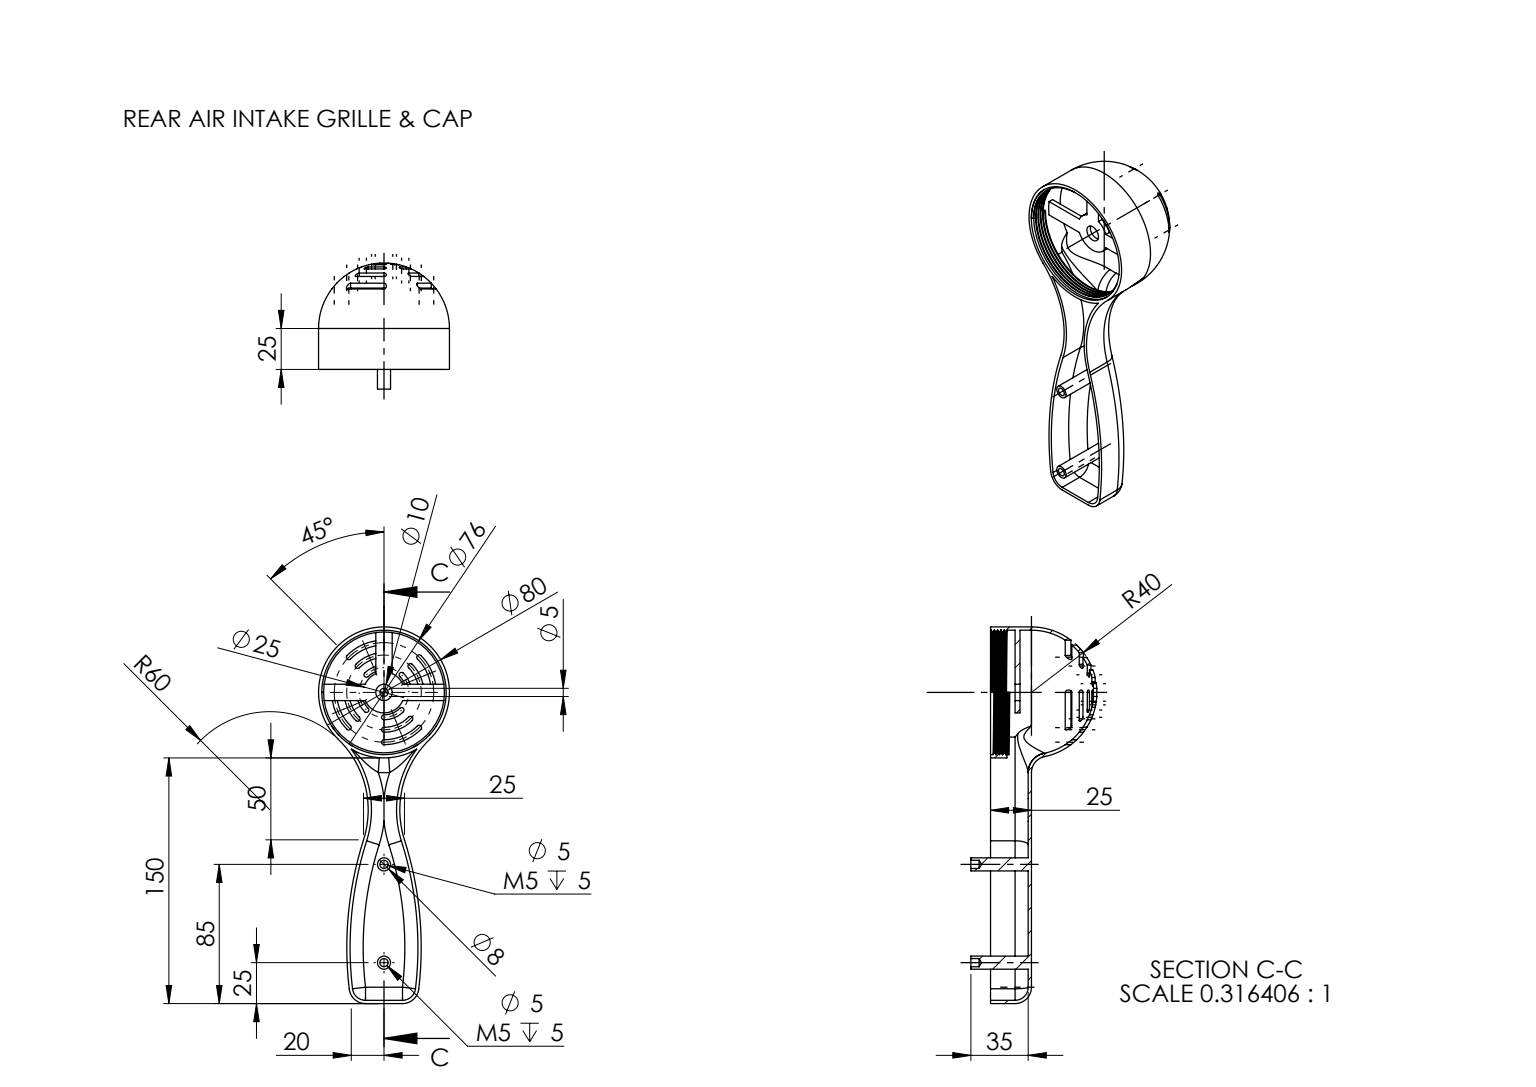
ISO-10303-21;
HEADER;
FILE_DESCRIPTION (('STEP AP214'),
    '1' );
FILE_NAME ('Rear Air Intake Grille & Cap.step',
    '2026-10-04T13:31:42',
    ( '' ),
    ( '' ),
    'SwSTEP 2.0',
    'SolidWorks 2026',
    '' );
FILE_SCHEMA (( 'AUTOMOTIVE_DESIGN' ));
ENDSEC;

DATA;
#20=CARTESIAN_POINT ( 'NONE',  ( 0.000000000000000000, 0.000000000000000000, -45.64921306006598201 ) ) ;
#25=CARTESIAN_POINT ( 'NONE',  ( -3.573655867282028392E-15, 2.428612866367529932E-14, -24.99999999999997868 ) ) ;
#63=ORIENTED_EDGE ( 'NONE', *, *, #98272, .F. ) ;
#65=CIRCLE ( 'NONE', #138924, 4.000000000000000888 ) ;
#97=CARTESIAN_POINT ( 'NONE',  ( 7.656827144875921753, -71.74905178543389184, -15.00000000000000178 ) ) ;
#127=FACE_OUTER_BOUND ( 'NONE', #92552, .T. ) ;
#189=ORIENTED_EDGE ( 'NONE', *, *, #119223, .F. ) ;
#212=SPHERICAL_SURFACE ( 'NONE', #37950, 10.00000000000000000 ) ;
#223=CARTESIAN_POINT ( 'NONE',  ( 15.64208950468054127, -40.81369178264755959, -21.33727593494802122 ) ) ;
#225=CYLINDRICAL_SURFACE ( 'NONE', #105054, 10.00000000000000178 ) ;
#232=CARTESIAN_POINT ( 'NONE',  ( 17.25602135761909395, -17.10936820804715808, -56.77278709839602300 ) ) ;
#243=VERTEX_POINT ( 'NONE', #159375 ) ;
#246=CARTESIAN_POINT ( 'NONE',  ( -30.74264578624800492, -22.33583958711396278, -7.800000000000000711 ) ) ;
#272=CARTESIAN_POINT ( 'NONE',  ( 14.16830335033699662, -40.16376294013230819, -20.11902964094307933 ) ) ;
#277=EDGE_LOOP ( 'NONE', ( #133276, #198078, #94972, #136074, #147190 ) ) ;
#299=CARTESIAN_POINT ( 'NONE',  ( 33.78191506369888941, -21.41920200728860380, -24.99999999999997868 ) ) ;
#420=ORIENTED_EDGE ( 'NONE', *, *, #46651, .T. ) ;
#424=ORIENTED_EDGE ( 'NONE', *, *, #57992, .F. ) ;
#435=CARTESIAN_POINT ( 'NONE',  ( -8.139631411200216604, -37.86970803905148131, -24.01681473740524808 ) ) ;
#457=CARTESIAN_POINT ( 'NONE',  ( 22.90195793322444473, -20.95683088396668481, -46.91699765554876222 ) ) ;
#468=EDGE_CURVE ( 'NONE', #150285, #194492, #147057, .T. ) ;
#495=CARTESIAN_POINT ( 'NONE',  ( 5.136056113497502906, -40.38396894446272967, -25.53196577693411840 ) ) ;
#515=VERTEX_POINT ( 'NONE', #119633 ) ;
#540=DIRECTION ( 'NONE',  ( 1.000000000000000000, 0.000000000000000000, 0.000000000000000000 ) ) ;
#584=AXIS2_PLACEMENT_3D ( 'NONE', #105275, #147807, #196325 ) ;
#611=ORIENTED_EDGE ( 'NONE', *, *, #28066, .F. ) ;
#630=EDGE_CURVE ( 'NONE', #182346, #12418, #12467, .T. ) ;
#707=CARTESIAN_POINT ( 'NONE',  ( -1.429200727443362906, -15.66521691804238436, -59.59145728475412795 ) ) ;
#713=CARTESIAN_POINT ( 'NONE',  ( 0.9827870232946694928, 21.65019873939048267, -58.62068706038626686 ) ) ;
#720=EDGE_LOOP ( 'NONE', ( #54967, #73852, #188508, #135992 ) ) ;
#722=ADVANCED_FACE ( 'NONE', ( #57962 ), #165143, .F. ) ;
#729=CARTESIAN_POINT ( 'NONE',  ( 37.99999999999999289, 2.893978650043524126E-14, -10.74999999453762811 ) ) ;
#742=CARTESIAN_POINT ( 'NONE',  ( 3.915344532211609163, 5.773958127068983259, -62.35465819465156301 ) ) ;
#749=EDGE_CURVE ( 'NONE', #58211, #154964, #98211, .T. ) ;
#778=CARTESIAN_POINT ( 'NONE',  ( -11.40812507854754720, -35.11059874428192273, -8.724999997268813701 ) ) ;
#782=ORIENTED_EDGE ( 'NONE', *, *, #187478, .F. ) ;
#789=CARTESIAN_POINT ( 'NONE',  ( -11.74323870453920549, 9.621741624713935792, -62.00714677346291381 ) ) ;
#803=CARTESIAN_POINT ( 'NONE',  ( -33.52048507002410105, -21.84028095222511823, -24.62089730557312350 ) ) ;
#834=ORIENTED_EDGE ( 'NONE', *, *, #188269, .F. ) ;
#928=CARTESIAN_POINT ( 'NONE',  ( -22.90350128981420141, 22.02608267474392179, -45.83983912514964487 ) ) ;
#930=CARTESIAN_POINT ( 'NONE',  ( 6.685465210013314952, -6.128229644718811819, -61.90241664256964782 ) ) ;
#962=EDGE_LOOP ( 'NONE', ( #189631, #4030 ) ) ;
#966=CARTESIAN_POINT ( 'NONE',  ( -8.724588103088155577, 0.9974278668898441946, -61.97156292062780381 ) ) ;
#981=EDGE_CURVE ( 'NONE', #31363, #49313, #26634, .T. ) ;
#1026=CARTESIAN_POINT ( 'NONE',  ( -10.65638358537376007, -44.90791467878717924, -23.56120423312990297 ) ) ;
#1031=DIRECTION ( 'NONE',  ( 0.000000000000000000, 0.000000000000000000, 1.000000000000000000 ) ) ;
#1065=CARTESIAN_POINT ( 'NONE',  ( -0.4881926659581863892, -9.021779378622676759, -61.91041879129567604 ) ) ;
#1092=CARTESIAN_POINT ( 'NONE',  ( 0.000000000000000000, 0.000000000000000000, -64.92279855667830191 ) ) ;
#1129=DIRECTION ( 'NONE',  ( -0.000000000000000000, 0.000000000000000000, 1.000000000000000000 ) ) ;
#1179=ORIENTED_EDGE ( 'NONE', *, *, #88509, .T. ) ;
#1181=DIRECTION ( 'NONE',  ( -0.000000000000000000, -0.000000000000000000, 1.000000000000000000 ) ) ;
#1190=EDGE_CURVE ( 'NONE', #113441, #194207, #182299, .T. ) ;
#1215=CARTESIAN_POINT ( 'NONE',  ( 26.46959431505284499, -27.26463967846488146, -15.00000000000000178 ) ) ;
#1217=CARTESIAN_POINT ( 'NONE',  ( -1.227931366032057224E-14, -24.30000000000003268, -54.21489346206828230 ) ) ;
#1222=CARTESIAN_POINT ( 'NONE',  ( 17.61359324038537721, -16.30702395557608142, -56.99769869564799052 ) ) ;
#1227=CARTESIAN_POINT ( 'NONE',  ( -17.26089242801066348, 17.10449713765558499, -56.77278709839601589 ) ) ;
#1233=VERTEX_POINT ( 'NONE', #44770 ) ;
#1262=CARTESIAN_POINT ( 'NONE',  ( 17.93416671128860784, -36.08982269496112139, -18.53391066944393728 ) ) ;
#1266=ORIENTED_EDGE ( 'NONE', *, *, #147318, .T. ) ;
#1280=VECTOR ( 'NONE', #85682, 1000.000000000000000 ) ;
#1289=ORIENTED_EDGE ( 'NONE', *, *, #38432, .T. ) ;
#1351=LINE ( 'NONE', #17535, #30677 ) ;
#1378=CARTESIAN_POINT ( 'NONE',  ( -20.01995586163601715, -21.79717389941245287, -51.90954606063881016 ) ) ;
#1419=ORIENTED_EDGE ( 'NONE', *, *, #80402, .F. ) ;
#1430=EDGE_CURVE ( 'NONE', #122419, #49313, #11102, .T. ) ;
#1432=CARTESIAN_POINT ( 'NONE',  ( -17.48462780208382128, -33.70920939566911301, -26.63509803227388062 ) ) ;
#1450=CARTESIAN_POINT ( 'NONE',  ( 17.62203461105333702, -16.12203461105326951, -57.08650645001478097 ) ) ;
#1454=CARTESIAN_POINT ( 'NONE',  ( 22.14710224105762748, -20.13854895287483515, -48.40914604263300447 ) ) ;
#1462=CARTESIAN_POINT ( 'NONE',  ( 6.685389299484707948, -6.128353407782586082, -63.95879637121625194 ) ) ;
#1481=CARTESIAN_POINT ( 'NONE',  ( 11.40812507854754365, 35.11059874428196537, -1.224999997268813479 ) ) ;
#1491=CARTESIAN_POINT ( 'NONE',  ( 21.53686564358446631, -33.52628202222955167, -20.57266355564622629 ) ) ;
#1611=VERTEX_POINT ( 'NONE', #4204 ) ;
#1629=EDGE_CURVE ( 'NONE', #185763, #46465, #128478, .T. ) ;
#1684=AXIS2_PLACEMENT_3D ( 'NONE', #76193, #63008, #124687 ) ;
#1712=CARTESIAN_POINT ( 'NONE',  ( -0.2055526423334300690, -16.68934465457932959, -59.13845350790287370 ) ) ;
#1733=CARTESIAN_POINT ( 'NONE',  ( 3.556970738554033499E-15, -38.81732327939057825, -10.62499999726881050 ) ) ;
#1746=CARTESIAN_POINT ( 'NONE',  ( -193.3062444957834884, -155.7167183371838064, -15.00000000000000178 ) ) ;
#1762=AXIS2_PLACEMENT_3D ( 'NONE', #110360, #81011, #66842 ) ;
#1784=CARTESIAN_POINT ( 'NONE',  ( 22.81625015709509441, 31.40387420917330275, -3.824999997268813345 ) ) ;
#1786=ORIENTED_EDGE ( 'NONE', *, *, #121976, .F. ) ;
#1793=CARTESIAN_POINT ( 'NONE',  ( 17.10305700086941272, -33.88765926517208982, -26.94085628989243730 ) ) ;
#1807=ORIENTED_EDGE ( 'NONE', *, *, #14345, .F. ) ;
#1891=DIRECTION ( 'NONE',  ( 1.000000000000000000, 0.000000000000000000, 0.000000000000000000 ) ) ;
#1893=EDGE_CURVE ( 'NONE', #82035, #127301, #31585, .T. ) ;
#1906=VECTOR ( 'NONE', #11374, 1000.000000000000000 ) ;
#1912=CARTESIAN_POINT ( 'NONE',  ( 1.425040633100159937, 7.121692137566853376, -62.29960613186693763 ) ) ;
#1935=CARTESIAN_POINT ( 'NONE',  ( 1.366360357771132517, 29.77508901761298787, -48.57104573785031221 ) ) ;
#1937=CARTESIAN_POINT ( 'NONE',  ( -24.11542121825890561, 0.7284999611697620114, -54.35861002160294930 ) ) ;
#1974=ADVANCED_FACE ( 'NONE', ( #188258, #93235, #49732, #35552, #138750, #32579, #47755, #94232, #173085, #34564, #96220, #155913, #15422, #140738, #16418, #19399, #154920, #127556 ), #125579, .F. ) ;
#2027=CARTESIAN_POINT ( 'NONE',  ( 1.221313414957698099E-14, -31.90000000000003411, -45.64921306006598201 ) ) ;
#2054=AXIS2_PLACEMENT_3D ( 'NONE', #17433, #106450, #168129 ) ;
#2072=CYLINDRICAL_SURFACE ( 'NONE', #98302, 1.500000000000001332 ) ;
#2145=CIRCLE ( 'NONE', #140835, 61.99999999999998579 ) ;
#2188=CARTESIAN_POINT ( 'NONE',  ( 0.000000000000000000, -165.0000000000000000, 12.00000000000000355 ) ) ;
#2196=VECTOR ( 'NONE', #7013, 1000.000000000000000 ) ;
#2220=CARTESIAN_POINT ( 'NONE',  ( 13.50000934768028671, -42.70547949999480153, -22.37447973961942793 ) ) ;
#2232=DIRECTION ( 'NONE',  ( 0.000000000000000000, 0.000000000000000000, 1.000000000000000000 ) ) ;
#2238=ORIENTED_EDGE ( 'NONE', *, *, #185422, .T. ) ;
#2265=CARTESIAN_POINT ( 'NONE',  ( 9.164641033550608995, -36.31047332450842902, -31.46032839770289513 ) ) ;
#2292=ORIENTED_EDGE ( 'NONE', *, *, #135320, .T. ) ;
#2294=AXIS2_PLACEMENT_3D ( 'NONE', #133017, #26862, #120823 ) ;
#2307=DIRECTION ( 'NONE',  ( 1.000000000000000000, 0.000000000000000000, 0.000000000000000000 ) ) ;
#2350=CARTESIAN_POINT ( 'NONE',  ( -38.00000000000000711, 2.428612866367529932E-14, -3.749999994537626780 ) ) ;
#2366=EDGE_CURVE ( 'NONE', #144904, #188934, #66351, .T. ) ;
#2371=DIRECTION ( 'NONE',  ( 0.000000000000000000, 0.000000000000000000, -1.000000000000000000 ) ) ;
#2380=CARTESIAN_POINT ( 'NONE',  ( 3.766062262543149401E-15, -39.95556452105413570, -7.500000000000000888 ) ) ;
#2382=CARTESIAN_POINT ( 'NONE',  ( -21.29652154493212990, -22.98910344481098988, -49.85957558946837054 ) ) ;
#2401=B_SPLINE_CURVE_WITH_KNOTS ( 'NONE', 3,
 ( #185497, #49966, #125805, #48974, #110629, #172310, #78294, #18640, #139968, #80286, #46988, #31817, #63135, #143950, #37777, #52933, #51944, #193471, #159112, #5430, #7426, #19624, #113604, #189481, #116620, #175298 ),
 .UNSPECIFIED., .F., .F.,
 ( 4, 2, 2, 2, 2, 2, 2, 2, 2, 2, 2, 2, 4 ),
 ( 2.788292423116888737E-07, 0.0002961032055655192312, 0.0005919275818887267775, 0.0008877519582119342695, 0.001183576334535141545, 0.001775225087181556095, 0.002366873839827970862, 0.002662698216151183558, 0.002958522592474396255, 0.003254346968797609384, 0.003550171345120822081, 0.004141820097767247473, 0.004733468850413673733 ),
 .UNSPECIFIED. ) ;
#2417=ORIENTED_EDGE ( 'NONE', *, *, #165213, .F. ) ;
#2423=DIRECTION ( 'NONE',  ( -9.445700745138859830E-17, 1.000000000000000000, 0.000000000000000000 ) ) ;
#2456=CARTESIAN_POINT ( 'NONE',  ( 21.60633875066715959, -19.99157099255409165, -49.03222299240194815 ) ) ;
#2462=DIRECTION ( 'NONE',  ( 0.000000000000000000, 0.000000000000000000, 1.000000000000000000 ) ) ;
#2474=AXIS2_PLACEMENT_3D ( 'NONE', #196952, #104924, #28113 ) ;
#2483=CARTESIAN_POINT ( 'NONE',  ( 22.81625015709510151, -31.40387420917324590, -3.924999997268811658 ) ) ;
#2493=CARTESIAN_POINT ( 'NONE',  ( 24.80109738229595351, -30.87060611836716717, -19.02242571536587334 ) ) ;
#2512=ORIENTED_EDGE ( 'NONE', *, *, #55964, .F. ) ;
#2540=CARTESIAN_POINT ( 'NONE',  ( -16.15948758285046338, -17.62941224709156529, -54.53140136687973438 ) ) ;
#2544=CARTESIAN_POINT ( 'NONE',  ( 11.40812507854755253, -35.11059874428192273, -8.524999997268814411 ) ) ;
#2545=CARTESIAN_POINT ( 'NONE',  ( 23.48529157249599564, 32.32473071737754111, -2.449999994537626513 ) ) ;
#2552=FACE_OUTER_BOUND ( 'NONE', #116365, .T. ) ;
#2590=ADVANCED_FACE ( 'NONE', ( #83038 ), #179085, .F. ) ;
#2607=CIRCLE ( 'NONE', #18786, 216.0437394197456911 ) ;
#2693=B_SPLINE_CURVE_WITH_KNOTS ( 'NONE', 3,
 ( #139494, #65640, #46503, #108163, #142482, #141494, #49487, #63665, #200187, #111149, #153678, #172839, #140497, #186027, #169845, #45512, #110160, #34318, #80804, #77825, #32336, #15175, #48506, #3960 ),
 .UNSPECIFIED., .F., .F.,
 ( 4, 2, 2, 2, 2, 2, 2, 2, 2, 2, 2, 4 ),
 ( 1.968491852713559257E-07, 0.0003260565056757782384, 0.0006519161621662850634, 0.0009777758186567920510, 0.001303635475147298930, 0.001955354788128312472, 0.002607074101109326230, 0.003258793414090339988, 0.003910512727071354180, 0.004562232040052368806, 0.004888091696542873517, 0.005213951353033378228 ),
 .UNSPECIFIED. ) ;
#2723=EDGE_LOOP ( 'NONE', ( #5934, #77789, #146194, #159845 ) ) ;
#2730=CARTESIAN_POINT ( 'NONE',  ( -22.81625015709509441, -31.40387420917324590, -10.82499999726881157 ) ) ;
#2742=CARTESIAN_POINT ( 'NONE',  ( 4.381595247748339084, 6.502951376627817304, -62.18229462841636490 ) ) ;
#2746=EDGE_CURVE ( 'NONE', #167830, #92192, #92435, .T. ) ;
#2777=DIRECTION ( 'NONE',  ( 0.000000000000000000, 0.000000000000000000, 1.000000000000000000 ) ) ;
#2780=CARTESIAN_POINT ( 'NONE',  ( 22.81625015709510151, -31.40387420917324590, -2.424999997268812546 ) ) ;
#2803=ORIENTED_EDGE ( 'NONE', *, *, #179291, .F. ) ;
#2889=CARTESIAN_POINT ( 'NONE',  ( -1.040834085586084257E-14, 30.40000000000003766, -65.00100000000003320 ) ) ;
#2927=DIRECTION ( 'NONE',  ( 0.000000000000000000, 0.000000000000000000, 1.000000000000000000 ) ) ;
#2931=CARTESIAN_POINT ( 'NONE',  ( -1.304248841091933035E-15, -21.30000000000002913, -64.92279855667830191 ) ) ;
#2947=CARTESIAN_POINT ( 'NONE',  ( -3.874011537017814977, -5.276842784226742467, -62.43202641272173992 ) ) ;
#2962=ORIENTED_EDGE ( 'NONE', *, *, #57363, .F. ) ;
#2966=DIRECTION ( 'NONE',  ( -0.000000000000000000, -0.000000000000000000, -1.000000000000000000 ) ) ;
#2980=CARTESIAN_POINT ( 'NONE',  ( -1.029908246020144968, -31.49504140153652898, -49.63772645510944415 ) ) ;
#3037=CARTESIAN_POINT ( 'NONE',  ( 0.000000000000000000, 0.000000000000000000, -18.00000000000000000 ) ) ;
#3054=DIRECTION ( 'NONE',  ( -0.000000000000000000, -0.000000000000000000, 1.000000000000000000 ) ) ;
#3068=CARTESIAN_POINT ( 'NONE',  ( -13.70000000000001528, 0.2066332630088025535, -62.58071313852362039 ) ) ;
#3092=CARTESIAN_POINT ( 'NONE',  ( -10.46900522708356895, -36.04764466666199496, -30.96889465344750292 ) ) ;
#3107=AXIS2_PLACEMENT_3D ( 'NONE', #176431, #145067, #162243 ) ;
#3134=DIRECTION ( 'NONE',  ( 1.000000000000000000, 0.000000000000000000, 0.000000000000000000 ) ) ;
#3195=CARTESIAN_POINT ( 'NONE',  ( 15.29519331188521747, -1.499966876285990347, -61.92990168432670828 ) ) ;
#3228=CARTESIAN_POINT ( 'NONE',  ( -15.50344475828858748, 14.75151636811253120, -58.79419791951499974 ) ) ;
#3262=CARTESIAN_POINT ( 'NONE',  ( 24.50241233882493219, -28.74340065771663433, -20.80149134687501089 ) ) ;
#3267=ORIENTED_EDGE ( 'NONE', *, *, #14918, .T. ) ;
#3288=DIRECTION ( 'NONE',  ( 1.000000000000000000, 0.000000000000000000, 0.000000000000000000 ) ) ;
#3289=ORIENTED_EDGE ( 'NONE', *, *, #133011, .T. ) ;
#3323=DIRECTION ( 'NONE',  ( -0.000000000000000000, -0.000000000000000000, -1.000000000000000000 ) ) ;
#3328=CARTESIAN_POINT ( 'NONE',  ( 8.348819774032595120, -1.314123079931750926, -62.04874212273342948 ) ) ;
#3344=CARTESIAN_POINT ( 'NONE',  ( -4.071997446883320215, -4.622768748654204174, -62.49744614497421935 ) ) ;
#3371=CARTESIAN_POINT ( 'NONE',  ( 9.456233179636212682, 11.51622829137495074, -59.95663916823115613 ) ) ;
#3411=ORIENTED_EDGE ( 'NONE', *, *, #139086, .F. ) ;
#3412=PLANE ( 'NONE',  #166342 ) ;
#3422=CARTESIAN_POINT ( 'NONE',  ( -25.83444802367754178, -27.47999234037504834, -20.36589038153027076 ) ) ;
#3444=CARTESIAN_POINT ( 'NONE',  ( -22.55670631985092456, 22.55670631985084995, -45.64921306006598201 ) ) ;
#3450=CARTESIAN_POINT ( 'NONE',  ( 2.500000000000000000, -165.0000000000000000, 7.000000000000003553 ) ) ;
#3467=ORIENTED_EDGE ( 'NONE', *, *, #68507, .F. ) ;
#3469=CARTESIAN_POINT ( 'NONE',  ( -22.81625015709510507, 31.40387420917330275, -4.924999997268813878 ) ) ;
#3479=CARTESIAN_POINT ( 'NONE',  ( 22.60381889853746173, -32.71308136366295827, -20.00853410804237242 ) ) ;
#3531=CARTESIAN_POINT ( 'NONE',  ( 11.40812507854754365, 35.11059874428196537, -3.224999997268813701 ) ) ;
#3564=CARTESIAN_POINT ( 'NONE',  ( 29.61737564226525876, -1.282731051913165388, -51.85482277101435500 ) ) ;
#3595=EDGE_LOOP ( 'NONE', ( #36208, #123149, #70849, #193266 ) ) ;
#3690=CARTESIAN_POINT ( 'NONE',  ( 1.342408831710876438, 22.10627130652513017, -55.87976878746020759 ) ) ;
#3708=ORIENTED_EDGE ( 'NONE', *, *, #21762, .T. ) ;
#3711=B_SPLINE_CURVE_WITH_KNOTS ( 'NONE', 3,
 ( #6941, #68620, #140734, #100949, #49728, #176825, #162633, #187273 ),
 .UNSPECIFIED., .F., .F.,
 ( 4, 2, 2, 4 ),
 ( 0.005020700917424133526, 0.005703339821162721132, 0.006044659273032013634, 0.006385978724901306136 ),
 .UNSPECIFIED. ) ;
#3715=CARTESIAN_POINT ( 'NONE',  ( 36.91746824999999887, 11.99521256947799053, -8.024999997268814411 ) ) ;
#3749=CARTESIAN_POINT ( 'NONE',  ( 0.000000000000000000, 0.000000000000000000, -18.00000000000000000 ) ) ;
#3755=VERTEX_POINT ( 'NONE', #40545 ) ;
#3759=DIRECTION ( 'NONE',  ( -1.000000000000000000, 1.246178594180516623E-14, 0.000000000000000000 ) ) ;
#3762=CARTESIAN_POINT ( 'NONE',  ( -36.91746825000000598, 2.428612866367529932E-14, -3.124999997268813168 ) ) ;
#3763=CARTESIAN_POINT ( 'NONE',  ( -21.85243030949941456, 20.02676387111000622, -51.86007293692900078 ) ) ;
#3776=PRODUCT_CONTEXT ( 'NONE', #173204, 'mechanical' ) ;
#3786=ORIENTED_EDGE ( 'NONE', *, *, #177460, .F. ) ;
#3931=CARTESIAN_POINT ( 'NONE',  ( 16.53812085701073187, -14.65432885500447746, -55.91693222716156697 ) ) ;
#3940=EDGE_CURVE ( 'NONE', #118127, #27924, #43421, .T. ) ;
#3948=DIRECTION ( 'NONE',  ( -1.000000000000000000, 0.000000000000000000, 0.000000000000000000 ) ) ;
#3960=CARTESIAN_POINT ( 'NONE',  ( 21.30000000000002913, -7.567280135845077329E-14, -58.85720012050612837 ) ) ;
#3962=CARTESIAN_POINT ( 'NONE',  ( 27.48145228890733094, -25.86941904439665052, -20.55877432051690690 ) ) ;
#3996=B_SPLINE_CURVE_WITH_KNOTS ( 'NONE', 3,
 ( #16571, #139889, #1378, #171245, #14584, #32734, #94386, #156065, #183444, #17563, #76241, #2382, #106584, #137919, #168261, #199603, #29757, #91392 ),
 .UNSPECIFIED., .F., .F.,
 ( 4, 2, 2, 2, 2, 2, 2, 2, 4 ),
 ( 0.001292559216902551241, 0.001886468742252372498, 0.002480378267602193973, 0.003074287792952015014, 0.003668197318301836922, 0.004262106843651657963, 0.004856016369001479004, 0.005449925894351300912, 0.006043835419701121953 ),
 .UNSPECIFIED. ) ;
#3999=CARTESIAN_POINT ( 'NONE',  ( 0.000000000000000000, -105.0000000000000000, 7.000000000000003553 ) ) ;
#4017=CARTESIAN_POINT ( 'NONE',  ( -2.802625768539468432, -39.09149893265184517, -33.00000000000000000 ) ) ;
#4030=ORIENTED_EDGE ( 'NONE', *, *, #121810, .F. ) ;
#4084=FACE_OUTER_BOUND ( 'NONE', #127362, .T. ) ;
#4108=DIRECTION ( 'NONE',  ( -1.000000000000000000, 0.000000000000000000, 0.000000000000000000 ) ) ;
#4111=CARTESIAN_POINT ( 'NONE',  ( 13.70000000000001528, -4.867217739956692332E-14, -64.92279855667830191 ) ) ;
#4160=ORIENTED_EDGE ( 'NONE', *, *, #91683, .T. ) ;
#4166=DIRECTION ( 'NONE',  ( -0.000000000000000000, -0.000000000000000000, -1.000000000000000000 ) ) ;
#4204=CARTESIAN_POINT ( 'NONE',  ( 1.221313414957698099E-14, -31.90000000000003411, -45.64921306006598201 ) ) ;
#4209=CARTESIAN_POINT ( 'NONE',  ( -15.29496450215403058, 1.499960427298884680, -59.75377357153833913 ) ) ;
#4217=AXIS2_PLACEMENT_3D ( 'NONE', #86911, #8069, #40413 ) ;
#4228=ORIENTED_EDGE ( 'NONE', *, *, #72173, .F. ) ;
#4269=VERTEX_POINT ( 'NONE', #96770 ) ;
#4303=CYLINDRICAL_SURFACE ( 'NONE', #49564, 38.00000000000000000 ) ;
#4318=CARTESIAN_POINT ( 'NONE',  ( -9.141470119588765426E-16, -69.45486021086043138, -22.99263613531268291 ) ) ;
#4351=CARTESIAN_POINT ( 'NONE',  ( 37.99999999999999289, 2.893978650043524126E-14, -7.000000000000000000 ) ) ;
#4389=EDGE_CURVE ( 'NONE', #70174, #115376, #63320, .T. ) ;
#4404=CARTESIAN_POINT ( 'NONE',  ( -37.02045864137325992, -17.72559658019849138, -19.07609595512615996 ) ) ;
#4420=CIRCLE ( 'NONE', #36755, 16.70000000000002061 ) ;
#4421=DIRECTION ( 'NONE',  ( 1.000000000000000000, 0.000000000000000000, 0.000000000000000000 ) ) ;
#4426=CARTESIAN_POINT ( 'NONE',  ( -31.77050690183224546, 0.6194686979414664174, -45.83912112027729080 ) ) ;
#4448=CARTESIAN_POINT ( 'NONE',  ( 36.91746825000000598, -11.99521256947793546, -1.724999997268813479 ) ) ;
#4459=CARTESIAN_POINT ( 'NONE',  ( 13.37225149056123108, -38.04021455641917271, -24.47500528307575252 ) ) ;
#4485=CARTESIAN_POINT ( 'NONE',  ( 0.000000000000000000, 0.000000000000000000, -64.92279855667830191 ) ) ;
#4506=CARTESIAN_POINT ( 'NONE',  ( -16.00800591765002778, -17.62450045179643254, -54.61670405711556242 ) ) ;
#4510=CARTESIAN_POINT ( 'NONE',  ( 3.556970738554033499E-15, -38.81732327939057825, -8.624999997268814056 ) ) ;
#4526=AXIS2_PLACEMENT_3D ( 'NONE', #70715, #118222, #178904 ) ;
#4530=DIRECTION ( 'NONE',  ( 0.000000000000000000, 0.000000000000000000, -1.000000000000000000 ) ) ;
#4544=CARTESIAN_POINT ( 'NONE',  ( 12.21143611141174468, -11.13220115481712646, -61.42794421580953212 ) ) ;
#4547=AXIS2_PLACEMENT_3D ( 'NONE', #182810, #104965, #93502 ) ;
#4595=CIRCLE ( 'NONE', #146625, 24.30000000000003268 ) ;
#4618=VECTOR ( 'NONE', #144945, 1000.000000000000000 ) ;
#4644=VERTEX_POINT ( 'NONE', #59254 ) ;
#4670=VECTOR ( 'NONE', #189946, 1000.000000000000000 ) ;
#4698=CARTESIAN_POINT ( 'NONE',  ( -36.91746825000001309, -11.99521256947794789, -7.024999997268812635 ) ) ;
#4747=CARTESIAN_POINT ( 'NONE',  ( 36.91746825000000598, -11.99521256947793546, -2.224999997268813701 ) ) ;
#4748=CARTESIAN_POINT ( 'NONE',  ( -20.61667489342692150, 20.25409705915558689, -52.65483682830181777 ) ) ;
#4763=ORIENTED_EDGE ( 'NONE', *, *, #39724, .F. ) ;
#4818=ORIENTED_EDGE ( 'NONE', *, *, #137018, .F. ) ;
#4841=CARTESIAN_POINT ( 'NONE',  ( 0.000000000000000000, 0.000000000000000000, -56.77278709839600879 ) ) ;
#4843=DIRECTION ( 'NONE',  ( -0.000000000000000000, -0.000000000000000000, 1.000000000000000000 ) ) ;
#4868=EDGE_CURVE ( 'NONE', #192734, #168486, #104777, .T. ) ;
#4898=DIRECTION ( 'NONE',  ( -0.000000000000000000, 0.000000000000000000, 1.000000000000000000 ) ) ;
#4920=CARTESIAN_POINT ( 'NONE',  ( -30.26186088262143059, 1.502453648625585281, -51.11561252063849281 ) ) ;
#4937=CARTESIAN_POINT ( 'NONE',  ( 37.99999999999999289, 2.893978650043524126E-14, -2.749999994537626780 ) ) ;
#4947=DIRECTION ( 'NONE',  ( 0.000000000000000000, 0.000000000000000000, 1.000000000000000000 ) ) ;
#4965=AXIS2_PLACEMENT_3D ( 'NONE', #90039, #28400, #135568 ) ;
#4995=CARTESIAN_POINT ( 'NONE',  ( -1.278449583442071713, -31.20457203169705096, -46.64972497815391250 ) ) ;
#4999=AXIS2_PLACEMENT_3D ( 'NONE', #194247, #161891, #192238 ) ;
#5009=CARTESIAN_POINT ( 'NONE',  ( -9.646990561631263006, -38.22155086790370149, -31.80034568179328858 ) ) ;
#5010=VERTEX_POINT ( 'NONE', #89630 ) ;
#5042=CARTESIAN_POINT ( 'NONE',  ( -1.351304681146049624, -6.941592873960400922, -62.33628431810817716 ) ) ;
#5055=TOROIDAL_SURFACE ( 'NONE', #179484, 206.0437394197456342, 10.00000000000000000 ) ;
#5062=CARTESIAN_POINT ( 'NONE',  ( -2.500000000000000000, -165.0000000000000000, 7.000000000000003553 ) ) ;
#5079=ADVANCED_FACE ( 'NONE', ( #148320 ), #71476, .T. ) ;
#5138=DIRECTION ( 'NONE',  ( -1.000000000000000000, 0.000000000000000000, 0.000000000000000000 ) ) ;
#5177=ORIENTED_EDGE ( 'NONE', *, *, #34776, .T. ) ;
#5204=CARTESIAN_POINT ( 'NONE',  ( 0.000000000000000000, 0.000000000000000000, -45.64921306006598201 ) ) ;
#5211=ORIENTED_EDGE ( 'NONE', *, *, #139086, .T. ) ;
#5234=LINE ( 'NONE', #97233, #43292 ) ;
#5301=DIRECTION ( 'NONE',  ( -0.000000000000000000, 0.000000000000000000, 1.000000000000000000 ) ) ;
#5350=CARTESIAN_POINT ( 'NONE',  ( -11.74264578624799782, -36.14014761921581709, -7.599999999999999645 ) ) ;
#5390=ORIENTED_EDGE ( 'NONE', *, *, #176309, .T. ) ;
#5394=ORIENTED_EDGE ( 'NONE', *, *, #47533, .T. ) ;
#5404=CARTESIAN_POINT ( 'NONE',  ( -27.37900830011268027, -26.18142635053349210, -16.57177559434630609 ) ) ;
#5408=EDGE_CURVE ( 'NONE', #57684, #116458, #31935, .T. ) ;
#5420=ORIENTED_EDGE ( 'NONE', *, *, #58231, .F. ) ;
#5422=DIRECTION ( 'NONE',  ( 0.000000000000000000, 0.000000000000000000, 1.000000000000000000 ) ) ;
#5430=CARTESIAN_POINT ( 'NONE',  ( 5.170161995863685966, 6.863278975470355370, -64.06628402976478753 ) ) ;
#5431=CARTESIAN_POINT ( 'NONE',  ( -9.656827144875922642, -71.74905178543390605, -25.00000000000000000 ) ) ;
#5454=CARTESIAN_POINT ( 'NONE',  ( -36.91746825000001309, -11.99521256947794789, -4.524999997268813523 ) ) ;
#5465=CARTESIAN_POINT ( 'NONE',  ( 18.40487137061644418, -35.48337831122941566, -26.72115582345234941 ) ) ;
#5499=AXIS2_PLACEMENT_3D ( 'NONE', #65195, #36836, #37853 ) ;
#5508=EDGE_CURVE ( 'NONE', #66459, #145335, #32930, .T. ) ;
#5516=CARTESIAN_POINT ( 'NONE',  ( 36.91746825000000598, -11.99521256947793546, -10.22499999726881548 ) ) ;
#5551=CARTESIAN_POINT ( 'NONE',  ( 23.48529157249600630, -32.32473071737748427, -1.299999999999999822 ) ) ;
#5609=EDGE_CURVE ( 'NONE', #62967, #140310, #11253, .T. ) ;
#5635=CARTESIAN_POINT ( 'NONE',  ( 0.000000000000000000, 0.000000000000000000, -59.13370768023891344 ) ) ;
#5662=LINE ( 'NONE', #189711, #146711 ) ;
#5674=DIRECTION ( 'NONE',  ( -0.000000000000000000, -0.000000000000000000, -1.000000000000000000 ) ) ;
#5679=DIRECTION ( 'NONE',  ( -0.000000000000000000, -0.000000000000000000, 1.000000000000000000 ) ) ;
#5689=CARTESIAN_POINT ( 'NONE',  ( 1.577468763857913883E-14, -78.62686331009493301, -24.99999901254159695 ) ) ;
#5691=CARTESIAN_POINT ( 'NONE',  ( 0.000000000000000000, 0.000000000000000000, -61.34707691135562868 ) ) ;
#5698=ORIENTED_EDGE ( 'NONE', *, *, #139940, .F. ) ;
#5704=CARTESIAN_POINT ( 'NONE',  ( -29.86685920354755552, 21.69954338932564397, -9.324999997268813345 ) ) ;
#5750=CARTESIAN_POINT ( 'NONE',  ( 31.90000000000003411, -9.916512055951908821E-14, -45.64921306006598201 ) ) ;
#5753=CARTESIAN_POINT ( 'NONE',  ( 22.81625015709509441, 31.40387420917330275, -1.824999997268813567 ) ) ;
#5764=AXIS2_PLACEMENT_3D ( 'NONE', #10969, #196003, #74627 ) ;
#5777=EDGE_CURVE ( 'NONE', #113441, #35858, #44000, .T. ) ;
#5778=EDGE_LOOP ( 'NONE', ( #158950, #3267, #104526 ) ) ;
#5788=EDGE_CURVE ( 'NONE', #135024, #43345, #75504, .T. ) ;
#5863=FACE_OUTER_BOUND ( 'NONE', #105488, .T. ) ;
#5880=DIRECTION ( 'NONE',  ( -0.000000000000000000, 0.000000000000000000, 1.000000000000000000 ) ) ;
#5899=CARTESIAN_POINT ( 'NONE',  ( -7.980598154334920480, -36.52039581308733318, -31.83703727319203125 ) ) ;
#5905=CARTESIAN_POINT ( 'NONE',  ( -0.1032682159774158670, -16.70000000000002061, -61.34707691135562868 ) ) ;
#5921=CARTESIAN_POINT ( 'NONE',  ( 15.32289026290833611, -14.84183971327400542, -56.44770181572976497 ) ) ;
#5934=ORIENTED_EDGE ( 'NONE', *, *, #160165, .T. ) ;
#5953=CARTESIAN_POINT ( 'NONE',  ( 39.99999999999999289, 2.428612866367529932E-14, -25.00000000000000000 ) ) ;
#5975=CARTESIAN_POINT ( 'NONE',  ( -11.30153831258470731, -180.0000000000000568, -15.00000000000000178 ) ) ;
#5992=ORIENTED_EDGE ( 'NONE', *, *, #183981, .T. ) ;
#5997=CARTESIAN_POINT ( 'NONE',  ( -1.135674102528219320, -29.41559601785655076, -49.03020479230151807 ) ) ;
#6009=CARTESIAN_POINT ( 'NONE',  ( -2.919401842228618094, -40.72031138817900597, -24.99999999999999289 ) ) ;
#6010=ADVANCED_FACE ( 'NONE', ( #112734 ), #110751, .T. ) ;
#6041=B_SPLINE_CURVE_WITH_KNOTS ( 'NONE', 3,
 ( #29383, #75859, #10232, #40563, #148744, #71892, #133563, #106031, #72734, #73732, #199044, #198056, #181899, #151560, #137365, #58543, #153527, #165735, #89877, #167717, #11058, #118235, #42392, #44375, #60514, #57563 ),
 .UNSPECIFIED., .F., .F.,
 ( 4, 2, 2, 2, 2, 2, 2, 2, 2, 2, 2, 2, 4 ),
 ( 1.971416325814069830E-07, 0.0002960211146592699161, 0.0005918450876859584521, 0.0008876690607126472591, 0.001183493033739336066, 0.001775140979792709343, 0.002366788925846082838, 0.002662612898872765248, 0.002958436871899448525, 0.003254260844926130936, 0.003550084817952813779, 0.004141732764006179034, 0.004733380710059543854 ),
 .UNSPECIFIED. ) ;
#6068=CARTESIAN_POINT ( 'NONE',  ( -14.61778469963293325, -34.91027835867548390, -28.77367925216612576 ) ) ;
#6077=CARTESIAN_POINT ( 'NONE',  ( -3.874011537017815865, -5.668178584001447362, -62.37582247038324823 ) ) ;
#6118=ORIENTED_EDGE ( 'NONE', *, *, #178686, .F. ) ;
#6145=EDGE_CURVE ( 'NONE', #27850, #11421, #169810, .T. ) ;
#6159=ORIENTED_EDGE ( 'NONE', *, *, #78263, .T. ) ;
#6171=CARTESIAN_POINT ( 'NONE',  ( -6.856101608890801443E-16, -71.74905178543389184, -22.99263613531268291 ) ) ;
#6179=VERTEX_POINT ( 'NONE', #111749 ) ;
#6188=CARTESIAN_POINT ( 'NONE',  ( 0.000000000000000000, 0.000000000000000000, -23.00000000000000355 ) ) ;
#6197=( BOUNDED_CURVE ( )  B_SPLINE_CURVE ( 2, ( #81814, #143502, #159671, #66672, #82823, #72681, #162677, #54502, #119183, #149510, #27182, #150522, #133337, #116174, #57515, #146496, #11007, #120160, #7987, #177864, #55501, #102008, #180868, #134356, #40333, #39333, #181851, #178866, #195028, #41342, #103004, #117171, #166685, #164689, #100992, #163690, #86834, #148520, #10010, #135355, #131337, #147523, #25192, #165684, #71670, #26184, #193025, #24183, #43330, #9011, #132345, #85833, #12021, #69670, #56505, #196040, #70679, #118183, #194037, #88829, #179874, #42344, #87824, #104006, #73683, #197027, #58494, #104998, #84817, #137318, #89829, #15971, #168643, #108964, #60466, #59476, #778, #183829, #151510, #182843, #78616, #44326, #31142, #167669, #75640, #62449, #140291, #121150, #13973, #105985, #29167, #13002, #124123, #30142, #46303, #198999, #77631, #185822, #123132, #74665, #32133 ),
 .UNSPECIFIED., .F., .F. ) 
 B_SPLINE_CURVE_WITH_KNOTS ( ( 3, 2, 2, 2, 2, 2, 2, 2, 2, 2, 2, 2, 2, 2, 2, 2, 2, 2, 2, 2, 2, 2, 2, 2, 2, 2, 2, 2, 2, 2, 2, 2, 2, 2, 2, 2, 2, 2, 2, 2, 2, 2, 2, 2, 2, 2, 2, 2, 2, 2, 3 ),
 ( 0.000000000000000000, 0.02000000000000000042, 0.04000000000000000083, 0.05999999999999999778, 0.08000000000000000167, 0.1000000000000000056, 0.1199999999999999956, 0.1400000000000000133, 0.1600000000000000033, 0.1799999999999999933, 0.2000000000000000111, 0.2200000000000000011, 0.2399999999999999911, 0.2600000000000000089, 0.2800000000000000266, 0.2999999999999999889, 0.3200000000000000067, 0.3400000000000000244, 0.3599999999999999867, 0.3800000000000000044, 0.4000000000000000222, 0.4199999999999999845, 0.4400000000000000022, 0.4600000000000000200, 0.4799999999999999822, 0.5000000000000000000, 0.5200000000000000178, 0.5400000000000000355, 0.5600000000000000533, 0.5799999999999999600, 0.5999999999999999778, 0.6199999999999999956, 0.6400000000000000133, 0.6600000000000000311, 0.6800000000000000488, 0.6999999999999999556, 0.7199999999999999734, 0.7399999999999999911, 0.7600000000000000089, 0.7800000000000000266, 0.8000000000000000444, 0.8199999999999999512, 0.8399999999999999689, 0.8599999999999999867, 0.8800000000000000044, 0.9000000000000000222, 0.9200000000000000400, 0.9399999999999999467, 0.9599999999999999645, 0.9799999999999999822, 1.000000000000000000 ),
 .UNSPECIFIED. ) 
 CURVE ( )  GEOMETRIC_REPRESENTATION_ITEM ( )  RATIONAL_B_SPLINE_CURVE ( ( 1.000000000000000000, 0.9510565162951535312, 1.000000000000000000, 0.9510565162951535312, 1.000000000000000000, 0.9510565162951535312, 1.000000000000000000, 0.9510565162951535312, 1.000000000000000000, 0.9510565162951535312, 1.000000000000000000, 0.9510565162951535312, 1.000000000000000000, 0.9510565162951535312, 1.000000000000000000, 0.9510565162951535312, 1.000000000000000000, 0.9510565162951535312, 1.000000000000000000, 0.9510565162951535312, 1.000000000000000000, 0.9510565162951535312, 1.000000000000000000, 0.9510565162951535312, 1.000000000000000000, 0.9510565162951535312, 1.000000000000000000, 0.9510565162951535312, 1.000000000000000000, 0.9510565162951535312, 1.000000000000000000, 0.9510565162951535312, 1.000000000000000000, 0.9510565162951535312, 1.000000000000000000, 0.9510565162951535312, 1.000000000000000000, 0.9510565162951535312, 1.000000000000000000, 0.9510565162951535312, 1.000000000000000000, 0.9510565162951535312, 1.000000000000000000, 0.9510565162951535312, 1.000000000000000000, 0.9510565162951535312, 1.000000000000000000, 0.9510565162951535312, 1.000000000000000000, 0.9510565162951535312, 1.000000000000000000, 0.9510565162951535312, 1.000000000000000000, 0.9510565162951535312, 1.000000000000000000, 0.9510565162951535312, 1.000000000000000000, 0.9510565162951535312, 1.000000000000000000, 0.9510565162951535312, 1.000000000000000000, 0.9510565162951535312, 1.000000000000000000, 0.9510565162951535312, 1.000000000000000000, 0.9510565162951535312, 1.000000000000000000, 0.9510565162951535312, 1.000000000000000000, 0.9510565162951535312, 1.000000000000000000, 0.9510565162951535312, 1.000000000000000000, 0.9510565162951535312, 1.000000000000000000, 0.9510565162951535312, 1.000000000000000000, 0.9510565162951535312, 1.000000000000000000, 0.9510565162951535312, 1.000000000000000000, 0.9510565162951535312, 1.000000000000000000, 0.9510565162951535312, 1.000000000000000000, 0.9510565162951535312, 1.000000000000000000, 0.9510565162951535312, 1.000000000000000000, 0.9510565162951535312, 1.000000000000000000, 0.9510565162951535312, 1.000000000000000000, 0.9510565162951535312, 1.000000000000000000, 0.9510565162951535312, 1.000000000000000000, 0.9510565162951535312, 1.000000000000000000, 0.9510565162951535312, 1.000000000000000000 ) ) 
 REPRESENTATION_ITEM ( '' )  );
#6199=CARTESIAN_POINT ( 'NONE',  ( -38.00000000000000711, 2.428612866367529932E-14, -5.749999994537626336 ) ) ;
#6236=SURFACE_SIDE_STYLE ('',( #127591 ) ) ;
#6240=CARTESIAN_POINT ( 'NONE',  ( 24.94736998983877285, -28.55544918295356638, -16.60430580961556402 ) ) ;
#6263=LINE ( 'NONE', #191292, #46725 ) ;
#6300=AXIS2_PLACEMENT_3D ( 'NONE', #67822, #132498, #161831 ) ;
#6350=CARTESIAN_POINT ( 'NONE',  ( -20.03497210076587010, -21.14457701270107037, -52.41383543719814497 ) ) ;
#6393=CARTESIAN_POINT ( 'NONE',  ( 11.74264578624800315, -36.14014761921581709, -3.400000000000000355 ) ) ;
#6401=CARTESIAN_POINT ( 'NONE',  ( -25.53334702086137042, -27.44079366658189301, -18.45201707417109915 ) ) ;
#6413=FACE_OUTER_BOUND ( 'NONE', #20333, .T. ) ;
#6416=ORIENTED_EDGE ( 'NONE', *, *, #152623, .F. ) ;
#6448=CARTESIAN_POINT ( 'NONE',  ( 11.74264578624800315, -36.14014761921581709, -1.399999999999999689 ) ) ;
#6474=FACE_BOUND ( 'NONE', #962, .T. ) ;
#6485=DIRECTION ( 'NONE',  ( 0.9526137857479310966, -0.3041824702427718408, 0.000000000000000000 ) ) ;
#6510=B_SPLINE_CURVE_WITH_KNOTS ( 'NONE', 3,
 ( #75257, #90421, #186434, #122741, #47910, #64061, #15578, #169243, #45912, #152106, #140893, #198616, #13590, #184432, #154084, #44928, #109564, #77236, #182457, #46911 ),
 .UNSPECIFIED., .F., .F.,
 ( 4, 2, 2, 2, 2, 2, 2, 2, 2, 4 ),
 ( 2.784207231387392883E-07, 0.0003311547508960732472, 0.0006620310810690078346, 0.0009929074112419423136, 0.001323783741414876793, 0.002647289062106605601, 0.003309041722452476294, 0.003970794382798350022, 0.004632547043144224184, 0.005294299703490098347 ),
 .UNSPECIFIED. ) ;
#6511=CARTESIAN_POINT ( 'NONE',  ( 36.91746825000000598, -11.99521256947793546, -8.224999997268810148 ) ) ;
#6515=DIRECTION ( 'NONE',  ( -1.000000000000000000, 0.000000000000000000, 0.000000000000000000 ) ) ;
#6519=FACE_OUTER_BOUND ( 'NONE', #134586, .T. ) ;
#6577=ORIENTED_EDGE ( 'NONE', *, *, #25423, .F. ) ;
#6631=DIRECTION ( 'NONE',  ( 0.000000000000000000, 0.000000000000000000, -1.000000000000000000 ) ) ;
#6641=EDGE_CURVE ( 'NONE', #36560, #198744, #104764, .T. ) ;
#6673=CARTESIAN_POINT ( 'NONE',  ( -28.45933917494770427, -27.69424206401140864, -20.18904788101069769 ) ) ;
#6683=DIRECTION ( 'NONE',  ( 1.000000000000000000, 0.000000000000000000, 0.000000000000000000 ) ) ;
#6692=ORIENTED_EDGE ( 'NONE', *, *, #32808, .T. ) ;
#6705=CARTESIAN_POINT ( 'NONE',  ( 12.50000000000001066, -90.00000000000005684, -25.00000000000000000 ) ) ;
#6742=EDGE_CURVE ( 'NONE', #143487, #74970, #177432, .T. ) ;
#6795=EDGE_CURVE ( 'NONE', #140935, #23953, #150090, .T. ) ;
#6817=VERTEX_POINT ( 'NONE', #56062 ) ;
#6873=LINE ( 'NONE', #190912, #159839 ) ;
#6914=CARTESIAN_POINT ( 'NONE',  ( 16.24127373534237861, -14.59486009359520509, -56.10187840754844757 ) ) ;
#6930=CARTESIAN_POINT ( 'NONE',  ( 26.37337922943876123, -29.71119707698740697, -20.32121347158684799 ) ) ;
#6932=CARTESIAN_POINT ( 'NONE',  ( -15.06137443927361019, -15.06137443927335440, -64.92279855667830191 ) ) ;
#6941=CARTESIAN_POINT ( 'NONE',  ( 22.99604614807110181, -21.49604614807103786, -46.28618945597792589 ) ) ;
#6947=CARTESIAN_POINT ( 'NONE',  ( 22.19904868473526705, -30.74855836414197086, -22.45812049023449219 ) ) ;
#6966=DIRECTION ( 'NONE',  ( 1.000000000000000000, 0.000000000000000000, 3.469446951953612217E-15 ) ) ;
#6979=EDGE_CURVE ( 'NONE', #198657, #243, #178426, .T. ) ;
#6982=CARTESIAN_POINT ( 'NONE',  ( -1.499560036715100075, -22.98313974082796918, -57.70434786042496000 ) ) ;
#7001=CARTESIAN_POINT ( 'NONE',  ( -12.33280382558396404, -43.64415646941903049, -22.88837716264928801 ) ) ;
#7002=ORIENTED_EDGE ( 'NONE', *, *, #173288, .T. ) ;
#7013=DIRECTION ( 'NONE',  ( 0.000000000000000000, 0.000000000000000000, 1.000000000000000000 ) ) ;
#7017=DIRECTION ( 'NONE',  ( 1.000000000000000000, 0.000000000000000000, 0.000000000000000000 ) ) ;
#7028=FACE_OUTER_BOUND ( 'NONE', #115842, .T. ) ;
#7035=DIRECTION ( 'NONE',  ( -0.000000000000000000, -0.000000000000000000, 1.000000000000000000 ) ) ;
#7070=AXIS2_PLACEMENT_3D ( 'NONE', #152759, #109240, #140573 ) ;
#7074=CARTESIAN_POINT ( 'NONE',  ( 1.221313414957698099E-14, -31.90000000000003411, -64.92279855667830191 ) ) ;
#7114=ORIENTED_EDGE ( 'NONE', *, *, #149935, .F. ) ;
#7136=CARTESIAN_POINT ( 'NONE',  ( -15.35002835867562432, -17.41572776432974479, -57.57448828401508933 ) ) ;
#7153=EDGE_LOOP ( 'NONE', ( #32159, #159327, #16906, #182605 ) ) ;
#7160=DIRECTION ( 'NONE',  ( 1.000000000000000000, 0.000000000000000000, 0.000000000000000000 ) ) ;
#7186=DIRECTION ( 'NONE',  ( 0.000000000000000000, 0.000000000000000000, 1.000000000000000000 ) ) ;
#7188=DIRECTION ( 'NONE',  ( -1.000000000000000000, 0.000000000000000000, -0.000000000000000000 ) ) ;
#7211=ORIENTED_EDGE ( 'NONE', *, *, #183499, .T. ) ;
#7232=FILL_AREA_STYLE ('',( #69926 ) ) ;
#7262=CARTESIAN_POINT ( 'NONE',  ( -15.06137443927351249, 15.06137443927345210, -58.85720012050612837 ) ) ;
#7263=ORIENTED_EDGE ( 'NONE', *, *, #66362, .F. ) ;
#7317=EDGE_CURVE ( 'NONE', #142110, #123757, #172728, .T. ) ;
#7340=CARTESIAN_POINT ( 'NONE',  ( -28.26900468436335245, -28.30519395875711552, -15.36550801296253432 ) ) ;
#7343=DIRECTION ( 'NONE',  ( 0.000000000000000000, 0.000000000000000000, 1.000000000000000000 ) ) ;
#7379=VECTOR ( 'NONE', #45031, 1000.000000000000000 ) ;
#7393=DIRECTION ( 'NONE',  ( -0.000000000000000000, -0.000000000000000000, 1.000000000000000000 ) ) ;
#7406=CIRCLE ( 'NONE', #188271, 28.90000000000004476 ) ;
#7426=CARTESIAN_POINT ( 'NONE',  ( 5.267258167721604600, 6.873473828371179373, -64.05152134952703591 ) ) ;
#7432=CARTESIAN_POINT ( 'NONE',  ( 33.67159378368906175, -21.59246066468708847, -24.63947658914731420 ) ) ;
#7445=EDGE_LOOP ( 'NONE', ( #130021, #155977, #65948, #134955 ) ) ;
#7448=CARTESIAN_POINT ( 'NONE',  ( -36.91746825000000598, 2.428612866367529932E-14, -10.62499999726881406 ) ) ;
#7458=CARTESIAN_POINT ( 'NONE',  ( 30.87493573979816119, -25.21320017017430715, -21.56479137965274973 ) ) ;
#7472=ORIENTED_EDGE ( 'NONE', *, *, #110611, .F. ) ;
#7510=CARTESIAN_POINT ( 'NONE',  ( 29.86685920354754842, -21.69954338932559068, -7.824999997268813345 ) ) ;
#7544=CARTESIAN_POINT ( 'NONE',  ( 21.49604614807111602, 21.49604614807102720, -64.92279855667830191 ) ) ;
#7545=CARTESIAN_POINT ( 'NONE',  ( 11.80868324581538253, -11.80868324581533457, -61.34707691135562868 ) ) ;
#7587=CARTESIAN_POINT ( 'NONE',  ( -69.65682714487590488, -71.74905178543390605, 0.000000000000000000 ) ) ;
#7594=EDGE_CURVE ( 'NONE', #181556, #117432, #185718, .T. ) ;
#7609=EDGE_CURVE ( 'NONE', #24124, #177464, #30709, .T. ) ;
#7657=CARTESIAN_POINT ( 'NONE',  ( 22.46063206192303241, 22.65278057777875986, -45.64921306006598911 ) ) ;
#7683=CARTESIAN_POINT ( 'NONE',  ( -11.40812507854755609, 35.11059874428196537, -1.024999997268813301 ) ) ;
#7694=CARTESIAN_POINT ( 'NONE',  ( -13.70000000000001528, 1.443387660838688656E-13, -62.58071313852362039 ) ) ;
#7742=CARTESIAN_POINT ( 'NONE',  ( 29.87692619418715267, -1.408284774589644517, -48.43935853184048312 ) ) ;
#7751=( BOUNDED_CURVE ( )  B_SPLINE_CURVE ( 2, ( #44363, #121187, #110737, #174413, #30180 ),
 .UNSPECIFIED., .F., .F. ) 
 B_SPLINE_CURVE_WITH_KNOTS ( ( 3, 2, 3 ),
 ( 0.9000000000000000222, 0.9200000000000000400, 0.9255006513465138251 ),
 .UNSPECIFIED. ) 
 CURVE ( )  GEOMETRIC_REPRESENTATION_ITEM ( )  RATIONAL_B_SPLINE_CURVE ( ( 1.000000000000000000, 0.9510565162951535312, 1.000000000000000000, 0.9865389480227928498, 0.9804823514139773266 ) ) 
 REPRESENTATION_ITEM ( '' )  );
#7759=CARTESIAN_POINT ( 'NONE',  ( 14.62341493535845416, 16.00195535827008442, -58.61703605924742533 ) ) ;
#7784=CIRCLE ( 'NONE', #130448, 38.00000000000000000 ) ;
#7790=EDGE_CURVE ( 'NONE', #6179, #40990, #17513, .T. ) ;
#7839=CARTESIAN_POINT ( 'NONE',  ( -1.221313414957698099E-14, 31.90000000000003411, -65.00100000000003320 ) ) ;
#7898=CARTESIAN_POINT ( 'NONE',  ( 9.921929963571523459, -9.486473617298056382, -62.57108492361744823 ) ) ;
#7917=CARTESIAN_POINT ( 'NONE',  ( -29.32058373238548654, 1.046637022531065719, -52.18867397238356887 ) ) ;
#7938=CARTESIAN_POINT ( 'NONE',  ( 38.00000000000000711, -12.34694845685040754, -6.849999994537626868 ) ) ;
#7955=CARTESIAN_POINT ( 'NONE',  ( -0.6023940538448385729, -29.02171288343480882, -52.52077797743537957 ) ) ;
#7975=DIRECTION ( 'NONE',  ( 0.000000000000000000, 0.000000000000000000, 1.000000000000000000 ) ) ;
#7987=CARTESIAN_POINT ( 'NONE',  ( -29.86685920354755197, -21.69954338932560134, -2.924999997268813878 ) ) ;
#7988=CARTESIAN_POINT ( 'NONE',  ( -1.240847218223085413, -23.66491666289340401, -57.22545927231450946 ) ) ;
#7996=CARTESIAN_POINT ( 'NONE',  ( -0.2690448904508037087, -28.91886483090992854, -49.65045026909250225 ) ) ;
#8009=CARTESIAN_POINT ( 'NONE',  ( -6.004573588232718251, -47.77740467397597968, -24.84605846612137725 ) ) ;
#8010=EDGE_LOOP ( 'NONE', ( #184344, #148536, #25787, #20628 ) ) ;
#8026=CARTESIAN_POINT ( 'NONE',  ( 21.65895526037594010, -0.9928668394655185692, -56.20821996642038698 ) ) ;
#8030=EDGE_CURVE ( 'NONE', #120176, #111780, #137786, .T. ) ;
#8039=VECTOR ( 'NONE', #46142, 1000.000000000000000 ) ;
#8048=CARTESIAN_POINT ( 'NONE',  ( -1.136345303629771264, -6.615873399348758177, -62.40252569733547716 ) ) ;
#8068=VECTOR ( 'NONE', #126784, 1000.000000000000000 ) ;
#8069=DIRECTION ( 'NONE',  ( -0.000000000000000000, -0.000000000000000000, 1.000000000000000000 ) ) ;
#8084=DIRECTION ( 'NONE',  ( 0.000000000000000000, 0.000000000000000000, 1.000000000000000000 ) ) ;
#8114=AXIS2_PLACEMENT_3D ( 'NONE', #68843, #71847, #148699 ) ;
#8128=AXIS2_PLACEMENT_3D ( 'NONE', #113217, #146545, #159720 ) ;
#8149=CARTESIAN_POINT ( 'NONE',  ( -27.03637221620033770, -26.30952996081082773, -20.42959548696012462 ) ) ;
#8163=ORIENTED_EDGE ( 'NONE', *, *, #26705, .F. ) ;
#8170=CARTESIAN_POINT ( 'NONE',  ( 11.78083973539067486, -37.76997396076107805, -30.94638762609303129 ) ) ;
#8179=AXIS2_PLACEMENT_3D ( 'NONE', #36261, #97915, #22107 ) ;
#8188=EDGE_CURVE ( 'NONE', #144904, #70166, #146333, .T. ) ;
#8204=CARTESIAN_POINT ( 'NONE',  ( 30.74264578624799782, 22.33583958711400541, -4.800000000000000711 ) ) ;
#8210=CARTESIAN_POINT ( 'NONE',  ( 37.99999999999999289, 2.893978650043524126E-14, -4.749999994537627224 ) ) ;
#8216=ORIENTED_EDGE ( 'NONE', *, *, #29165, .T. ) ;
#8251=CARTESIAN_POINT ( 'NONE',  ( 24.54856932378043410, -28.36614238946604161, -18.58410241723692025 ) ) ;
#8341=CARTESIAN_POINT ( 'NONE',  ( 11.80868324581538253, -11.80868324581533457, -61.34707691135562868 ) ) ;
#8410=ORIENTED_EDGE ( 'NONE', *, *, #1629, .T. ) ;
#8412=ORIENTED_EDGE ( 'NONE', *, *, #195701, .F. ) ;
#8448=DIRECTION ( 'NONE',  ( -0.000000000000000000, -0.000000000000000000, -1.000000000000000000 ) ) ;
#8450=CARTESIAN_POINT ( 'NONE',  ( 16.70000000000002061, 0.000000000000000000, -59.13370768023891344 ) ) ;
#8460=CARTESIAN_POINT ( 'NONE',  ( 37.66961640367472341, -4.999999999999976019, -18.00000000000000355 ) ) ;
#8468=CARTESIAN_POINT ( 'NONE',  ( 36.91746824999999177, 2.880721459617395097E-14, -7.624999997268813168 ) ) ;
#8473=CARTESIAN_POINT ( 'NONE',  ( 0.000000000000000000, 0.000000000000000000, -64.92279855667830191 ) ) ;
#8477=CARTESIAN_POINT ( 'NONE',  ( 33.17138627372818860, -22.14683228597266762, -20.77970695692249237 ) ) ;
#8493=CARTESIAN_POINT ( 'NONE',  ( -3.573655867282028392E-15, 2.428612866367529932E-14, -23.00000000000000000 ) ) ;
#8522=ORIENTED_EDGE ( 'NONE', *, *, #6979, .T. ) ;
#8527=CARTESIAN_POINT ( 'NONE',  ( 29.86685920354754842, -21.69954338932559068, -5.824999997268813345 ) ) ;
#8550=CIRCLE ( 'NONE', #157064, 12.50000000000000000 ) ;
#8559=DIRECTION ( 'NONE',  ( -1.000000000000000000, 0.000000000000000000, 0.000000000000000000 ) ) ;
#8561=AXIS2_PLACEMENT_3D ( 'NONE', #20, #13237, #15213 ) ;
#8570=FACE_OUTER_BOUND ( 'NONE', #24783, .T. ) ;
#8580=B_SPLINE_CURVE_WITH_KNOTS ( 'NONE', 3,
 ( #163921, #72911, #166905, #105218, #180102, #182069, #134580, #183061, #73903, #195253, #152700, #149736, #198225, #56738, #118408, #121369, #135573, #43552, #196267, #41570, #120376, #44545, #167884, #197245 ),
 .UNSPECIFIED., .F., .F.,
 ( 4, 2, 2, 2, 2, 2, 2, 2, 2, 2, 2, 4 ),
 ( 0.000000000000000000, 0.002199680649073693962, 0.004399361298147387925, 0.006599041947221081887, 0.008798722596294775850, 0.01319808389444217418, 0.01759744519258957252, 0.02199680649073697605, 0.02639616778888437959, 0.03079552908703178313, 0.03299520973610547969, 0.03519489038517917973 ),
 .UNSPECIFIED. ) ;
#8599=ORIENTED_EDGE ( 'NONE', *, *, #37462, .T. ) ;
#8611=CARTESIAN_POINT ( 'NONE',  ( 27.86273085795036408, -28.69962071417356242, 0.000000000000000000 ) ) ;
#8674=B_SPLINE_CURVE_WITH_KNOTS ( 'NONE', 3,
 ( #85040, #129539, #142729, #69894, #193246, #128546, #175073, #23394, #189263, #35557, #99213, #143724, #65887, #177090, #4209, #113383, #98195, #22394, #131562, #160901, #52713, #84044, #145723, #50738 ),
 .UNSPECIFIED., .F., .F.,
 ( 4, 2, 2, 2, 2, 2, 2, 2, 2, 2, 2, 4 ),
 ( 1.970462154608161142E-07, 0.0003069708713091477670, 0.0006137446964028346478, 0.001227292346590209060, 0.001534066171683895561, 0.001840839996777582496, 0.002147613821871268997, 0.002454387646964955282, 0.003067935297152315274, 0.003681482947339676133, 0.004295030597527037426, 0.004908578247714397852 ),
 .UNSPECIFIED. ) ;
#8691=CARTESIAN_POINT ( 'NONE',  ( 11.45643923738959735, 5.000000000000007105, -18.00000000000000000 ) ) ;
#8707=CARTESIAN_POINT ( 'NONE',  ( 22.81625015709510151, -31.40387420917324590, -1.924999997268813212 ) ) ;
#8766=CARTESIAN_POINT ( 'NONE',  ( 31.61347055016709007, -0.9086318102906248972, -46.06737158113914177 ) ) ;
#8780=CARTESIAN_POINT ( 'NONE',  ( 16.44579809102488710, 17.60164288208763850, -56.93377352129066082 ) ) ;
#8791=ORIENTED_EDGE ( 'NONE', *, *, #84741, .T. ) ;
#8803=AXIS2_PLACEMENT_3D ( 'NONE', #44105, #64234, #152268 ) ;
#8828=VECTOR ( 'NONE', #50723, 1000.000000000000000 ) ;
#8896=CARTESIAN_POINT ( 'NONE',  ( -15.22666363356483821, 14.91361452257038422, -56.46021433273639190 ) ) ;
#8914=CARTESIAN_POINT ( 'NONE',  ( -3.620324696388704577, -38.95353743397183166, -23.38767721380492048 ) ) ;
#8956=DIRECTION ( 'NONE',  ( 1.000000000000000000, 0.000000000000000000, 0.000000000000000000 ) ) ;
#8959=CARTESIAN_POINT ( 'NONE',  ( 30.74264578624799782, 22.33583958711400541, -6.549999994537627046 ) ) ;
#8976=EDGE_LOOP ( 'NONE', ( #101835, #70618, #40159, #782 ) ) ;
#9011=CARTESIAN_POINT ( 'NONE',  ( 36.91746824999999177, 11.99521256947799230, -6.024999997268812635 ) ) ;
#9012=DIRECTION ( 'NONE',  ( -0.000000000000000000, -0.000000000000000000, 1.000000000000000000 ) ) ;
#9031=CARTESIAN_POINT ( 'NONE',  ( -26.41049836824041464, -29.67629096701854863, -20.30943395415518182 ) ) ;
#9045=CARTESIAN_POINT ( 'NONE',  ( -0.7565710328820600683, -8.898962301217522963, -63.99033069988504963 ) ) ;
#9059=B_SPLINE_CURVE_WITH_KNOTS ( 'NONE', 3,
 ( #31329, #123314, #76824, #138495, #90985, #122328, #75829, #28378, #966, #170834, #121340, #74855, #155659, #30333, #17155, #90016, #46492, #200177, #91974, #183033, #13192, #62642, #78808, #108153, #107157, #153668 ),
 .UNSPECIFIED., .F., .F.,
 ( 4, 2, 2, 2, 2, 2, 2, 2, 2, 2, 2, 2, 4 ),
 ( 1.971390914465818311E-07, 0.0002963316798229296048, 0.0005924662205544125584, 0.0008886007612858956746, 0.001184735302017378899, 0.001777004383480341879, 0.002369273464943304642, 0.002665408005674786349, 0.002961542546406268055, 0.003257677087137749328, 0.003553811627869231035, 0.004146080709332196183, 0.004738349790795161331 ),
 .UNSPECIFIED. ) ;
#9086=MANIFOLD_SOLID_BREP ( 'Extrude-Thin3', #40546 ) ;
#9121=CIRCLE ( 'NONE', #145522, 28.90000000000004476 ) ;
#9144=DIRECTION ( 'NONE',  ( 1.000000000000000000, 0.000000000000000000, 0.000000000000000000 ) ) ;
#9152=B_SPLINE_CURVE_WITH_KNOTS ( 'NONE', 3,
 ( #131548, #149720, #11220, #72895, #179076, #194240, #134563, #116378, #55707, #40547, #163905, #82673, #114007, #176720, #131188, #54356 ),
 .UNSPECIFIED., .F., .F.,
 ( 4, 2, 2, 2, 2, 2, 2, 4 ),
 ( 0.001191682210564843237, 0.002120961452828536587, 0.002585601073960383696, 0.003050240695092231238, 0.003514880316224078347, 0.003979519937355925456, 0.004444159558487772999, 0.004908799179619620541 ),
 .UNSPECIFIED. ) ;
#9163=CARTESIAN_POINT ( 'NONE',  ( -30.74264578624800492, 22.33583958711400186, -6.200000000000001066 ) ) ;
#9166=CARTESIAN_POINT ( 'NONE',  ( -22.19904868473514981, -30.74855836414207744, -22.45812049023462009 ) ) ;
#9187=CARTESIAN_POINT ( 'NONE',  ( 0.000000000000000000, -105.0000000000000000, 12.00000000000000355 ) ) ;
#9212=CARTESIAN_POINT ( 'NONE',  ( 19.99598863510436786, 21.26972126690560216, -52.34638024103105636 ) ) ;
#9251=ORIENTED_EDGE ( 'NONE', *, *, #115825, .T. ) ;
#9262=SPHERICAL_SURFACE ( 'NONE', #151291, 40.00000000000002132 ) ;
#9329=ORIENTED_EDGE ( 'NONE', *, *, #39985, .T. ) ;
#9338=EDGE_CURVE ( 'NONE', #120176, #41844, #186669, .T. ) ;
#9368=CARTESIAN_POINT ( 'NONE',  ( 30.74264578624800137, -22.33583958711395212, -2.949999994537626957 ) ) ;
#9417=ORIENTED_EDGE ( 'NONE', *, *, #177665, .F. ) ;
#9428=CARTESIAN_POINT ( 'NONE',  ( 0.5956237041775711560, 29.01886376551548352, -52.52392249052597606 ) ) ;
#9440=B_SPLINE_CURVE_WITH_KNOTS ( 'NONE', 3,
 ( #85746, #5905, #118097, #175771, #147433, #70589, #86745, #194941, #71583, #193948, #148429, #36241, #55411, #9924, #37246, #56417, #97893, #160596, #83736, #145415, #13886, #75552 ),
 .UNSPECIFIED., .F., .F.,
 ( 4, 2, 2, 2, 2, 2, 2, 2, 2, 2, 4 ),
 ( 1.970604704964099883E-07, 0.0003054521314110426400, 0.0006107072023515888737, 0.001221217344232681341, 0.001831727486113774242, 0.002136982557054321018, 0.002442237627994867360, 0.003052747769875972621, 0.003663257911757078315, 0.004273768053638177071, 0.004884278195519273225 ),
 .UNSPECIFIED. ) ;
#9454=B_SPLINE_CURVE_WITH_KNOTS ( 'NONE', 3,
 ( #130773, #175295, #114605, #49963, #4426, #190468, #158129, #176302, #22615, #21609, #34787, #69107, #192465, #131788, #96442, #67111, #160121, #127778, #81263, #189478, #50956, #174307, #128769, #113601, #83267, #42785 ),
 .UNSPECIFIED., .F., .F.,
 ( 4, 2, 2, 2, 2, 2, 2, 2, 2, 2, 2, 2, 4 ),
 ( 1.969502666224155977E-07, 0.0004009345686709464129, 0.0008016721870752703321, 0.001603147423883922182, 0.002404622660692573924, 0.003206097897501225449, 0.004007573134309877841, 0.004408310752714203820, 0.004809048371118529799, 0.005209785989522855779, 0.005610523607927182625, 0.006011261226331507737, 0.006411998844735834584 ),
 .UNSPECIFIED. ) ;
#9458=CARTESIAN_POINT ( 'NONE',  ( 31.90000000000003411, -9.916512055951908821E-14, -64.92279855667830191 ) ) ;
#9465=ORIENTED_EDGE ( 'NONE', *, *, #98300, .F. ) ;
#9476=ORIENTED_EDGE ( 'NONE', *, *, #127759, .T. ) ;
#9479=CARTESIAN_POINT ( 'NONE',  ( 36.91746824999999887, 11.99521256947799053, -9.524999997268812635 ) ) ;
#9488=CARTESIAN_POINT ( 'NONE',  ( 28.71286925542251112, -27.61909494970911183, -16.96471949291807135 ) ) ;
#9489=CIRCLE ( 'NONE', #106305, 48.98979485566358250 ) ;
#9537=CARTESIAN_POINT ( 'NONE',  ( 22.81625015709509441, 31.40387420917330275, -5.324999997268812457 ) ) ;
#9571=DIRECTION ( 'NONE',  ( 1.000000000000000000, 0.000000000000000000, 0.000000000000000000 ) ) ;
#9598=CARTESIAN_POINT ( 'NONE',  ( 0.000000000000000000, 0.000000000000000000, -60.44446360152740283 ) ) ;
#9658=ORIENTED_EDGE ( 'NONE', *, *, #149935, .T. ) ;
#9668=EDGE_CURVE ( 'NONE', #73091, #73471, #91628, .T. ) ;
#9714=CARTESIAN_POINT ( 'NONE',  ( -36.91746825000000598, 2.428612866367529932E-14, -2.624999997268813168 ) ) ;
#9724=DIRECTION ( 'NONE',  ( 0.000000000000000000, 0.000000000000000000, -1.000000000000000000 ) ) ;
#9769=VERTEX_POINT ( 'NONE', #14572 ) ;
#9771=CARTESIAN_POINT ( 'NONE',  ( 29.64248797448942696, -1.297617798568356573, -48.74145669546051352 ) ) ;
#9789=ORIENTED_EDGE ( 'NONE', *, *, #107496, .F. ) ;
#9807=CIRCLE ( 'NONE', #38950, 13.70000000000001528 ) ;
#9844=ORIENTED_EDGE ( 'NONE', *, *, #64870, .T. ) ;
#9918=CARTESIAN_POINT ( 'NONE',  ( -20.92307141426356409, -31.70153649905130422, -23.60833562326012469 ) ) ;
#9924=CARTESIAN_POINT ( 'NONE',  ( -1.500065973499163041, -15.01118352434400549, -62.04667436142317172 ) ) ;
#9937=DIRECTION ( 'NONE',  ( -1.000000000000000000, 0.000000000000000000, 0.000000000000000000 ) ) ;
#9960=CARTESIAN_POINT ( 'NONE',  ( -11.74264578624800670, 36.14014761921585972, -6.149999994537627579 ) ) ;
#9968=CARTESIAN_POINT ( 'NONE',  ( 69.65682714487590488, -71.74905178543389184, -15.00000000000000178 ) ) ;
#9973=CARTESIAN_POINT ( 'NONE',  ( -11.51622829137498805, 9.456233179636171826, -59.95663916823117034 ) ) ;
#9977=ORIENTED_EDGE ( 'NONE', *, *, #199123, .T. ) ;
#10010=CARTESIAN_POINT ( 'NONE',  ( -29.86685920354755197, -21.69954338932560134, -4.924999997268813878 ) ) ;
#10011=CARTESIAN_POINT ( 'NONE',  ( -0.8101246706333771197, -24.06642195515787108, -56.93999021579659825 ) ) ;
#10033=CARTESIAN_POINT ( 'NONE',  ( -28.71047547314692849, -27.16362253576033936, -18.60589795198331231 ) ) ;
#10047=CARTESIAN_POINT ( 'NONE',  ( 24.20415418211126735, -0.5379555815578801470, -54.28961862586979237 ) ) ;
#10054=CARTESIAN_POINT ( 'NONE',  ( 28.47622644277404191, -25.16156846422445881, -16.68312038616162241 ) ) ;
#10059=CARTESIAN_POINT ( 'NONE',  ( 0.4034547045401649656, 16.64828639225574136, -61.36869763530247468 ) ) ;
#10071=EDGE_CURVE ( 'NONE', #170287, #25627, #21017, .T. ) ;
#10075=ORIENTED_EDGE ( 'NONE', *, *, #1629, .F. ) ;
#10139=EDGE_CURVE ( 'NONE', #35858, #196503, #111377, .T. ) ;
#10145=LINE ( 'NONE', #149649, #28034 ) ;
#10180=ORIENTED_EDGE ( 'NONE', *, *, #14847, .F. ) ;
#10187=CARTESIAN_POINT ( 'NONE',  ( -1.734723475976807094E-15, 15.20000000000001883, -65.00100000000003320 ) ) ;
#10202=ORIENTED_EDGE ( 'NONE', *, *, #2366, .F. ) ;
#10232=CARTESIAN_POINT ( 'NONE',  ( 9.090093023806478101, -0.1983487321476342102, -63.95305636720453890 ) ) ;
#10269=EDGE_LOOP ( 'NONE', ( #111846, #198402 ) ) ;
#10295=ORIENTED_EDGE ( 'NONE', *, *, #53802, .T. ) ;
#10328=ORIENTED_EDGE ( 'NONE', *, *, #136461, .F. ) ;
#10331=CARTESIAN_POINT ( 'NONE',  ( 1.500000000000163203, 7.503014402978025466, -64.26148919578614027 ) ) ;
#10361=FACE_OUTER_BOUND ( 'NONE', #38175, .T. ) ;
#10416=DIRECTION ( 'NONE',  ( 0.000000000000000000, 0.000000000000000000, -1.000000000000000000 ) ) ;
#10459=CYLINDRICAL_SURFACE ( 'NONE', #137253, 216.0437394197456342 ) ;
#10478=CARTESIAN_POINT ( 'NONE',  ( -5.950531402560715689E-15, 38.81732327939063509, -7.124999997268814944 ) ) ;
#10502=ORIENTED_EDGE ( 'NONE', *, *, #34682, .T. ) ;
#10504=CARTESIAN_POINT ( 'NONE',  ( 3.503282210674364627, -48.86437366581479580, -23.00000000000000355 ) ) ;
#10537=CARTESIAN_POINT ( 'NONE',  ( 36.91746824999999177, 2.880721459617395097E-14, -7.624999997268813168 ) ) ;
#10541=CARTESIAN_POINT ( 'NONE',  ( 4.802760416696449930, -3.979030490183114388, -64.51105135991079464 ) ) ;
#10566=CARTESIAN_POINT ( 'NONE',  ( -3.573655867282028392E-15, 2.428612866367529932E-14, -25.00000000000000000 ) ) ;
#10573=DIRECTION ( 'NONE',  ( -1.000000000000000000, 0.000000000000000000, 0.000000000000000000 ) ) ;
#10577=B_SPLINE_CURVE_WITH_KNOTS ( 'NONE', 3,
 ( #194721, #10704, #56191, #83512, #190715, #175542, #130002, #149213, #54198, #178551, #162365, #71367, #113846, #145189, #6673, #25881, #147205, #40017, #37017, #193723, #98678, #68351, #132034, #87526 ),
 .UNSPECIFIED., .F., .F.,
 ( 4, 2, 2, 2, 2, 2, 2, 2, 2, 2, 2, 4 ),
 ( 0.02035494470246975926, 0.02303009228666412500, 0.02570523987085848727, 0.02838038745505284954, 0.02971796124715003068, 0.03105553503924721181, 0.03172432193529579891, 0.03239310883134438601, 0.03373068262344156021, 0.03640583020763589472, 0.03908097779183024312, 0.04175612537602457763 ),
 .UNSPECIFIED. ) ;
#10598=LINE ( 'NONE', #57100, #90607 ) ;
#10682=ADVANCED_FACE ( 'NONE', ( #99351 ), #192219, .F. ) ;
#10688=CARTESIAN_POINT ( 'NONE',  ( -24.24789025133655329, -29.25582059975612026, -16.65643465479912066 ) ) ;
#10704=CARTESIAN_POINT ( 'NONE',  ( -21.02068080879918455, -34.03872152684794372, -24.45646120681623970 ) ) ;
#10711=ORIENTED_EDGE ( 'NONE', *, *, #86821, .T. ) ;
#10714=CARTESIAN_POINT ( 'NONE',  ( -29.86685920354755197, -21.69954338932560134, -6.424999997268812990 ) ) ;
#10724=CYLINDRICAL_SURFACE ( 'NONE', #120397, 38.00000000000000000 ) ;
#10749=EDGE_LOOP ( 'NONE', ( #29190, #196064, #83348, #49237, #191422 ) ) ;
#10773=CARTESIAN_POINT ( 'NONE',  ( 31.48176515315800117, -1.054302444749900536, -46.25693415911322859 ) ) ;
#10789=ORIENTED_EDGE ( 'NONE', *, *, #32449, .T. ) ;
#10796=ORIENTED_EDGE ( 'NONE', *, *, #66362, .T. ) ;
#10848=( NAMED_UNIT ( * ) SI_UNIT ( $, .STERADIAN. ) SOLID_ANGLE_UNIT ( ) );
#10897=CARTESIAN_POINT ( 'NONE',  ( -16.60031353666876797, 14.64731493820422514, -55.88827192845551650 ) ) ;
#10904=TOROIDAL_SURFACE ( 'NONE', #43230, 206.0437394197456342, 8.000000000000000000 ) ;
#10919=CARTESIAN_POINT ( 'NONE',  ( 11.92407319027615920, -9.806099294356528162, -61.90095559709221362 ) ) ;
#10933=CARTESIAN_POINT ( 'NONE',  ( 0.000000000000000000, 0.000000000000000000, -49.67367017693150189 ) ) ;
#10949=ORIENTED_EDGE ( 'NONE', *, *, #115458, .F. ) ;
#10952=CARTESIAN_POINT ( 'NONE',  ( 27.33089735363351735, -28.79505088701976234, -20.09366309423206687 ) ) ;
#10956=CARTESIAN_POINT ( 'NONE',  ( -11.74264578624800670, 36.14014761921585972, -10.14999999453762669 ) ) ;
#10969=CARTESIAN_POINT ( 'NONE',  ( 11.30153831258470731, -180.0000000000000000, -15.00000000000000178 ) ) ;
#10973=ORIENTED_EDGE ( 'NONE', *, *, #159157, .F. ) ;
#10981=CARTESIAN_POINT ( 'NONE',  ( -21.30000000000002913, 2.244099063931684814E-13, -58.85720012050612837 ) ) ;
#11007=CARTESIAN_POINT ( 'NONE',  ( -11.40812507854754720, -35.11059874428192273, -2.724999997268813257 ) ) ;
#11022=DIRECTION ( 'NONE',  ( 0.000000000000000000, 0.000000000000000000, 1.000000000000000000 ) ) ;
#11029=CARTESIAN_POINT ( 'NONE',  ( -27.35218628822427434, -28.77384467243344801, -20.10380102094744714 ) ) ;
#11044=CARTESIAN_POINT ( 'NONE',  ( 24.23981148858513635, -0.4346045811322880037, -54.26183423998838862 ) ) ;
#11057=DIRECTION ( 'NONE',  ( 1.000000000000000000, 0.000000000000000000, 0.000000000000000000 ) ) ;
#11058=CARTESIAN_POINT ( 'NONE',  ( 6.615299585309121433, -1.135848680322177451, -64.43295106733367561 ) ) ;
#11102=CIRCLE ( 'NONE', #36896, 40.00000000000000000 ) ;
#11138=CIRCLE ( 'NONE', #124106, 5.000000000000000000 ) ;
#11182=ORIENTED_EDGE ( 'NONE', *, *, #90658, .T. ) ;
#11189=DIRECTION ( 'NONE',  ( -0.000000000000000000, -0.000000000000000000, 1.000000000000000000 ) ) ;
#11214=LINE ( 'NONE', #24388, #41679 ) ;
#11220=CARTESIAN_POINT ( 'NONE',  ( -9.338429343928289939, -11.33503711070567554, -60.04863804042465603 ) ) ;
#11224=CIRCLE ( 'NONE', #104733, 206.0437394197456911 ) ;
#11244=AXIS2_PLACEMENT_3D ( 'NONE', #190710, #5674, #51195 ) ;
#11253=CIRCLE ( 'NONE', #175759, 38.00000000000000000 ) ;
#11291=EDGE_CURVE ( 'NONE', #174271, #70701, #154452, .T. ) ;
#11297=B_SPLINE_CURVE_WITH_KNOTS ( 'NONE', 3,
 ( #2027, #50533, #35354, #97005, #63707, #20176, #125382, #4995, #81822, #48548, #66680, #190041, #51515, #113177, #67676, #146506, #37339, #5997, #39343, #84826, #129334, #52504, #85843, #7996, #68671, #175867 ),
 .UNSPECIFIED., .F., .F.,
 ( 4, 2, 2, 2, 2, 2, 2, 2, 2, 2, 2, 2, 4 ),
 ( 1.969502665979568066E-07, 0.0004009345686709217473, 0.0008016721870752456123, 0.001603147423883905052, 0.002404622660692559612, 0.003206097897501214173, 0.004007573134309868300, 0.004408310752714196014, 0.004809048371118523728, 0.005209785989522850574, 0.005610523607927177421, 0.006011261226331506002, 0.006411998844735832849 ),
 .UNSPECIFIED. ) ;
#11338=DIRECTION ( 'NONE',  ( 0.000000000000000000, 0.000000000000000000, 1.000000000000000000 ) ) ;
#11359=AXIS2_PLACEMENT_3D ( 'NONE', #104342, #74016, #72008 ) ;
#11365=DIRECTION ( 'NONE',  ( 0.9526137857479317628, 0.3041824702427701199, 0.000000000000000000 ) ) ;
#11371=CARTESIAN_POINT ( 'NONE',  ( 37.99999999999999289, 2.893978650043524126E-14, -2.749999994537626780 ) ) ;
#11374=DIRECTION ( 'NONE',  ( 0.000000000000000000, 0.000000000000000000, 1.000000000000000000 ) ) ;
#11421=VERTEX_POINT ( 'NONE', #25552 ) ;
#11425=VERTEX_POINT ( 'NONE', #73041 ) ;
#11437=CARTESIAN_POINT ( 'NONE',  ( 0.2521225200370412201, 28.91645205756829995, -52.63676493945838075 ) ) ;
#11450=CARTESIAN_POINT ( 'NONE',  ( 11.30153831258471797, -180.0000000000000000, -15.00000000000000178 ) ) ;
#11453=ORIENTED_EDGE ( 'NONE', *, *, #92250, .F. ) ;
#11486=CARTESIAN_POINT ( 'NONE',  ( -30.74264578624800492, 22.33583958711400186, -8.200000000000001066 ) ) ;
#11518=ORIENTED_EDGE ( 'NONE', *, *, #6742, .T. ) ;
#11548=CARTESIAN_POINT ( 'NONE',  ( -29.86685920354755552, 21.69954338932564397, -4.824999997268814234 ) ) ;
#11583=DIRECTION ( 'NONE',  ( 0.000000000000000000, 0.000000000000000000, 1.000000000000000000 ) ) ;
#11606=DIRECTION ( 'NONE',  ( -0.000000000000000000, -0.000000000000000000, 1.000000000000000000 ) ) ;
#11677=AXIS2_PLACEMENT_3D ( 'NONE', #24067, #85722, #21057 ) ;
#11698=CARTESIAN_POINT ( 'NONE',  ( -17.41079204577539841, -36.66972510653778983, -18.74440029985510137 ) ) ;
#11722=CARTESIAN_POINT ( 'NONE',  ( 3.556970738554034288E-15, -38.81732327939057114, -6.124999997268812280 ) ) ;
#11724=AXIS2_PLACEMENT_3D ( 'NONE', #75086, #119618, #27627 ) ;
#11729=EDGE_CURVE ( 'NONE', #177464, #140780, #41494, .T. ) ;
#11773=CIRCLE ( 'NONE', #89245, 206.0437394197456342 ) ;
#11807=ORIENTED_EDGE ( 'NONE', *, *, #91315, .F. ) ;
#11846=EDGE_CURVE ( 'NONE', #137572, #36107, #198420, .T. ) ;
#11961=ORIENTED_EDGE ( 'NONE', *, *, #125347, .T. ) ;
#11967=CARTESIAN_POINT ( 'NONE',  ( 11.74264578624799427, 36.14014761921585972, -6.349999994537625980 ) ) ;
#12021=CARTESIAN_POINT ( 'NONE',  ( 29.86685920354754842, -21.69954338932559068, -6.324999997268814234 ) ) ;
#12042=CARTESIAN_POINT ( 'NONE',  ( -28.32820575348087644, -27.54591730359596369, -18.54425385669249593 ) ) ;
#12058=CARTESIAN_POINT ( 'NONE',  ( -1.452908486251138553, -7.214655873249289364, -64.31726809345073548 ) ) ;
#12070=CARTESIAN_POINT ( 'NONE',  ( -6.434671708797603529, 6.434671708797564449, -65.00100000000003320 ) ) ;
#12078=CARTESIAN_POINT ( 'NONE',  ( -37.45873412500000654, 2.428612866367529932E-14, -0.3124999986344065839 ) ) ;
#12139=VERTEX_POINT ( 'NONE', #39445 ) ;
#12177=AXIS2_PLACEMENT_3D ( 'NONE', #82012, #99198, #7188 ) ;
#12178=FACE_OUTER_BOUND ( 'NONE', #174880, .T. ) ;
#12187=EDGE_LOOP ( 'NONE', ( #74168, #95274, #89424, #11518 ) ) ;
#12191=ORIENTED_EDGE ( 'NONE', *, *, #62085, .T. ) ;
#12220=CARTESIAN_POINT ( 'NONE',  ( 21.16989542479042186, 22.97168310438076588, -49.98402367076291597 ) ) ;
#12238=DIRECTION ( 'NONE',  ( 6.938893903907222461E-16, -1.000000000000000000, 0.000000000000000000 ) ) ;
#12263=CARTESIAN_POINT ( 'NONE',  ( -4.990514878257755527, 3.920520744267788960, -64.49346902751020139 ) ) ;
#12309=AXIS2_PLACEMENT_3D ( 'NONE', #85796, #147482, #127299 ) ;
#12327=CARTESIAN_POINT ( 'NONE',  ( 2.500000000000000000, -105.0000000000000000, 12.00000000000000355 ) ) ;
#12332=DIRECTION ( 'NONE',  ( -0.000000000000000000, -0.000000000000000000, 1.000000000000000000 ) ) ;
#12418=VERTEX_POINT ( 'NONE', #22450 ) ;
#12459=FACE_OUTER_BOUND ( 'NONE', #41122, .T. ) ;
#12461=CARTESIAN_POINT ( 'NONE',  ( 15.76708390931707093, -14.65644741022703990, -58.71372985409217904 ) ) ;
#12464=CARTESIAN_POINT ( 'NONE',  ( 15.29496450215404479, -1.499960427298778098, -59.75377357153833913 ) ) ;
#12467=LINE ( 'NONE', #30590, #65903 ) ;
#12481=CARTESIAN_POINT ( 'NONE',  ( -30.74264578624800492, -22.33583958711396278, -3.799999999999999822 ) ) ;
#12486=CARTESIAN_POINT ( 'NONE',  ( 0.1038182526441163017, 16.70000000000002061, -59.13370768023889923 ) ) ;
#12506=CARTESIAN_POINT ( 'NONE',  ( -20.43538597629143538, -20.43538597629106945, -52.65483682830182488 ) ) ;
#12539=CARTESIAN_POINT ( 'NONE',  ( -69.65682714487590488, -71.74905178543390605, -23.00000000000000000 ) ) ;
#12613=DIRECTION ( 'NONE',  ( 0.000000000000000000, 0.000000000000000000, 1.000000000000000000 ) ) ;
#12679=AXIS2_PLACEMENT_3D ( 'NONE', #156904, #121577, #76070 ) ;
#12683=CARTESIAN_POINT ( 'NONE',  ( -9.444085519387874328, -44.71325174467975216, -21.93802053968664367 ) ) ;
#12689=CARTESIAN_POINT ( 'NONE',  ( -14.62203461105063873, -16.12203461105573865, -58.56003730381080175 ) ) ;
#12707=CARTESIAN_POINT ( 'NONE',  ( 36.91746824999999887, -11.99521256947793546, -5.724999997268813701 ) ) ;
#12724=CARTESIAN_POINT ( 'NONE',  ( 12.33280382558395871, -43.64415646942563853, -22.88837716264674427 ) ) ;
#12763=EDGE_CURVE ( 'NONE', #127568, #188843, #6263, .T. ) ;
#12839=VERTEX_POINT ( 'NONE', #38619 ) ;
#12851=AXIS2_PLACEMENT_3D ( 'NONE', #92936, #50438, #200135 ) ;
#12911=CYLINDRICAL_SURFACE ( 'NONE', #115324, 31.90000000000003411 ) ;
#12949=CARTESIAN_POINT ( 'NONE',  ( 36.91746824999999177, 2.880721459617395097E-14, -4.124999997268813168 ) ) ;
#12955=CIRCLE ( 'NONE', #41979, 10.00000000000000000 ) ;
#12984=AXIS2_PLACEMENT_3D ( 'NONE', #30466, #31461, #136645 ) ;
#13002=CARTESIAN_POINT ( 'NONE',  ( 36.91746824999999887, -11.99521256947793546, -10.22499999726881548 ) ) ;
#13022=CARTESIAN_POINT ( 'NONE',  ( -32.73422133880766438, -23.92350924394295575, -17.85299461211518590 ) ) ;
#13037=CARTESIAN_POINT ( 'NONE',  ( 193.3062444957835453, -155.7167183371837496, -15.00000000000000178 ) ) ;
#13049=FACE_OUTER_BOUND ( 'NONE', #133371, .T. ) ;
#13135=PLANE ( 'NONE',  #131319 ) ;
#13189=ORIENTED_EDGE ( 'NONE', *, *, #23592, .T. ) ;
#13192=CARTESIAN_POINT ( 'NONE',  ( -6.615873399348746631, 1.136345303629841208, -62.40252569733544874 ) ) ;
#13199=FACE_OUTER_BOUND ( 'NONE', #110358, .T. ) ;
#13201=CARTESIAN_POINT ( 'NONE',  ( -1.040834085586084257E-14, 30.40000000000003766, -65.00100000000003320 ) ) ;
#13219=CARTESIAN_POINT ( 'NONE',  ( -5.512880932802044498, -6.874811933691526988, -64.01752234774738781 ) ) ;
#13237=DIRECTION ( 'NONE',  ( 0.000000000000000000, 0.000000000000000000, -1.000000000000000000 ) ) ;
#13254=ORIENTED_EDGE ( 'NONE', *, *, #8188, .F. ) ;
#13317=DIRECTION ( 'NONE',  ( -0.000000000000000000, -0.000000000000000000, 1.000000000000000000 ) ) ;
#13335=DIRECTION ( 'NONE',  ( 1.000000000000000000, 0.000000000000000000, 0.000000000000000000 ) ) ;
#13398=CARTESIAN_POINT ( 'NONE',  ( -37.99999999999997158, 12.34694845685052123, -7.849999994537627757 ) ) ;
#13433=CARTESIAN_POINT ( 'NONE',  ( -3.874011537017657769, -5.276777131403250998, -64.46083232413522524 ) ) ;
#13437=DIRECTION ( 'NONE',  ( 1.000000000000000000, 0.000000000000000000, 0.000000000000000000 ) ) ;
#13451=CARTESIAN_POINT ( 'NONE',  ( -11.74264578624799782, -36.14014761921581709, -3.600000000000000533 ) ) ;
#13480=ORIENTED_EDGE ( 'NONE', *, *, #164374, .T. ) ;
#13507=CARTESIAN_POINT ( 'NONE',  ( 8.388830574159379737E-16, 13.70000000000001528, -62.58071313852362039 ) ) ;
#13590=CARTESIAN_POINT ( 'NONE',  ( 15.33930553228143800, 17.41439684931609122, -55.09142748592169170 ) ) ;
#13613=B_SPLINE_CURVE_WITH_KNOTS ( 'NONE', 3,
 ( #148994, #12486, #26655, #87310, #54976, #55973, #88297, #134832, #196511, #181335, #57981, #89302, #23646, #164167, #193498, #119653 ),
 .UNSPECIFIED., .F., .F.,
 ( 4, 2, 2, 2, 2, 2, 2, 4 ),
 ( 1.970462154302192724E-07, 0.0003070558431632680260, 0.0006139146401111058486, 0.001227632234006777482, 0.001534491030954616064, 0.001841349827902454645, 0.002148208624850302551, 0.002455067421798150240 ),
 .UNSPECIFIED. ) ;
#13639=CARTESIAN_POINT ( 'NONE',  ( -25.08997344982928013, -28.19247641866677512, -20.54396225644688556 ) ) ;
#13670=CARTESIAN_POINT ( 'NONE',  ( 20.82780142840221060, -20.15002084202731680, -52.57152731843168425 ) ) ;
#13676=EDGE_LOOP ( 'NONE', ( #5390, #89021, #93737, #165098, #128042 ) ) ;
#13679=CARTESIAN_POINT ( 'NONE',  ( 11.40812507854755253, -35.11059874428192273, -10.02499999726881441 ) ) ;
#13697=CARTESIAN_POINT ( 'NONE',  ( 11.94140034372758308, -38.57382067147720761, -24.90972908440997458 ) ) ;
#13699=CARTESIAN_POINT ( 'NONE',  ( -10.27527212369962406, -12.17889776840641325, -61.68947035941219070 ) ) ;
#13738=ORIENTED_EDGE ( 'NONE', *, *, #199554, .T. ) ;
#13753=CARTESIAN_POINT ( 'NONE',  ( -38.00000000000000711, 12.34694845685046438, -2.100000000000000089 ) ) ;
#13788=B_SPLINE_CURVE_WITH_KNOTS ( 'NONE', 3,
 ( #61699, #169890, #123368, #15218, #43577, #185061, #12263, #73927, #108211, #107210, #76877, #167908, #104250, #138547, #119429, #196289, #29408, #199242, #59724, #88073, #28430, #134603, #181113, #91038, #197268, #42587 ),
 .UNSPECIFIED., .F., .F.,
 ( 4, 2, 2, 2, 2, 2, 2, 2, 2, 2, 2, 2, 4 ),
 ( 2.788292423116888737E-07, 0.0002961032055655217791, 0.0005919275818887318732, 0.0008877519582119420757, 0.001183576334535152170, 0.001775225087181574743, 0.002366873839827997750, 0.002662698216151209146, 0.002958522592474420107, 0.003254346968797631502, 0.003550171345120842030, 0.004141820097767267422, 0.004733468850413692815 ),
 .UNSPECIFIED. ) ;
#13857=ORIENTED_EDGE ( 'NONE', *, *, #87886, .F. ) ;
#13873=EDGE_CURVE ( 'NONE', #88773, #51008, #143542, .T. ) ;
#13886=CARTESIAN_POINT ( 'NONE',  ( -0.2066332630086595012, -13.70000000000001528, -62.58071313852357775 ) ) ;
#13903=CARTESIAN_POINT ( 'NONE',  ( -1.315686079477255355, -15.92681084339658781, -59.47631410104520455 ) ) ;
#13923=CARTESIAN_POINT ( 'NONE',  ( -38.00000000000001421, -12.34694845685042708, -11.64999999453762669 ) ) ;
#13940=ADVANCED_FACE ( 'NONE', ( #42618 ), #105272, .F. ) ;
#13947=CARTESIAN_POINT ( 'NONE',  ( -24.30000000000003268, 0.1103568551768616401, -56.77278709839603010 ) ) ;
#13972=CARTESIAN_POINT ( 'NONE',  ( -22.73749492396214933, -155.7167183371837496, -15.00000000000000178 ) ) ;
#13973=CARTESIAN_POINT ( 'NONE',  ( 29.86685920354754487, 21.69954338932564752, -9.924999997268812990 ) ) ;
#13976=CARTESIAN_POINT ( 'NONE',  ( 1.500000000000008438, 22.80000000000002913, -57.83153971412246364 ) ) ;
#14062=B_SPLINE_CURVE_WITH_KNOTS ( 'NONE', 3,
 ( #113867, #160394, #21883, #115889, #100704, #162384, #147226, #85539, #159034, #190390, #34710, #47908 ),
 .UNSPECIFIED., .F., .F.,
 ( 4, 2, 2, 2, 2, 4 ),
 ( -5.955746802939833779E-05, 0.001235637542566280249, 0.002530832553161958733, 0.005121222574353310499, 0.007711612595544660963, 0.01030200261673601056 ),
 .UNSPECIFIED. ) ;
#14120=CARTESIAN_POINT ( 'NONE',  ( -6.502951376627836844, 4.381595247748321320, -62.18229462841632937 ) ) ;
#14136=ORIENTED_EDGE ( 'NONE', *, *, #6145, .T. ) ;
#14142=DIRECTION ( 'NONE',  ( 1.000000000000000000, 0.000000000000000000, 0.000000000000000000 ) ) ;
#14171=DIRECTION ( 'NONE',  ( 0.000000000000000000, 0.000000000000000000, 1.000000000000000000 ) ) ;
#14189=CARTESIAN_POINT ( 'NONE',  ( -3.896019243642140584, -5.669039853121431882, -64.40437979500936194 ) ) ;
#14215=CARTESIAN_POINT ( 'NONE',  ( -19.99604614807126524, -21.49604614807087799, -49.12629558063592583 ) ) ;
#14282=VECTOR ( 'NONE', #46913, 1000.000000000000000 ) ;
#14283=CARTESIAN_POINT ( 'NONE',  ( 22.99604614807109826, -21.66199780171331923, -49.53544670972640773 ) ) ;
#14286=EDGE_LOOP ( 'NONE', ( #183716, #59594, #152016, #13480 ) ) ;
#14291=ORIENTED_EDGE ( 'NONE', *, *, #192660, .T. ) ;
#14292=CARTESIAN_POINT ( 'NONE',  ( 193.3062444957835453, -155.7167183371837496, -15.00000000000000178 ) ) ;
#14301=EDGE_CURVE ( 'NONE', #176889, #29612, #38026, .T. ) ;
#14345=EDGE_CURVE ( 'NONE', #48561, #19028, #114532, .T. ) ;
#14377=VERTEX_POINT ( 'NONE', #39023 ) ;
#14389=CARTESIAN_POINT ( 'NONE',  ( 16.64831001466047056, -0.4033639900674985679, -61.36868776158050309 ) ) ;
#14403=CARTESIAN_POINT ( 'NONE',  ( -33.78191506369886810, -21.41920200728862511, -24.99999999999999289 ) ) ;
#14428=AXIS2_PLACEMENT_3D ( 'NONE', #96766, #158455, #89350 ) ;
#14437=CARTESIAN_POINT ( 'NONE',  ( -38.00000000000000711, 2.428612866367529932E-14, -6.000000000000000000 ) ) ;
#14447=CARTESIAN_POINT ( 'NONE',  ( 1.304248841091933035E-15, 21.30000000000002913, -58.85720012050612837 ) ) ;
#14463=CARTESIAN_POINT ( 'NONE',  ( 16.29108346408296271, -34.51247628902855524, -22.00899094813389567 ) ) ;
#14489=AXIS2_PLACEMENT_3D ( 'NONE', #152770, #138593, #183130 ) ;
#14492=ORIENTED_EDGE ( 'NONE', *, *, #41383, .F. ) ;
#14545=VECTOR ( 'NONE', #30827, 1000.000000000000000 ) ;
#14557=CARTESIAN_POINT ( 'NONE',  ( 1.500000000000011102, 30.56489079787948882, -50.76047248289020786 ) ) ;
#14572=CARTESIAN_POINT ( 'NONE',  ( -6.100000000000006750, 6.426762577456935076E-14, -62.50719930893269805 ) ) ;
#14575=CARTESIAN_POINT ( 'NONE',  ( 69.65682714487590488, -71.74905178543389184, -25.00000000000000000 ) ) ;
#14584=CARTESIAN_POINT ( 'NONE',  ( -20.15904164509370489, -22.18854071326290622, -51.48245768792372701 ) ) ;
#14625=LINE ( 'NONE', #108611, #92092 ) ;
#14634=CARTESIAN_POINT ( 'NONE',  ( -21.12688062493582919, -32.57662631298939715, -17.38946437510490028 ) ) ;
#14651=DIRECTION ( 'NONE',  ( 1.000000000000000000, 0.000000000000000000, 0.000000000000000000 ) ) ;
#14656=CARTESIAN_POINT ( 'NONE',  ( 21.36642364538387540, -19.99951666465409517, -49.23853142240816538 ) ) ;
#14664=CARTESIAN_POINT ( 'NONE',  ( 21.08147685851793440, -20.05196361705210961, -52.44995202553442226 ) ) ;
#14674=CARTESIAN_POINT ( 'NONE',  ( -29.86685920354755197, -21.69954338932560134, -10.42499999726881299 ) ) ;
#14685=CARTESIAN_POINT ( 'NONE',  ( -8.673617379884035472E-16, 7.600000000000007638, -65.00100000000003320 ) ) ;
#14693=FACE_OUTER_BOUND ( 'NONE', #153595, .T. ) ;
#14695=AXIS2_PLACEMENT_3D ( 'NONE', #155720, #171893, #142537 ) ;
#14774=CARTESIAN_POINT ( 'NONE',  ( 0.7794527325549597263, 16.49732430514584536, -61.43175061772111434 ) ) ;
#14780=CYLINDRICAL_SURFACE ( 'NONE', #68898, 38.00000000000000000 ) ;
#14847=EDGE_CURVE ( 'NONE', #71084, #110784, #112856, .T. ) ;
#14859=ORIENTED_EDGE ( 'NONE', *, *, #26654, .T. ) ;
#14869=AXIS2_PLACEMENT_3D ( 'NONE', #50951, #127773, #66107 ) ;
#14890=DIRECTION ( 'NONE',  ( -1.000000000000000000, 6.391086490440866478E-16, 0.000000000000000000 ) ) ;
#14903=CARTESIAN_POINT ( 'NONE',  ( -22.55670631985108443, -22.55670631985069008, -49.13275782002545355 ) ) ;
#14906=CARTESIAN_POINT ( 'NONE',  ( -1.499960427298724808, -15.29496450215404479, -59.75377357153833913 ) ) ;
#14918=EDGE_CURVE ( 'NONE', #27850, #16723, #196723, .T. ) ;
#14923=ORIENTED_EDGE ( 'NONE', *, *, #103523, .F. ) ;
#14929=CARTESIAN_POINT ( 'NONE',  ( 11.40812507854755253, -35.11059874428192273, -4.524999997268813523 ) ) ;
#14941=CARTESIAN_POINT ( 'NONE',  ( 3.875073520655164305, 5.577594645134329454, -62.38867879588715937 ) ) ;
#14978=CARTESIAN_POINT ( 'NONE',  ( 1.500000000004810818, 7.599999999999482725, -64.24270632869257724 ) ) ;
#14992=EDGE_LOOP ( 'NONE', ( #82068, #49986, #96774, #10711, #167686 ) ) ;
#15024=CARTESIAN_POINT ( 'NONE',  ( -16.70000000000002061, 1.759457951533292443E-13, -59.13370768023891344 ) ) ;
#15054=CIRCLE ( 'NONE', #92542, 10.00000000000000000 ) ;
#15073=EDGE_CURVE ( 'NONE', #27924, #56776, #115942, .T. ) ;
#15093=ORIENTED_EDGE ( 'NONE', *, *, #76762, .T. ) ;
#15101=DIRECTION ( 'NONE',  ( 0.000000000000000000, 0.000000000000000000, 1.000000000000000000 ) ) ;
#15137=VERTEX_POINT ( 'NONE', #29833 ) ;
#15143=CYLINDRICAL_SURFACE ( 'NONE', #47671, 2.500000000000000000 ) ;
#15175=CARTESIAN_POINT ( 'NONE',  ( 21.31248648291599324, -0.2211803504529610831, -58.84879416108399397 ) ) ;
#15213=DIRECTION ( 'NONE',  ( 1.000000000000000000, 2.486899575160350335E-14, 0.000000000000000000 ) ) ;
#15218=CARTESIAN_POINT ( 'NONE',  ( -4.624734593510437364, 4.070821633784361460, -64.52277792523199196 ) ) ;
#15264=CARTESIAN_POINT ( 'NONE',  ( 193.3062444957835453, -155.7167183371837496, 0.000000000000000000 ) ) ;
#15297=CARTESIAN_POINT ( 'NONE',  ( 0.000000000000000000, -165.0000000000000000, 7.000000000000003553 ) ) ;
#15305=VECTOR ( 'NONE', #129287, 1000.000000000000000 ) ;
#15323=CARTESIAN_POINT ( 'NONE',  ( -8.516692751257721739, 1.203296689329442115, -64.06477955746665032 ) ) ;
#15326=LINE ( 'NONE', #18319, #111594 ) ;
#15377=VERTEX_POINT ( 'NONE', #102695 ) ;
#15417=CARTESIAN_POINT ( 'NONE',  ( -4.025060008621055729, -4.710691162182125247, -64.51731263004398897 ) ) ;
#15422=FACE_BOUND ( 'NONE', #277, .T. ) ;
#15427=CARTESIAN_POINT ( 'NONE',  ( -15.80137536867090908, 14.65320595882610277, -58.69884337265983021 ) ) ;
#15437=CARTESIAN_POINT ( 'NONE',  ( 11.74264578624800315, -36.14014761921581709, -7.400000000000000355 ) ) ;
#15465=CARTESIAN_POINT ( 'NONE',  ( 21.12688062493369756, -32.57662631299258749, -17.38946437510359644 ) ) ;
#15497=CARTESIAN_POINT ( 'NONE',  ( 0.4080409027416297962, 13.74233039485027774, -62.56360233571632534 ) ) ;
#15578=CARTESIAN_POINT ( 'NONE',  ( 14.65109730209616146, 15.81114279943204437, -56.29481432398279139 ) ) ;
#15614=EDGE_CURVE ( 'NONE', #126569, #38777, #76319, .T. ) ;
#15629=CARTESIAN_POINT ( 'NONE',  ( -16.63682861930514889, -37.51503513662309075, -19.06746308534875922 ) ) ;
#15652=CYLINDRICAL_SURFACE ( 'NONE', #42200, 38.00000000000000000 ) ;
#15676=ORIENTED_EDGE ( 'NONE', *, *, #158416, .F. ) ;
#15688=CARTESIAN_POINT ( 'NONE',  ( 9.646990561632259542, -38.22155086790374412, -31.80034568179171472 ) ) ;
#15771=DIRECTION ( 'NONE',  ( -1.000000000000000000, 0.000000000000000000, 0.000000000000000000 ) ) ;
#15772=DIRECTION ( 'NONE',  ( 0.000000000000000000, 0.000000000000000000, 1.000000000000000000 ) ) ;
#15782=CARTESIAN_POINT ( 'NONE',  ( -5.000000000000000888, 4.999999999999999112, -18.00000000000000000 ) ) ;
#15803=ORIENTED_EDGE ( 'NONE', *, *, #168981, .T. ) ;
#15852=EDGE_CURVE ( 'NONE', #138825, #77704, #2401, .T. ) ;
#15882=DIRECTION ( 'NONE',  ( -0.000000000000000000, -0.000000000000000000, 1.000000000000000000 ) ) ;
#15902=CARTESIAN_POINT ( 'NONE',  ( -0.2077008434174324458, -13.70000000000001705, -60.44446360152740993 ) ) ;
#15908=CARTESIAN_POINT ( 'NONE',  ( 1.500000000000008438, 22.80000000000002913, -57.83153971412246364 ) ) ;
#15915=ORIENTED_EDGE ( 'NONE', *, *, #94659, .F. ) ;
#15923=CARTESIAN_POINT ( 'NONE',  ( 22.81625015709509441, 31.40387420917330275, -3.824999997268813345 ) ) ;
#15971=CARTESIAN_POINT ( 'NONE',  ( 36.91746824999999887, -11.99521256947793546, -8.224999997268811924 ) ) ;
#15973=CARTESIAN_POINT ( 'NONE',  ( -19.97888994334923751, -34.65319547504298470, -10.00000000000000000 ) ) ;
#15974=CARTESIAN_POINT ( 'NONE',  ( 1.461487595131980566, 7.989588206515827906, -64.16719899660255066 ) ) ;
#15982=CARTESIAN_POINT ( 'NONE',  ( -11.51446144058598975, 9.455153793104305038, -62.12179458070791327 ) ) ;
#15986=EDGE_CURVE ( 'NONE', #140047, #102181, #43573, .T. ) ;
#15997=CARTESIAN_POINT ( 'NONE',  ( -36.54539699253353291, -20.47674586971619703, -19.42837732572457909 ) ) ;
#16045=ORIENTED_EDGE ( 'NONE', *, *, #125126, .T. ) ;
#16118=FACE_OUTER_BOUND ( 'NONE', #138338, .T. ) ;
#16123=CARTESIAN_POINT ( 'NONE',  ( -22.68986043004510833, 20.57406348593920953, -47.49330165217068611 ) ) ;
#16125=CARTESIAN_POINT ( 'NONE',  ( -21.30000000000002203, 0.1123844339352012556, -56.46919128290399215 ) ) ;
#16150=CIRCLE ( 'NONE', #90468, 2.500000000000000000 ) ;
#16157=VERTEX_POINT ( 'NONE', #68107 ) ;
#16174=CARTESIAN_POINT ( 'NONE',  ( -2.662494480112493012, -37.13692398601925504, -32.59999999999999432 ) ) ;
#16228=FACE_OUTER_BOUND ( 'NONE', #160343, .T. ) ;
#16244=PRODUCT_DEFINITION_SHAPE ( 'NONE', 'NONE',  #180876 ) ;
#16254=AXIS2_PLACEMENT_3D ( 'NONE', #86283, #38792, #20613 ) ;
#16262=CARTESIAN_POINT ( 'NONE',  ( -2.577820198429831642E-15, -9.100000000000001421, -61.89430850415821794 ) ) ;
#16289=CYLINDRICAL_SURFACE ( 'NONE', #189030, 21.30000000000002913 ) ;
#16377=ORIENTED_EDGE ( 'NONE', *, *, #36572, .F. ) ;
#16379=FACE_OUTER_BOUND ( 'NONE', #101788, .T. ) ;
#16413=CARTESIAN_POINT ( 'NONE',  ( -4.313351365237979351, -4.313351365237916291, -64.53213882399992940 ) ) ;
#16418=FACE_BOUND ( 'NONE', #144674, .T. ) ;
#16423=CARTESIAN_POINT ( 'NONE',  ( -17.33027132694084571, 17.01743274722957011, -56.78176416808770455 ) ) ;
#16432=CARTESIAN_POINT ( 'NONE',  ( -23.48529157249599919, -32.32473071737750558, -9.699999999999999289 ) ) ;
#16447=CARTESIAN_POINT ( 'NONE',  ( 0.000000000000000000, 0.000000000000000000, -54.21489346206828230 ) ) ;
#16456=CARTESIAN_POINT ( 'NONE',  ( 14.20416113188340823, -35.58439206127390975, -22.81347619871590027 ) ) ;
#16480=ADVANCED_FACE ( 'NONE', ( #161121 ), #22618, .F. ) ;
#16487=CARTESIAN_POINT ( 'NONE',  ( 1.322633123934117361, 14.46694947601600312, -62.26929068799466904 ) ) ;
#16523=DIRECTION ( 'NONE',  ( -0.000000000000000000, -0.000000000000000000, -1.000000000000000000 ) ) ;
#16526=CARTESIAN_POINT ( 'NONE',  ( 7.794582437828440291, -1.499905742985332191, -62.16226466885329671 ) ) ;
#16545=CARTESIAN_POINT ( 'NONE',  ( 0.000000000000000000, -165.0000000000000000, 7.000000000000003553 ) ) ;
#16571=CARTESIAN_POINT ( 'NONE',  ( -19.99604614807126524, -21.49604614807087799, -52.16759353428663104 ) ) ;
#16606=EDGE_LOOP ( 'NONE', ( #172037, #135664, #86664, #56163 ) ) ;
#16621=CARTESIAN_POINT ( 'NONE',  ( -22.83040865997688229, -30.22555755524879828, -21.93998231254863285 ) ) ;
#16644=CARTESIAN_POINT ( 'NONE',  ( 21.02739490616371754, -20.06800196981514262, -49.47723517191376885 ) ) ;
#16652=CARTESIAN_POINT ( 'NONE',  ( 6.874011537017776341, -5.374011537017756801, -64.03675147074802965 ) ) ;
#16680=CARTESIAN_POINT ( 'NONE',  ( 20.47811964340659330, -34.28713832286810259, -21.14919058558335507 ) ) ;
#16720=EDGE_CURVE ( 'NONE', #138331, #1611, #101723, .T. ) ;
#16723=VERTEX_POINT ( 'NONE', #86278 ) ;
#16747=EDGE_CURVE ( 'NONE', #40506, #185763, #94067, .T. ) ;
#16764=DIRECTION ( 'NONE',  ( -0.000000000000000000, 0.000000000000000000, 1.000000000000000000 ) ) ;
#16893=CARTESIAN_POINT ( 'NONE',  ( -8.388830574159379737E-16, -13.70000000000001528, -60.44446360152740283 ) ) ;
#16906=ORIENTED_EDGE ( 'NONE', *, *, #197184, .F. ) ;
#16914=CARTESIAN_POINT ( 'NONE',  ( -11.40812507854754720, -35.11059874428192273, -2.724999997268813257 ) ) ;
#16927=CARTESIAN_POINT ( 'NONE',  ( 5.266531018137392550, 6.873421141834948678, -62.00040165901308598 ) ) ;
#16950=CARTESIAN_POINT ( 'NONE',  ( -6.020228577223754586E-15, 39.95556452105416412, -8.500000000000000000 ) ) ;
#16960=VERTEX_POINT ( 'NONE', #164141 ) ;
#16965=CARTESIAN_POINT ( 'NONE',  ( 3.556970738554033499E-15, -38.81732327939057825, -2.624999997268812724 ) ) ;
#16966=CARTESIAN_POINT ( 'NONE',  ( 1.338834197008474947, 23.50074569744939978, -57.34146676846842894 ) ) ;
#16988=EDGE_CURVE ( 'NONE', #77120, #196218, #25638, .T. ) ;
#16998=ADVANCED_FACE ( 'NONE', ( #72117 ), #225, .T. ) ;
#17032=VERTEX_POINT ( 'NONE', #1215 ) ;
#17038=ORIENTED_EDGE ( 'NONE', *, *, #19616, .F. ) ;
#17061=AXIS2_PLACEMENT_3D ( 'NONE', #29858, #46012, #199707 ) ;
#17113=CARTESIAN_POINT ( 'NONE',  ( -38.00000000000000711, 2.893978650043524126E-14, -25.00000000000000000 ) ) ;
#17117=CARTESIAN_POINT ( 'NONE',  ( -22.78165926218177972, 20.70663425419845893, -47.27781451939566892 ) ) ;
#17155=CARTESIAN_POINT ( 'NONE',  ( -7.405410116723207814, 1.490485923554937697, -62.24175268741322498 ) ) ;
#17243=CARTESIAN_POINT ( 'NONE',  ( 0.000000000000000000, 0.000000000000000000, -25.00000000000000000 ) ) ;
#17252=DIRECTION ( 'NONE',  ( 0.000000000000000000, 0.000000000000000000, 1.000000000000000000 ) ) ;
#17316=CARTESIAN_POINT ( 'NONE',  ( -69.65682714487590488, -71.74905178543390605, -25.00000000000000000 ) ) ;
#17351=EDGE_CURVE ( 'NONE', #69099, #132572, #185724, .T. ) ;
#17368=DIRECTION ( 'NONE',  ( -1.000000000000000000, 0.000000000000000000, 0.000000000000000000 ) ) ;
#17377=CARTESIAN_POINT ( 'NONE',  ( 16.70000000000002061, 0.000000000000000000, -61.34707691135562868 ) ) ;
#17384=CIRCLE ( 'NONE', #120715, 6.100000000000006750 ) ;
#17397=CARTESIAN_POINT ( 'NONE',  ( 0.000000000000000000, 0.000000000000000000, -10.00000000000000000 ) ) ;
#17401=CARTESIAN_POINT ( 'NONE',  ( 4.908066780550757180, -48.27782543269306359, -24.94981842180952469 ) ) ;
#17402=DIRECTION ( 'NONE',  ( 1.000000000000000000, 0.000000000000000000, 0.000000000000000000 ) ) ;
#17408=DIRECTION ( 'NONE',  ( -1.000000000000000000, 0.000000000000000000, 0.000000000000000000 ) ) ;
#17432=EDGE_CURVE ( 'NONE', #66168, #48307, #66202, .T. ) ;
#17433=CARTESIAN_POINT ( 'NONE',  ( -12.73749492396214578, -155.7167183371837496, -15.00000000000000178 ) ) ;
#17447=CARTESIAN_POINT ( 'NONE',  ( 23.65597376186088496, -29.51279439667791138, -21.31698521574967131 ) ) ;
#17465=AXIS2_PLACEMENT_3D ( 'NONE', #16447, #181346, #136801 ) ;
#17473=CARTESIAN_POINT ( 'NONE',  ( 6.938893903907228378E-15, 22.80000000000002913, -65.00100000000003320 ) ) ;
#17474=ORIENTED_EDGE ( 'NONE', *, *, #177434, .F. ) ;
#17478=VERTEX_POINT ( 'NONE', #199438 ) ;
#17513=LINE ( 'NONE', #79171, #40385 ) ;
#17516=CARTESIAN_POINT ( 'NONE',  ( 6.100000000000007638, -0.2002935562469382313, -62.50719930893271226 ) ) ;
#17535=CARTESIAN_POINT ( 'NONE',  ( -38.00000000000000711, 2.893978650043524126E-14, -25.00000000000000000 ) ) ;
#17536=LINE ( 'NONE', #36413, #145438 ) ;
#17563=CARTESIAN_POINT ( 'NONE',  ( -20.90420839357180682, -22.88042607247932025, -50.28910616114573884 ) ) ;
#17617=CARTESIAN_POINT ( 'NONE',  ( -27.29882810768609147, -25.71095057349984714, -18.52182797988006158 ) ) ;
#17639=CARTESIAN_POINT ( 'NONE',  ( 22.72298157751957248, -20.62403296052382728, -47.41336191935017297 ) ) ;
#17645=DIRECTION ( 'NONE',  ( 0.8571673007021135549, 0.000000000000000000, 0.5150380749100520461 ) ) ;
#17667=CARTESIAN_POINT ( 'NONE',  ( 11.40812507854755253, -35.11059874428192273, -6.024999997268814411 ) ) ;
#17677=CARTESIAN_POINT ( 'NONE',  ( 19.65751872600772998, -34.84114385728654639, -25.66966870009445856 ) ) ;
#17727=VECTOR ( 'NONE', #96835, 1000.000000000000000 ) ;
#17731=CARTESIAN_POINT ( 'NONE',  ( 36.91746824999999887, 11.99521256947799053, -10.02499999726881086 ) ) ;
#17739=CARTESIAN_POINT ( 'NONE',  ( -38.00000000000000711, 2.428612866367529932E-14, -2.000000000000000000 ) ) ;
#17757=AXIS2_PLACEMENT_3D ( 'NONE', #99951, #84776, #110396 ) ;
#17856=VECTOR ( 'NONE', #55254, 1000.000000000000000 ) ;
#17897=CARTESIAN_POINT ( 'NONE',  ( -1.359015117358330027, -15.84196527238552754, -59.51370404797111746 ) ) ;
#17967=CARTESIAN_POINT ( 'NONE',  ( 36.91746824999999177, 2.880721459617395097E-14, -2.124999997268813168 ) ) ;
#17968=CARTESIAN_POINT ( 'NONE',  ( -22.96000461283911065, 21.84063423829466544, -49.40985016368630767 ) ) ;
#17991=CARTESIAN_POINT ( 'NONE',  ( -33.88770617167997301, -21.25088722958029663, -25.15219191025231993 ) ) ;
#18014=EDGE_CURVE ( 'NONE', #159131, #19675, #142718, .T. ) ;
#18051=CIRCLE ( 'NONE', #11724, 13.70000000000001528 ) ;
#18119=CARTESIAN_POINT ( 'NONE',  ( -38.00000000000000711, 2.428612866367529932E-14, -10.87499999726881228 ) ) ;
#18121=CARTESIAN_POINT ( 'NONE',  ( -9.443730985155296409, -10.00060863403381006, -60.42334892181182227 ) ) ;
#18142=AXIS2_PLACEMENT_3D ( 'NONE', #86720, #59369, #90699 ) ;
#18169=CARTESIAN_POINT ( 'NONE',  ( -0.4884129450682956897, -31.82351365011402322, -49.22894560581806900 ) ) ;
#18184=AXIS2_PLACEMENT_3D ( 'NONE', #59648, #11189, #72864 ) ;
#18204=FACE_OUTER_BOUND ( 'NONE', #181058, .T. ) ;
#18218=ORIENTED_EDGE ( 'NONE', *, *, #5788, .T. ) ;
#18231=VECTOR ( 'NONE', #64442, 1000.000000000000000 ) ;
#18256=CARTESIAN_POINT ( 'NONE',  ( -14.46726734353920740, 1.322814319813122808, -62.26916108939693828 ) ) ;
#18276=DIRECTION ( 'NONE',  ( 0.9526137857479322069, -0.3041824702427683991, 0.000000000000000000 ) ) ;
#18319=CARTESIAN_POINT ( 'NONE',  ( 37.99999999999999289, 2.428612866367529932E-14, -25.00000000000000000 ) ) ;
#18384=CARTESIAN_POINT ( 'NONE',  ( 0.2219041290406811306, 24.28753333320288021, -54.22462712070620228 ) ) ;
#18407=CARTESIAN_POINT ( 'NONE',  ( 16.67568593663829901, -39.83563513005474732, -20.80532163689324676 ) ) ;
#18428=CARTESIAN_POINT ( 'NONE',  ( -11.74264578624799782, -36.14014761921581709, -9.600000000000001421 ) ) ;
#18437=FACE_OUTER_BOUND ( 'NONE', #72514, .T. ) ;
#18450=CARTESIAN_POINT ( 'NONE',  ( 9.554919064906188808, -36.23455639189494804, -31.31948065624977318 ) ) ;
#18478=CIRCLE ( 'NONE', #128148, 8.000000000000000000 ) ;
#18534=CARTESIAN_POINT ( 'NONE',  ( -4.180825498786520988, -4.459728486673432357, -62.50521485713754544 ) ) ;
#18561=CARTESIAN_POINT ( 'NONE',  ( 10.33027487414777568, 12.20125963778084710, -59.47400725600236626 ) ) ;
#18633=AXIS2_PLACEMENT_3D ( 'NONE', #169071, #103451, #28614 ) ;
#18637=CARTESIAN_POINT ( 'NONE',  ( -38.00000000000000711, 2.428612866367529932E-14, -10.00000000000000000 ) ) ;
#18640=CARTESIAN_POINT ( 'NONE',  ( 3.882848763669480618, 5.183909576824676790, -64.47227361656570110 ) ) ;
#18643=DIRECTION ( 'NONE',  ( -1.000000000000000000, 0.000000000000000000, 0.000000000000000000 ) ) ;
#18662=CARTESIAN_POINT ( 'NONE',  ( -36.91746825000001309, 11.99521256947798342, -6.724999997268813701 ) ) ;
#18672=CARTESIAN_POINT ( 'NONE',  ( 23.38344545171973010, -32.96869167543344048, -17.70766473210208858 ) ) ;
#18711=CARTESIAN_POINT ( 'NONE',  ( 0.000000000000000000, 0.000000000000000000, -18.00000000000000000 ) ) ;
#18723=CARTESIAN_POINT ( 'NONE',  ( -22.81625015709509441, -31.40387420917324590, -2.324999997268813789 ) ) ;
#18724=CARTESIAN_POINT ( 'NONE',  ( -9.687362902255795660, -9.687362902255630459, -60.44446360152740993 ) ) ;
#18759=CARTESIAN_POINT ( 'NONE',  ( 30.74264578624800137, -22.33583958711395212, -1.200000000000000178 ) ) ;
#18779=AXIS2_PLACEMENT_3D ( 'NONE', #186921, #190871, #172724 ) ;
#18786=AXIS2_PLACEMENT_3D ( 'NONE', #179317, #40781, #103455 ) ;
#18841=ORIENTED_EDGE ( 'NONE', *, *, #63306, .T. ) ;
#18890=CARTESIAN_POINT ( 'NONE',  ( -8.388830574159379737E-16, -13.70000000000001528, -60.44446360152740283 ) ) ;
#18896=CARTESIAN_POINT ( 'NONE',  ( 2.019537816779184180E-14, -78.64189009824758614, -24.99999966871768819 ) ) ;
#18904=ORIENTED_EDGE ( 'NONE', *, *, #42100, .F. ) ;
#18907=CYLINDRICAL_SURFACE ( 'NONE', #130279, 31.90000000000003411 ) ;
#18910=CARTESIAN_POINT ( 'NONE',  ( 22.81625015709510151, -31.40387420917324590, -6.424999997268812102 ) ) ;
#18926=AXIS2_PLACEMENT_3D ( 'NONE', #94783, #2777, #3759 ) ;
#18959=CARTESIAN_POINT ( 'NONE',  ( 11.40812507854755253, -35.11059874428192273, -4.524999997268813523 ) ) ;
#18967=CARTESIAN_POINT ( 'NONE',  ( 7.819668024151653185, -36.54656901728082374, -31.88218832179849116 ) ) ;
#19028=VERTEX_POINT ( 'NONE', #16174 ) ;
#19047=DIRECTION ( 'NONE',  ( 0.000000000000000000, 0.000000000000000000, 1.000000000000000000 ) ) ;
#19085=CARTESIAN_POINT ( 'NONE',  ( 1.500000000000211831, 7.503099880506102437, -62.22181180016721669 ) ) ;
#19122=CARTESIAN_POINT ( 'NONE',  ( -23.48529157249600985, 32.32473071737754111, -0.2999999999999999334 ) ) ;
#19125=CARTESIAN_POINT ( 'NONE',  ( -31.88380457335793849, 0.2515199893715405755, -49.15318026754364666 ) ) ;
#19129=CARTESIAN_POINT ( 'NONE',  ( -11.80868324581545714, -11.80868324581525997, -61.34707691135562868 ) ) ;
#19212=CARTESIAN_POINT ( 'NONE',  ( -7.765519415020589733, -39.80263117873666090, -25.57543461820454667 ) ) ;
#19247=CARTESIAN_POINT ( 'NONE',  ( -15.57446157010953591, 1.455575599911040019, -61.81477736546834478 ) ) ;
#19362=CYLINDRICAL_SURFACE ( 'NONE', #88954, 4.000000000000000888 ) ;
#19388=CARTESIAN_POINT ( 'NONE',  ( 17.62203461105333702, -16.12203461105326951, -64.92279855667830191 ) ) ;
#19399=FACE_BOUND ( 'NONE', #90520, .T. ) ;
#19423=CARTESIAN_POINT ( 'NONE',  ( 0.000000000000000000, 0.000000000000000000, -60.44446360152740283 ) ) ;
#19436=CARTESIAN_POINT ( 'NONE',  ( 27.37900830011397346, -26.18142635053362000, -16.57177559434128611 ) ) ;
#19497=DIRECTION ( 'NONE',  ( 6.391086490440865492E-16, 1.000000000000000000, -0.000000000000000000 ) ) ;
#19545=CARTESIAN_POINT ( 'NONE',  ( -38.00000000000000711, -12.34694845685042708, -7.900000000000000355 ) ) ;
#19547=CARTESIAN_POINT ( 'NONE',  ( -20.13069416963696057, -20.86710639515136023, -52.55595668995117364 ) ) ;
#19573=( BOUNDED_SURFACE ( )  B_SPLINE_SURFACE ( 3, 2, ( 
 ( #10504, #194521, #136812 ),
 ( #180370, #86328, #148015 ),
 ( #55993, #25685, #87330 ),
 ( #149016, #72166, #73184 ),
 ( #165183, #41839, #26678 ),
 ( #88318, #58003, #2265 ),
 ( #78105, #91273, #18450 ),
 ( #77122, #123609, #172121 ),
 ( #122628, #47796, #92284 ),
 ( #125617, #154960, #137803 ),
 ( #44810, #30631, #95270 ),
 ( #199487, #152964, #139774 ),
 ( #170131, #153968, #185304 ),
 ( #272, #16456, #168144 ),
 ( #60954, #140776, #138791 ),
 ( #61941, #14463, #29641 ),
 ( #46795, #93275, #45799 ),
 ( #1262, #183329, #62939 ),
 ( #106465, #33607, #108454 ),
 ( #64935, #124619, #63948 ),
 ( #109446, #184318, #107451 ),
 ( #31625, #169126, #76125 ),
 ( #15465, #94272, #186314 ),
 ( #171129, #156953, #32618 ),
 ( #155950, #80101, #17447 ),
 ( #141769, #79103, #187315 ),
 ( #48786, #110440, #3262 ),
 ( #68921, #8251, #65922 ),
 ( #6240, #81084, #67919 ),
 ( #159932, #112431, #51753 ),
 ( #128583, #113414, #144755 ),
 ( #177124, #21419, #34600 ),
 ( #85074, #20414, #66919 ),
 ( #19436, #127595, #191269 ),
 ( #157945, #130583, #98229 ),
 ( #192278, #188296, #174120 ),
 ( #83079, #158925, #126594 ),
 ( #37584, #189294, #146757 ),
 ( #53759, #142762, #173125 ),
 ( #190277, #115433, #38595 ),
 ( #49773, #176113, #96259 ),
 ( #129572, #100251, #52744 ),
 ( #175105, #82064, #114412 ),
 ( #143757, #111438, #161932 ) ),
 .UNSPECIFIED., .F., .F., .T. ) 
 B_SPLINE_SURFACE_WITH_KNOTS ( ( 4, 2, 2, 2, 2, 2, 2, 2, 2, 2, 2, 2, 2, 2, 2, 2, 2, 2, 2, 2, 2, 4 ),
 ( 3, 3 ),
 ( 0.1334715276261013994, 0.1400397817209069751, 0.1416818452446083620, 0.1433239087683097490, 0.1466080358157125230, 0.1498921628631152969, 0.1531762899105180986, 0.1564604169579209003, 0.1597445440053236743, 0.1630286710527264482, 0.1646707345764278352, 0.1663127981001292222, 0.1679548616238306091, 0.1695969251475319961, 0.1712389886712333831, 0.1720600204330841043, 0.1728810521949347978, 0.1745231157186362125, 0.1761651792423375995, 0.1794493062897403735, 0.1827334333371431474, 0.1860175603845459213 ),
 ( 0.000000000000000000, 1.000000000000000000 ),
 .UNSPECIFIED. ) 
 GEOMETRIC_REPRESENTATION_ITEM ( )  RATIONAL_B_SPLINE_SURFACE ( (
 ( 1.000000000000000000, 0.7745966692414831822, 1.000000000000000000),
 ( 1.000000000000000000, 0.7873173169473692834, 1.000000000000000000),
 ( 1.000000000000000000, 0.8012080269095258611, 1.000000000000000000),
 ( 1.000000000000000000, 0.8197272276932416890, 1.000000000000000000),
 ( 1.000000000000000000, 0.8234885421913027415, 1.000000000000000000),
 ( 1.000000000000000000, 0.8311157573375616003, 1.000000000000000000),
 ( 1.000000000000000000, 0.8349728938257290345, 1.000000000000000000),
 ( 1.000000000000000000, 0.8465302108189953767, 1.000000000000000000),
 ( 1.000000000000000000, 0.8542644918355704053, 1.000000000000000000),
 ( 1.000000000000000000, 0.8696747091109493510, 1.000000000000000000),
 ( 1.000000000000000000, 0.8773507960692895624, 1.000000000000000000),
 ( 1.000000000000000000, 0.8925002889087803037, 1.000000000000000000),
 ( 1.000000000000000000, 0.8999891582782625354, 1.000000000000000000),
 ( 1.000000000000000000, 0.9145203485640004404, 1.000000000000000000),
 ( 1.000000000000000000, 0.9215166741119604765, 1.000000000000000000),
 ( 1.000000000000000000, 0.9348196634156800133, 1.000000000000000000),
 ( 1.000000000000000000, 0.9411264847296241243, 1.000000000000000000),
 ( 1.000000000000000000, 0.9528821887672445090, 1.000000000000000000),
 ( 1.000000000000000000, 0.9583320463343323325, 1.000000000000000000),
 ( 1.000000000000000000, 0.9657141226242917931, 1.000000000000000000),
 ( 1.000000000000000000, 0.9680424144921332408, 1.000000000000000000),
 ( 1.000000000000000000, 0.9724014971077671321, 1.000000000000000000),
 ( 1.000000000000000000, 0.9744334801158450743, 1.000000000000000000),
 ( 1.000000000000000000, 0.9781204877085362126, 1.000000000000000000),
 ( 1.000000000000000000, 0.9797809101335807069, 1.000000000000000000),
 ( 1.000000000000000000, 0.9826818083352882871, 1.000000000000000000),
 ( 1.000000000000000000, 0.9839230189806438265, 1.000000000000000000),
 ( 1.000000000000000000, 0.9859013487405716702, 1.000000000000000000),
 ( 1.000000000000000000, 0.9866146582094302842, 1.000000000000000000),
 ( 1.000000000000000000, 0.9872250220265940124, 1.000000000000000000),
 ( 1.000000000000000000, 0.9873522598263612116, 1.000000000000000000),
 ( 1.000000000000000000, 0.9874472609175478643, 1.000000000000000000),
 ( 1.000000000000000000, 0.9874138636738800656, 1.000000000000000000),
 ( 1.000000000000000000, 0.9870735186574125519, 1.000000000000000000),
 ( 1.000000000000000000, 0.9865315217160652850, 1.000000000000000000),
 ( 1.000000000000000000, 0.9848873008857785827, 1.000000000000000000),
 ( 1.000000000000000000, 0.9837743821442975767, 1.000000000000000000),
 ( 1.000000000000000000, 0.9797976954002131089, 1.000000000000000000),
 ( 1.000000000000000000, 0.9763000371664848354, 1.000000000000000000),
 ( 1.000000000000000000, 0.9680363503266696812, 1.000000000000000000),
 ( 1.000000000000000000, 0.9632464763793496809, 1.000000000000000000),
 ( 1.000000000000000000, 0.9526889542241597786, 1.000000000000000000),
 ( 1.000000000000000000, 0.9469283804590763465, 1.000000000000000000),
 ( 1.000000000000000000, 0.9407878411039235500, 1.000000000000000000) ) ) 
 REPRESENTATION_ITEM ( '' )  SURFACE ( )  );
#19588=ORIENTED_EDGE ( 'NONE', *, *, #32449, .F. ) ;
#19599=CARTESIAN_POINT ( 'NONE',  ( -30.69486229629621832, -23.16037512311192614, -17.06287707313649449 ) ) ;
#19616=EDGE_CURVE ( 'NONE', #193677, #25217, #35308, .T. ) ;
#19624=CARTESIAN_POINT ( 'NONE',  ( 5.563988007711757611, 6.875025434611794495, -64.01045944195827531 ) ) ;
#19644=ORIENTED_EDGE ( 'NONE', *, *, #166964, .T. ) ;
#19646=CARTESIAN_POINT ( 'NONE',  ( -22.81625015709510507, 31.40387420917330275, -2.924999997268813434 ) ) ;
#19654=FACE_OUTER_BOUND ( 'NONE', #166003, .T. ) ;
#19656=CARTESIAN_POINT ( 'NONE',  ( 22.23580286100631653, -34.17069428430818334, -18.13567467416763179 ) ) ;
#19675=VERTEX_POINT ( 'NONE', #144469 ) ;
#19694=DIRECTION ( 'NONE',  ( 1.000000000000000000, 0.000000000000000000, 0.000000000000000000 ) ) ;
#19706=CARTESIAN_POINT ( 'NONE',  ( 29.86685920354754842, -21.69954338932559068, -1.824999997268813345 ) ) ;
#19726=CARTESIAN_POINT ( 'NONE',  ( -0.9271017399331331621, -6.404328268737251584, -64.47359807031668311 ) ) ;
#19740=CARTESIAN_POINT ( 'NONE',  ( 31.62105185743274660, -0.8768460684519197024, -49.48175094143203268 ) ) ;
#19810=EDGE_CURVE ( 'NONE', #56239, #23346, #185257, .T. ) ;
#19818=VERTEX_POINT ( 'NONE', #5953 ) ;
#19866=CARTESIAN_POINT ( 'NONE',  ( 0.1986149132935111361, 9.090066029660778923, -61.89635500127618428 ) ) ;
#19869=DIRECTION ( 'NONE',  ( -0.000000000000000000, -0.000000000000000000, -1.000000000000000000 ) ) ;
#19881=ORIENTED_EDGE ( 'NONE', *, *, #199458, .T. ) ;
#19889=CARTESIAN_POINT ( 'NONE',  ( 11.40812507854755253, -35.11059874428192273, -6.524999997268813523 ) ) ;
#19897=CARTESIAN_POINT ( 'NONE',  ( -2.500000000000000000, -165.0000000000000000, 12.00000000000000355 ) ) ;
#19936=CARTESIAN_POINT ( 'NONE',  ( -22.81625015709509441, -31.40387420917324590, -4.824999997268813345 ) ) ;
#19937=EDGE_CURVE ( 'NONE', #152430, #12139, #72114, .T. ) ;
#19948=CARTESIAN_POINT ( 'NONE',  ( 15.67660317299531414, 17.56609036915066469, -57.33766855040059340 ) ) ;
#20103=CARTESIAN_POINT ( 'NONE',  ( -31.62105185743270397, 0.8768460684521839354, -49.48175094143205399 ) ) ;
#20119=CARTESIAN_POINT ( 'NONE',  ( 29.23421922662630834, -26.92455035691565257, -20.45761606001068955 ) ) ;
#20121=CARTESIAN_POINT ( 'NONE',  ( 11.74264578624800315, -36.14014761921581709, -3.149999994537626247 ) ) ;
#20131=CYLINDRICAL_SURFACE ( 'NONE', #134998, 9.100000000000001421 ) ;
#20155=EDGE_LOOP ( 'NONE', ( #67839, #81108 ) ) ;
#20169=CARTESIAN_POINT ( 'NONE',  ( 0.000000000000000000, -105.0000000000000000, 7.000000000000003553 ) ) ;
#20176=CARTESIAN_POINT ( 'NONE',  ( -0.9086318102904998861, -31.61347055016711849, -46.06737158113915598 ) ) ;
#20187=CARTESIAN_POINT ( 'NONE',  ( -19.65751872600893080, -34.84114385728561558, -25.66966870010219637 ) ) ;
#20199=CARTESIAN_POINT ( 'NONE',  ( 11.66256017358946728, 11.95480631804125515, -61.34707691135565710 ) ) ;
#20220=CARTESIAN_POINT ( 'NONE',  ( -1.499905742985305324, -7.794582437828434962, -62.16226466885326118 ) ) ;
#20254=CYLINDRICAL_SURFACE ( 'NONE', #67796, 1.499999999999997780 ) ;
#20314=DIRECTION ( 'NONE',  ( -1.000000000000000000, 6.391086490440866478E-16, 0.000000000000000000 ) ) ;
#20333=EDGE_LOOP ( 'NONE', ( #55783, #66471, #28838, #7002, #127753, #65696, #36728, #43976, #135193 ) ) ;
#20363=CIRCLE ( 'NONE', #75225, 10.00000000000000000 ) ;
#20402=DIRECTION ( 'NONE',  ( 1.000000000000000000, 0.000000000000000000, 0.000000000000000000 ) ) ;
#20414=CARTESIAN_POINT ( 'NONE',  ( 26.32780677389235890, -26.67379781540241268, -18.43298970368203626 ) ) ;
#20454=CARTESIAN_POINT ( 'NONE',  ( -21.49604614807126524, -21.49604614807088154, -64.92279855667830191 ) ) ;
#20458=EDGE_CURVE ( 'NONE', #101425, #178697, #37334, .T. ) ;
#20485=ADVANCED_FACE ( 'NONE', ( #19654 ), #167636, .F. ) ;
#20538=CIRCLE ( 'NONE', #159380, 24.30000000000003268 ) ;
#20579=ORIENTED_EDGE ( 'NONE', *, *, #69149, .F. ) ;
#20581=CARTESIAN_POINT ( 'NONE',  ( -26.32780677389376578, -26.67379781540345718, -18.43298970368158152 ) ) ;
#20596=ORIENTED_EDGE ( 'NONE', *, *, #2366, .T. ) ;
#20611=CARTESIAN_POINT ( 'NONE',  ( 0.000000000000000000, -165.0000000000000000, -23.00000000000000000 ) ) ;
#20613=DIRECTION ( 'NONE',  ( -1.000000000000000000, 0.000000000000000000, 0.000000000000000000 ) ) ;
#20628=ORIENTED_EDGE ( 'NONE', *, *, #156887, .F. ) ;
#20630=CARTESIAN_POINT ( 'NONE',  ( 36.91746824999999887, 11.99521256947799053, -5.524999997268812635 ) ) ;
#20640=CARTESIAN_POINT ( 'NONE',  ( 21.50179914127970093, -34.93963825066541062, -18.44273973154308521 ) ) ;
#20677=CARTESIAN_POINT ( 'NONE',  ( -38.00000000000000711, 2.893978650043524126E-14, -25.00000000000000000 ) ) ;
#20684=VECTOR ( 'NONE', #119233, 1000.000000000000000 ) ;
#20687=FACE_OUTER_BOUND ( 'NONE', #166875, .T. ) ;
#20690=CARTESIAN_POINT ( 'NONE',  ( -11.40812507854755609, 35.11059874428196537, -1.024999997268813301 ) ) ;
#20704=ORIENTED_EDGE ( 'NONE', *, *, #172898, .F. ) ;
#20707=VECTOR ( 'NONE', #52230, 1000.000000000000000 ) ;
#20757=ORIENTED_EDGE ( 'NONE', *, *, #165015, .T. ) ;
#20775=AXIS2_PLACEMENT_3D ( 'NONE', #17473, #52769, #3288 ) ;
#20805=ORIENTED_EDGE ( 'NONE', *, *, #93266, .F. ) ;
#20816=EDGE_CURVE ( 'NONE', #189816, #194525, #82036, .T. ) ;
#20823=ORIENTED_EDGE ( 'NONE', *, *, #158246, .T. ) ;
#20836=CARTESIAN_POINT ( 'NONE',  ( -38.00000000000004263, -12.34694845685037023, -5.899999999999999467 ) ) ;
#20839=CARTESIAN_POINT ( 'NONE',  ( 20.25987216150956272, 20.63676584477893172, -49.65115959356506892 ) ) ;
#20851=EDGE_CURVE ( 'NONE', #66168, #27708, #136298, .T. ) ;
#20866=CARTESIAN_POINT ( 'NONE',  ( 3.556970738554034288E-15, -38.81732327939057114, -2.124999997268813168 ) ) ;
#20880=CARTESIAN_POINT ( 'NONE',  ( 22.81625015709510151, -31.40387420917324590, -10.42499999726881477 ) ) ;
#20910=AXIS2_PLACEMENT_3D ( 'NONE', #157148, #48977, #190475 ) ;
#20927=CARTESIAN_POINT ( 'NONE',  ( 22.81625015709510151, -31.40387420917324590, -4.424999997268812990 ) ) ;
#20928=CARTESIAN_POINT ( 'NONE',  ( -22.78074831271784362, 20.70421334297363458, -50.54281738342967856 ) ) ;
#21017=CIRCLE ( 'NONE', #79043, 12.50000000000000000 ) ;
#21018=CARTESIAN_POINT ( 'NONE',  ( 11.74264578624800315, -36.14014761921581709, -11.14999999453762669 ) ) ;
#21024=VECTOR ( 'NONE', #159887, 1000.000000000000114 ) ;
#21039=DIRECTION ( 'NONE',  ( -0.000000000000000000, -0.000000000000000000, 1.000000000000000000 ) ) ;
#21057=DIRECTION ( 'NONE',  ( 1.000000000000000000, 0.000000000000000000, 0.000000000000000000 ) ) ;
#21097=B_SPLINE_CURVE_WITH_KNOTS ( 'NONE', 3,
 ( #172051, #96193, #18384, #51688, #158857, #141704, #84010, #66852, #188229, #21355, #143687, #145688 ),
 .UNSPECIFIED., .F., .F.,
 ( 4, 2, 2, 2, 2, 4 ),
 ( 1.967889508672852735E-07, 0.0003319461778748304345, 0.0006636955667987935086, 0.0009954449557227568537, 0.001327194344646719874, 0.002654191900342570219 ),
 .UNSPECIFIED. ) ;
#21101=AXIS2_PLACEMENT_3D ( 'NONE', #122539, #10416, #184230 ) ;
#21129=DIRECTION ( 'NONE',  ( -0.000000000000000000, -0.000000000000000000, -1.000000000000000000 ) ) ;
#21132=CARTESIAN_POINT ( 'NONE',  ( 23.87356034986291320, -29.32389248808944160, -21.14071813158713908 ) ) ;
#21189=CARTESIAN_POINT ( 'NONE',  ( -12.04662589228467873, -37.70593178235914422, -30.82293284779907339 ) ) ;
#21190=ORIENTED_EDGE ( 'NONE', *, *, #82044, .F. ) ;
#21202=ORIENTED_EDGE ( 'NONE', *, *, #144540, .F. ) ;
#21213=CARTESIAN_POINT ( 'NONE',  ( -23.48529157249599919, -32.32473071737749848, -9.449999994537623849 ) ) ;
#21240=AXIS2_PLACEMENT_3D ( 'NONE', #75249, #60075, #150124 ) ;
#21249=DIRECTION ( 'NONE',  ( -0.1178549842436482503, 0.9930308165857338887, -1.226674847569999905E-16 ) ) ;
#21323=DIRECTION ( 'NONE',  ( -1.000000000000000000, 3.552713678800500929E-15, 0.000000000000000000 ) ) ;
#21355=CARTESIAN_POINT ( 'NONE',  ( 1.376754478911074830, 23.51071581304989522, -54.82534132429363183 ) ) ;
#21419=CARTESIAN_POINT ( 'NONE',  ( 26.12775673971824375, -26.86876869530867751, -18.42961048235288857 ) ) ;
#21485=EDGE_CURVE ( 'NONE', #193461, #85102, #172879, .T. ) ;
#21525=CYLINDRICAL_SURFACE ( 'NONE', #82564, 1.499999999999997780 ) ;
#21575=ORIENTED_EDGE ( 'NONE', *, *, #59660, .F. ) ;
#21583=VERTEX_POINT ( 'NONE', #140549 ) ;
#21594=ADVANCED_FACE ( 'NONE', ( #77879 ), #139546, .F. ) ;
#21603=CYLINDRICAL_SURFACE ( 'NONE', #24553, 214.0437394197456342 ) ;
#21609=CARTESIAN_POINT ( 'NONE',  ( -30.74964850363292257, 1.467638476639392398, -47.27948696604330081 ) ) ;
#21613=CARTESIAN_POINT ( 'NONE',  ( -30.74264578624800492, -22.33583958711396278, -7.549999994537627934 ) ) ;
#21637=CARTESIAN_POINT ( 'NONE',  ( -29.86685920354755197, -21.69954338932560134, -4.424999997268812990 ) ) ;
#21648=CARTESIAN_POINT ( 'NONE',  ( 31.83877234781633803, -24.10177343596294364, -22.51708424454470148 ) ) ;
#21694=EDGE_LOOP ( 'NONE', ( #116199, #160088, #175349, #73679 ) ) ;
#21699=CARTESIAN_POINT ( 'NONE',  ( 11.40812507854755253, -35.11059874428192273, -2.024999997268813079 ) ) ;
#21700=LINE ( 'NONE', #98516, #128135 ) ;
#21734=CARTESIAN_POINT ( 'NONE',  ( 29.53952216915894269, -1.232294487434747010, -51.94279119241699760 ) ) ;
#21738=CARTESIAN_POINT ( 'NONE',  ( 11.30153831258473573, -180.0000000000000284, -15.00000000000000178 ) ) ;
#21762=EDGE_CURVE ( 'NONE', #85102, #76043, #30864, .T. ) ;
#21766=ORIENTED_EDGE ( 'NONE', *, *, #23834, .T. ) ;
#21778=DIRECTION ( 'NONE',  ( -1.000000000000000000, 0.000000000000000000, 0.000000000000000000 ) ) ;
#21807=AXIS2_PLACEMENT_3D ( 'NONE', #27386, #25398, #119387 ) ;
#21863=CARTESIAN_POINT ( 'NONE',  ( 0.9208130691986635696, 8.788201535090163219, -61.95848299590669939 ) ) ;
#21866=CARTESIAN_POINT ( 'NONE',  ( -36.91746825000000598, 2.428612866367529932E-14, -10.87499999726881228 ) ) ;
#21872=DIRECTION ( 'NONE',  ( 1.000000000000000000, 0.000000000000000000, 0.000000000000000000 ) ) ;
#21874=CARTESIAN_POINT ( 'NONE',  ( 29.86685920354754487, 21.69954338932564752, -5.424999997268813878 ) ) ;
#21883=CARTESIAN_POINT ( 'NONE',  ( -31.88446454451164414, -20.67411064994756487, -24.22501891791619855 ) ) ;
#21935=CARTESIAN_POINT ( 'NONE',  ( -22.84806810306151093, 22.15679140170787065, -49.22928680315004613 ) ) ;
#22024=DIRECTION ( 'NONE',  ( 1.000000000000000000, 0.000000000000000000, 0.000000000000000000 ) ) ;
#22064=ORIENTED_EDGE ( 'NONE', *, *, #48766, .T. ) ;
#22099=CARTESIAN_POINT ( 'NONE',  ( 30.74264578624799782, 22.33583958711400541, -0.7999999999999999334 ) ) ;
#22107=DIRECTION ( 'NONE',  ( 1.000000000000000000, 0.000000000000000000, 0.000000000000000000 ) ) ;
#22120=CARTESIAN_POINT ( 'NONE',  ( 2.802625768539491968, -39.09149893265183806, -33.00000000000000000 ) ) ;
#22132=CARTESIAN_POINT ( 'NONE',  ( 0.000000000000000000, 0.000000000000000000, -64.92279855667830191 ) ) ;
#22136=CARTESIAN_POINT ( 'NONE',  ( 30.51643230682437036, -22.56685799121280311, -22.94790682118908975 ) ) ;
#22171=CARTESIAN_POINT ( 'NONE',  ( -0.7207009035786708928, -24.11964846217544789, -56.90195918390939767 ) ) ;
#22185=VERTEX_POINT ( 'NONE', #15973 ) ;
#22191=CARTESIAN_POINT ( 'NONE',  ( -16.25089620724270745, -36.76456463896731464, -23.32760966624081078 ) ) ;
#22208=DIRECTION ( 'NONE',  ( 0.000000000000000000, 0.000000000000000000, 1.000000000000000000 ) ) ;
#22219=PLANE ( 'NONE',  #26466 ) ;
#22303=ORIENTED_EDGE ( 'NONE', *, *, #38861, .T. ) ;
#22321=AXIS2_PLACEMENT_3D ( 'NONE', #9968, #86790, #55456 ) ;
#22341=VERTEX_POINT ( 'NONE', #185824 ) ;
#22348=DIRECTION ( 'NONE',  ( 1.000000000000000000, 0.000000000000000000, 0.000000000000000000 ) ) ;
#22386=CARTESIAN_POINT ( 'NONE',  ( 30.74264578624800137, -22.33583958711395212, -4.949999994537626513 ) ) ;
#22392=ORIENTED_EDGE ( 'NONE', *, *, #193896, .T. ) ;
#22394=CARTESIAN_POINT ( 'NONE',  ( -14.46985881644522642, 1.324169127979245797, -60.11284999819415020 ) ) ;
#22401=ORIENTED_EDGE ( 'NONE', *, *, #129491, .F. ) ;
#22413=VERTEX_POINT ( 'NONE', #44328 ) ;
#22429=ORIENTED_EDGE ( 'NONE', *, *, #37807, .F. ) ;
#22450=CARTESIAN_POINT ( 'NONE',  ( 11.30153831258470731, -190.0000000000000000, 0.000000000000000000 ) ) ;
#22535=CARTESIAN_POINT ( 'NONE',  ( 11.30153831258469843, -180.0000000000000000, -15.00000000000000178 ) ) ;
#22546=ADVANCED_FACE ( 'NONE', ( #106971 ), #154480, .T. ) ;
#22581=ORIENTED_EDGE ( 'NONE', *, *, #23142, .F. ) ;
#22607=ORIENTED_EDGE ( 'NONE', *, *, #187510, .T. ) ;
#22615=CARTESIAN_POINT ( 'NONE',  ( -31.05479031690789427, 1.359215367441364730, -46.85916094508149143 ) ) ;
#22618=CYLINDRICAL_SURFACE ( 'NONE', #188909, 2.500000000000000000 ) ;
#22623=CARTESIAN_POINT ( 'NONE',  ( 33.50392338572245166, -21.85172282306471203, -24.09813222787957443 ) ) ;
#22632=AXIS2_PLACEMENT_3D ( 'NONE', #76957, #61778, #151828 ) ;
#22640=CARTESIAN_POINT ( 'NONE',  ( 11.40812507854754365, 35.11059874428196537, -9.224999997268813701 ) ) ;
#22658=FACE_OUTER_BOUND ( 'NONE', #101157, .T. ) ;
#22663=ORIENTED_EDGE ( 'NONE', *, *, #120340, .F. ) ;
#22702=CARTESIAN_POINT ( 'NONE',  ( 29.86685920354754842, -21.69954338932559068, -3.824999997268813345 ) ) ;
#22736=CARTESIAN_POINT ( 'NONE',  ( 31.78116016545943268, -0.5954834035867749842, -49.28208245900466977 ) ) ;
#22784=VECTOR ( 'NONE', #55026, 1000.000000000000000 ) ;
#22834=VERTEX_POINT ( 'NONE', #61463 ) ;
#22881=ORIENTED_EDGE ( 'NONE', *, *, #199123, .F. ) ;
#22932=CARTESIAN_POINT ( 'NONE',  ( 29.03295818733085198, -0.6278704076485333019, -49.50940399778504286 ) ) ;
#22985=EDGE_CURVE ( 'NONE', #154964, #58211, #94556, .T. ) ;
#23007=EDGE_LOOP ( 'NONE', ( #10202, #34067, #25210, #125161, #73095 ) ) ;
#23022=ADVANCED_FACE ( 'NONE', ( #108966 ), #163337, .F. ) ;
#23026=CARTESIAN_POINT ( 'NONE',  ( -22.55670631985092456, 22.55670631985084995, -65.00100000000003320 ) ) ;
#23064=CARTESIAN_POINT ( 'NONE',  ( 6.100000000000006750, -2.167155344068307965E-14, -64.92279855667830191 ) ) ;
#23085=CARTESIAN_POINT ( 'NONE',  ( 12.24802307403562907, -10.59837847217739082, -61.57437130795283053 ) ) ;
#23103=CARTESIAN_POINT ( 'NONE',  ( 17.62203461105334767, -15.97121552610937911, -54.63804455921930270 ) ) ;
#23118=DIRECTION ( 'NONE',  ( 0.000000000000000000, 0.000000000000000000, -1.000000000000000000 ) ) ;
#23122=CARTESIAN_POINT ( 'NONE',  ( -38.00000000000001421, -12.34694845685042708, -5.649999994537625803 ) ) ;
#23139=CARTESIAN_POINT ( 'NONE',  ( -0.1280799071097934450, -28.90000000000004476, -52.65483682830182488 ) ) ;
#23142=EDGE_CURVE ( 'NONE', #15137, #42057, #175583, .T. ) ;
#23183=CARTESIAN_POINT ( 'NONE',  ( -69.65682714487590488, -71.74905178543390605, -15.00000000000000178 ) ) ;
#23197=CARTESIAN_POINT ( 'NONE',  ( -18.40487137061491296, -35.48337831123046726, -26.72115582344491358 ) ) ;
#23209=DIRECTION ( 'NONE',  ( 0.000000000000000000, 0.000000000000000000, 1.000000000000000000 ) ) ;
#23224=FACE_OUTER_BOUND ( 'NONE', #117136, .T. ) ;
#23267=DIRECTION ( 'NONE',  ( -0.000000000000000000, -0.000000000000000000, 1.000000000000000000 ) ) ;
#23346=VERTEX_POINT ( 'NONE', #102034 ) ;
#23376=CARTESIAN_POINT ( 'NONE',  ( 22.15679140170794881, 22.84806810306143632, -49.22928680315006034 ) ) ;
#23380=CARTESIAN_POINT ( 'NONE',  ( -11.74264578624800670, 36.14014761921585972, -4.400000000000000355 ) ) ;
#23394=CARTESIAN_POINT ( 'NONE',  ( -16.16661445520354334, 1.151164073136760946, -59.37042179516131313 ) ) ;
#23423=DIRECTION ( 'NONE',  ( -0.000000000000000000, -0.000000000000000000, -1.000000000000000000 ) ) ;
#23427=CARTESIAN_POINT ( 'NONE',  ( 0.000000000000000000, 0.000000000000000000, -18.00000000000000000 ) ) ;
#23454=DIRECTION ( 'NONE',  ( -1.000000000000000000, 0.000000000000000000, 0.000000000000000000 ) ) ;
#23486=CARTESIAN_POINT ( 'NONE',  ( 69.65682714487590488, -71.74905178543389184, -25.00000000000000000 ) ) ;
#23537=CARTESIAN_POINT ( 'NONE',  ( 11.80868324581537543, 11.80868324581533990, -59.13370768023891344 ) ) ;
#23585=DIRECTION ( 'NONE',  ( -0.000000000000000000, 0.000000000000000000, 1.000000000000000000 ) ) ;
#23592=EDGE_CURVE ( 'NONE', #192734, #116714, #88935, .T. ) ;
#23595=CARTESIAN_POINT ( 'NONE',  ( 1.274273735257150042, 29.60376251271834747, -51.87022419674244844 ) ) ;
#23613=FACE_OUTER_BOUND ( 'NONE', #7153, .T. ) ;
#23623=DIRECTION ( 'NONE',  ( 1.000000000000000000, 0.000000000000000000, 0.000000000000000000 ) ) ;
#23625=CARTESIAN_POINT ( 'NONE',  ( 33.56007109372392705, -21.76539027157619088, -24.27853470289443294 ) ) ;
#23641=CARTESIAN_POINT ( 'NONE',  ( 23.48529157249600630, -32.32473071737749137, -1.299999999999999822 ) ) ;
#23646=CARTESIAN_POINT ( 'NONE',  ( 1.456047670377071501, 15.57251747167111056, -59.63216870564059491 ) ) ;
#23657=AXIS2_PLACEMENT_3D ( 'NONE', #65046, #189403, #80209 ) ;
#23664=ORIENTED_EDGE ( 'NONE', *, *, #67401, .F. ) ;
#23679=DIRECTION ( 'NONE',  ( -0.3041824702427711191, -0.9526137857479313187, 0.000000000000000000 ) ) ;
#23702=CARTESIAN_POINT ( 'NONE',  ( 29.86685920354754842, -21.69954338932559068, -9.824999997268813345 ) ) ;
#23707=CARTESIAN_POINT ( 'NONE',  ( 4.419688410474993390, -4.207014320000904917, -64.53213882399992940 ) ) ;
#23733=CARTESIAN_POINT ( 'NONE',  ( 69.65682714487590488, -71.74905178543389184, -15.00000000000000178 ) ) ;
#23760=EDGE_CURVE ( 'NONE', #121632, #74887, #117230, .T. ) ;
#23763=FACE_OUTER_BOUND ( 'NONE', #185221, .T. ) ;
#23810=AXIS2_PLACEMENT_3D ( 'NONE', #124828, #140985, #171338 ) ;
#23834=EDGE_CURVE ( 'NONE', #41521, #36107, #20363, .T. ) ;
#23839=ORIENTED_EDGE ( 'NONE', *, *, #16988, .T. ) ;
#23857=CARTESIAN_POINT ( 'NONE',  ( -9.248023074035629065, -10.74802307403544077, -62.40259441833023857 ) ) ;
#23866=CARTESIAN_POINT ( 'NONE',  ( -2.577820198429831642E-15, -9.100000000000001421, -64.92279855667830191 ) ) ;
#23877=CARTESIAN_POINT ( 'NONE',  ( 22.81625015709509441, 31.40387420917330275, -3.324999997268812901 ) ) ;
#23935=DIRECTION ( 'NONE',  ( -0.000000000000000000, -0.000000000000000000, 1.000000000000000000 ) ) ;
#23953=VERTEX_POINT ( 'NONE', #55213 ) ;
#24020=ADVANCED_FACE ( 'NONE', ( #132056, #149233 ), #10724, .F. ) ;
#24056=VECTOR ( 'NONE', #152570, 1000.000000000000000 ) ;
#24067=CARTESIAN_POINT ( 'NONE',  ( -15.20000000000001883, 1.574768255752702759E-13, -64.92279855667830191 ) ) ;
#24079=VECTOR ( 'NONE', #11583, 1000.000000000000000 ) ;
#24091=( GEOMETRIC_REPRESENTATION_CONTEXT ( 3 ) GLOBAL_UNCERTAINTY_ASSIGNED_CONTEXT ( ( #114627 ) ) GLOBAL_UNIT_ASSIGNED_CONTEXT ( ( #101239, #86084, #176109 ) ) REPRESENTATION_CONTEXT ( 'NONE', 'WORKASPACE' ) );
#24108=DIRECTION ( 'NONE',  ( 0.000000000000000000, 0.000000000000000000, -1.000000000000000000 ) ) ;
#24120=EDGE_LOOP ( 'NONE', ( #125826, #149302, #22429, #55672 ) ) ;
#24124=VERTEX_POINT ( 'NONE', #168362 ) ;
#24127=CARTESIAN_POINT ( 'NONE',  ( 25.13006352617149375, -30.86725525062045605, -20.93759803324961055 ) ) ;
#24130=EDGE_CURVE ( 'NONE', #177464, #45827, #93493, .T. ) ;
#24131=CARTESIAN_POINT ( 'NONE',  ( -30.74264578624800492, -22.33583958711396278, -5.549999994537627046 ) ) ;
#24140=FACE_OUTER_BOUND ( 'NONE', #196057, .T. ) ;
#24144=LINE ( 'NONE', #177826, #141302 ) ;
#24150=CARTESIAN_POINT ( 'NONE',  ( -0.2552802045322777325, -28.91687668646900988, -52.63629878241253834 ) ) ;
#24162=CARTESIAN_POINT ( 'NONE',  ( 16.12203461105333702, -16.12203461105326951, -64.92279855667830191 ) ) ;
#24183=CARTESIAN_POINT ( 'NONE',  ( 22.81625015709509441, 31.40387420917330275, -5.824999997268813345 ) ) ;
#24193=DIRECTION ( 'NONE',  ( 1.000000000000000000, 0.000000000000000000, 0.000000000000000000 ) ) ;
#24197=CARTESIAN_POINT ( 'NONE',  ( 37.99999999999999289, 2.428612866367529932E-14, -15.00000000000000000 ) ) ;
#24205=CARTESIAN_POINT ( 'NONE',  ( -24.03200911576545096, -31.81637637394599238, -21.77892875005238693 ) ) ;
#24206=ORIENTED_EDGE ( 'NONE', *, *, #48766, .F. ) ;
#24216=CARTESIAN_POINT ( 'NONE',  ( 11.11254985580166910, 12.21717160642876543, -61.43205129781978258 ) ) ;
#24218=AXIS2_PLACEMENT_3D ( 'NONE', #145200, #176565, #6683 ) ;
#24233=DIRECTION ( 'NONE',  ( 0.9974398506828144884, 0.07151044867601406840, -0.000000000000000000 ) ) ;
#24243=DIRECTION ( 'NONE',  ( 0.000000000000000000, 0.000000000000000000, -1.000000000000000000 ) ) ;
#24260=VECTOR ( 'NONE', #39292, 1000.000000000000000 ) ;
#24276=FACE_OUTER_BOUND ( 'NONE', #146520, .T. ) ;
#24296=ADVANCED_FACE ( 'NONE', ( #123823 ), #59188, .F. ) ;
#24318=DIRECTION ( 'NONE',  ( -1.000000000000000000, 0.000000000000000000, 0.000000000000000000 ) ) ;
#24356=ORIENTED_EDGE ( 'NONE', *, *, #146444, .T. ) ;
#24359=FACE_OUTER_BOUND ( 'NONE', #107478, .T. ) ;
#24368=AXIS2_PLACEMENT_3D ( 'NONE', #112720, #4530, #198044 ) ;
#24378=ORIENTED_EDGE ( 'NONE', *, *, #107016, .T. ) ;
#24388=CARTESIAN_POINT ( 'NONE',  ( -3.573655867282028392E-15, -180.0000000000000000, -23.00000000000000000 ) ) ;
#24467=ORIENTED_EDGE ( 'NONE', *, *, #177460, .T. ) ;
#24502=ADVANCED_FACE ( 'NONE', ( #154189 ), #136047, .F. ) ;
#24503=CARTESIAN_POINT ( 'NONE',  ( 0.000000000000000000, 0.000000000000000000, -33.00000000000000000 ) ) ;
#24508=B_SPLINE_CURVE_WITH_KNOTS ( 'NONE', 3,
 ( #31117, #13947, #135328, #134329, #182818, #76611, #44300, #165658, #184792, #180841, #106945, #197001, #168618, #151484, #27156, #58467, #181825, #43304, #30118, #104972, #169620, #91759, #29140, #10981 ),
 .UNSPECIFIED., .F., .F.,
 ( 4, 2, 2, 2, 2, 2, 2, 2, 2, 2, 2, 4 ),
 ( 1.968491853871462031E-07, 0.0003260565056758917544, 0.0006519161621663963025, 0.0009777758186569011217, 0.001303635475147405616, 0.001955354788128404846, 0.002607074101109404726, 0.003258793414090403739, 0.003910512727071403620, 0.004562232040052403501, 0.004888091696542901272, 0.005213951353033399044 ),
 .UNSPECIFIED. ) ;
#24509=DIRECTION ( 'NONE',  ( -1.000000000000000000, 0.000000000000000000, 0.000000000000000000 ) ) ;
#24537=EDGE_CURVE ( 'NONE', #74939, #108968, #153182, .T. ) ;
#24553=AXIS2_PLACEMENT_3D ( 'NONE', #178300, #5422, #4421 ) ;
#24596=CYLINDRICAL_SURFACE ( 'NONE', #111451, 1.500000000000001332 ) ;
#24631=DIRECTION ( 'NONE',  ( -0.000000000000000000, -0.000000000000000000, 1.000000000000000000 ) ) ;
#24633=CARTESIAN_POINT ( 'NONE',  ( 16.37811251030165849, -0.9487569900773658027, -59.27680374464309665 ) ) ;
#24637=VERTEX_POINT ( 'NONE', #120857 ) ;
#24639=EDGE_CURVE ( 'NONE', #179364, #113699, #76347, .T. ) ;
#24652=CARTESIAN_POINT ( 'NONE',  ( -11.74264578624799782, -36.14014761921581709, -1.599999999999999867 ) ) ;
#24661=CARTESIAN_POINT ( 'NONE',  ( 31.47347929072392247, -24.22385046035867262, -19.66336643903433767 ) ) ;
#24662=CARTESIAN_POINT ( 'NONE',  ( -26.46959431505283789, -27.26463967846487435, -25.00000000000000000 ) ) ;
#24668=EDGE_CURVE ( 'NONE', #19818, #122419, #104712, .T. ) ;
#24677=ORIENTED_EDGE ( 'NONE', *, *, #121976, .T. ) ;
#24689=CARTESIAN_POINT ( 'NONE',  ( -29.64655366937558867, -26.74020568361526529, -17.07338589137929574 ) ) ;
#24713=CARTESIAN_POINT ( 'NONE',  ( -22.81625015709510507, 31.40387420917330275, -4.924999997268813878 ) ) ;
#24748=CYLINDRICAL_SURFACE ( 'NONE', #43981, 1.499999999999994449 ) ;
#24783=EDGE_LOOP ( 'NONE', ( #9417, #54938, #40276, #29561 ) ) ;
#24839=VECTOR ( 'NONE', #7343, 1000.000000000000000 ) ;
#24848=EDGE_LOOP ( 'NONE', ( #145730, #192513, #149528, #70905, #9465 ) ) ;
#24861=CARTESIAN_POINT ( 'NONE',  ( 0.000000000000000000, 0.000000000000000000, -65.00100000000003320 ) ) ;
#24887=DIRECTION ( 'NONE',  ( 1.000000000000000000, 0.000000000000000000, 0.000000000000000000 ) ) ;
#24897=CARTESIAN_POINT ( 'NONE',  ( 0.000000000000000000, -105.0000000000000000, 12.00000000000000355 ) ) ;
#24960=CARTESIAN_POINT ( 'NONE',  ( -9.327895405754907554E-15, -64.84118668444966715, -25.00000000000000000 ) ) ;
#24989=ADVANCED_FACE ( 'NONE', ( #111653 ), #79454, .F. ) ;
#25077=CARTESIAN_POINT ( 'NONE',  ( -17.60909914540868115, 15.84704938773722560, -54.71262039249372577 ) ) ;
#25096=CARTESIAN_POINT ( 'NONE',  ( -16.29108346408469288, -34.51247628902108033, -22.00899094814154822 ) ) ;
#25100=CARTESIAN_POINT ( 'NONE',  ( 10.19682395672834119, -9.344414726942043004, -62.53306532695916786 ) ) ;
#25136=CARTESIAN_POINT ( 'NONE',  ( 26.05560406886092295, -30.01072603040624998, -20.45417971608936725 ) ) ;
#25140=CARTESIAN_POINT ( 'NONE',  ( -6.020228577223754586E-15, 39.95556452105416412, -4.249999994537627224 ) ) ;
#25158=AXIS2_PLACEMENT_3D ( 'NONE', #53461, #38301, #99955 ) ;
#25192=CARTESIAN_POINT ( 'NONE',  ( -29.86685920354755552, 21.69954338932564397, -5.324999997268814234 ) ) ;
#25210=ORIENTED_EDGE ( 'NONE', *, *, #10139, .F. ) ;
#25216=CARTESIAN_POINT ( 'NONE',  ( -27.99776551637687305, -28.30561827218003046, -16.93438536460645949 ) ) ;
#25217=VERTEX_POINT ( 'NONE', #143785 ) ;
#25243=CYLINDRICAL_SURFACE ( 'NONE', #166356, 24.30000000000003268 ) ;
#25268=CIRCLE ( 'NONE', #147520, 31.90000000000003411 ) ;
#25293=VECTOR ( 'NONE', #35104, 1000.000000000000000 ) ;
#25368=EDGE_LOOP ( 'NONE', ( #119199, #156979, #46328, #191792, #150172, #57214 ) ) ;
#25387=VERTEX_POINT ( 'NONE', #7262 ) ;
#25396=CARTESIAN_POINT ( 'NONE',  ( 0.000000000000000000, 0.000000000000000000, -63.95112321872120731 ) ) ;
#25398=DIRECTION ( 'NONE',  ( -0.000000000000000000, -0.000000000000000000, 1.000000000000000000 ) ) ;
#25422=ORIENTED_EDGE ( 'NONE', *, *, #30838, .T. ) ;
#25423=EDGE_CURVE ( 'NONE', #71084, #197513, #67946, .T. ) ;
#25436=ORIENTED_EDGE ( 'NONE', *, *, #98879, .T. ) ;
#25455=ORIENTED_EDGE ( 'NONE', *, *, #183353, .T. ) ;
#25478=EDGE_LOOP ( 'NONE', ( #158929, #120044, #87890, #82703 ) ) ;
#25545=CYLINDRICAL_SURFACE ( 'NONE', #57024, 6.100000000000006750 ) ;
#25552=CARTESIAN_POINT ( 'NONE',  ( -38.00000000000000711, 2.428612866367529932E-14, -2.000000000000000000 ) ) ;
#25603=ORIENTED_EDGE ( 'NONE', *, *, #41891, .F. ) ;
#25627=VERTEX_POINT ( 'NONE', #112457 ) ;
#25631=CARTESIAN_POINT ( 'NONE',  ( 0.7573736981518488509, 8.898500934826572006, -61.93579448831083312 ) ) ;
#25635=CYLINDRICAL_SURFACE ( 'NONE', #199637, 1.500000000000001332 ) ;
#25638=LINE ( 'NONE', #119626, #182422 ) ;
#25653=ADVANCED_FACE ( 'NONE', ( #65950 ), #101270, .T. ) ;
#25660=CARTESIAN_POINT ( 'NONE',  ( -22.81625015709510507, 31.40387420917330275, -8.924999997268814766 ) ) ;
#25669=CARTESIAN_POINT ( 'NONE',  ( 37.24154831888315442, -19.83237144080993275, -19.76300508100036524 ) ) ;
#25685=CARTESIAN_POINT ( 'NONE',  ( 4.595912276381225681, -38.76652190273247811, -23.69787631203871214 ) ) ;
#25695=CARTESIAN_POINT ( 'NONE',  ( -27.44803035730395635, -28.83687526680896340, -16.92468093647912752 ) ) ;
#25713=ORIENTED_EDGE ( 'NONE', *, *, #162842, .T. ) ;
#25715=CARTESIAN_POINT ( 'NONE',  ( -17.18269478283316332, 17.18269478283309226, -65.00100000000003320 ) ) ;
#25718=CARTESIAN_POINT ( 'NONE',  ( 11.40812507854754365, 35.11059874428196537, -5.224999997268813701 ) ) ;
#25752=DIRECTION ( 'NONE',  ( -1.000000000000000000, 0.000000000000000000, 0.000000000000000000 ) ) ;
#25777=CARTESIAN_POINT ( 'NONE',  ( 0.000000000000000000, 0.000000000000000000, -18.00000000000000000 ) ) ;
#25787=ORIENTED_EDGE ( 'NONE', *, *, #128552, .F. ) ;
#25829=ADVANCED_FACE ( 'NONE', ( #55782 ), #134639, .F. ) ;
#25846=VECTOR ( 'NONE', #45626, 1000.000000000000000 ) ;
#25876=CARTESIAN_POINT ( 'NONE',  ( -14.62203461105304036, -16.12203461105356794, -56.14925526931841659 ) ) ;
#25881=CARTESIAN_POINT ( 'NONE',  ( -28.92784451463922579, -27.23096741515445629, -20.32502560054414076 ) ) ;
#25891=CARTESIAN_POINT ( 'NONE',  ( 29.86685920354754842, -21.69954338932559068, -5.824999997268813345 ) ) ;
#25944=CARTESIAN_POINT ( 'NONE',  ( -6.100000000000006750, 6.426762577456935076E-14, -64.92279855667830191 ) ) ;
#25960=CARTESIAN_POINT ( 'NONE',  ( 1.508955259217861487E-14, -71.74905152827281540, -24.99410988490251029 ) ) ;
#25966=ORIENTED_EDGE ( 'NONE', *, *, #191573, .F. ) ;
#25973=EDGE_LOOP ( 'NONE', ( #153117, #171378, #73335, #185218, #84762 ) ) ;
#25997=B_SPLINE_CURVE_WITH_KNOTS ( 'NONE', 3,
 ( #131347, #147533, #102018, #86845 ),
 .UNSPECIFIED., .F., .F.,
 ( 4, 4 ),
 ( 0.000000000000000000, 0.003358941478145230711 ),
 .UNSPECIFIED. ) ;
#26094=CARTESIAN_POINT ( 'NONE',  ( 12.24802307403557933, -10.74802307403627921, -61.53034260416801260 ) ) ;
#26112=DIRECTION ( 'NONE',  ( 1.000000000000000000, 8.881784197001252323E-16, 0.000000000000000000 ) ) ;
#26122=EDGE_CURVE ( 'NONE', #25627, #5010, #132627, .T. ) ;
#26129=CARTESIAN_POINT ( 'NONE',  ( 24.54195369798078374, -31.38977029645258909, -21.36864394644164733 ) ) ;
#26133=CARTESIAN_POINT ( 'NONE',  ( -38.00000000000001421, 12.34694845685046438, -9.849999994537625980 ) ) ;
#26184=CARTESIAN_POINT ( 'NONE',  ( -5.950531402560715689E-15, 38.81732327939063509, -5.624999997268813168 ) ) ;
#26185=FACE_OUTER_BOUND ( 'NONE', #151731, .T. ) ;
#26200=CARTESIAN_POINT ( 'NONE',  ( -4.647474457565486646E-15, 28.90000000000004476, -52.65483682830183199 ) ) ;
#26207=CARTESIAN_POINT ( 'NONE',  ( -25.49187754477127399, -30.53313611124044158, -20.74730905735241393 ) ) ;
#26221=CARTESIAN_POINT ( 'NONE',  ( 22.45286902209802804, -1.470710558936461521, -55.62279185774873014 ) ) ;
#26234=CARTESIAN_POINT ( 'NONE',  ( 3.503282210674389052, -48.86437366581480291, -35.00000000000000000 ) ) ;
#26286=EDGE_CURVE ( 'NONE', #41521, #11425, #45774, .T. ) ;
#26339=CARTESIAN_POINT ( 'NONE',  ( -5.284191517680379313, 3.873512393789712238, -62.43104308550747561 ) ) ;
#26342=CARTESIAN_POINT ( 'NONE',  ( 0.9209418409973284536, 31.60467972784392643, -46.08008370242323792 ) ) ;
#26363=FACE_OUTER_BOUND ( 'NONE', #86357, .T. ) ;
#26381=CARTESIAN_POINT ( 'NONE',  ( 37.66961640367472341, -4.999999999999976019, -25.00000000000000000 ) ) ;
#26388=CARTESIAN_POINT ( 'NONE',  ( -28.90000000000004476, 2.980639576201346218E-13, -49.67367017693150189 ) ) ;
#26393=CARTESIAN_POINT ( 'NONE',  ( 23.48529157249599564, 32.32473071737754111, -4.699999999999999289 ) ) ;
#26463=DIRECTION ( 'NONE',  ( 1.000000000000000000, 0.000000000000000000, 3.469446951953612217E-15 ) ) ;
#26466=AXIS2_PLACEMENT_3D ( 'NONE', #82874, #100043, #34401 ) ;
#26532=DIRECTION ( 'NONE',  ( -0.000000000000000000, -0.000000000000000000, 1.000000000000000000 ) ) ;
#26602=CARTESIAN_POINT ( 'NONE',  ( 1.105192082801339515, 29.38149524799785084, -52.12050502002018959 ) ) ;
#26634=LINE ( 'NONE', #198454, #82046 ) ;
#26649=CARTESIAN_POINT ( 'NONE',  ( 3.766062262543149401E-15, -39.95556452105413570, -5.500000000000000000 ) ) ;
#26654=EDGE_CURVE ( 'NONE', #89236, #140310, #145923, .T. ) ;
#26655=CARTESIAN_POINT ( 'NONE',  ( 0.2056090276421982943, 16.68933881255749085, -59.13845611041300288 ) ) ;
#26678=CARTESIAN_POINT ( 'NONE',  ( 8.377002814025898303, -36.45346134345118827, -31.71922177526206710 ) ) ;
#26682=ORIENTED_EDGE ( 'NONE', *, *, #129852, .F. ) ;
#26705=EDGE_CURVE ( 'NONE', #105638, #107603, #61915, .T. ) ;
#26706=ORIENTED_EDGE ( 'NONE', *, *, #63306, .F. ) ;
#26708=DIRECTION ( 'NONE',  ( 0.9974398506828147104, -0.07151044867601312471, 6.797078445321206297E-16 ) ) ;
#26711=CARTESIAN_POINT ( 'NONE',  ( 36.91746824999999177, 2.880721459617395097E-14, -5.624999997268813168 ) ) ;
#26715=CARTESIAN_POINT ( 'NONE',  ( 6.767090645865133425, -4.798697441033914934, -64.13056706087778025 ) ) ;
#26769=PLANE ( 'NONE',  #119641 ) ;
#26788=FACE_OUTER_BOUND ( 'NONE', #168802, .T. ) ;
#26840=EDGE_CURVE ( 'NONE', #191474, #188707, #78894, .T. ) ;
#26862=DIRECTION ( 'NONE',  ( -0.000000000000000000, -0.000000000000000000, 1.000000000000000000 ) ) ;
#26887=CARTESIAN_POINT ( 'NONE',  ( -31.05874284564964682, -25.21260394624121304, -18.17714894250296709 ) ) ;
#26944=VECTOR ( 'NONE', #55819, 1000.000000000000000 ) ;
#26945=EDGE_LOOP ( 'NONE', ( #611, #153759, #65082, #146158 ) ) ;
#26959=CARTESIAN_POINT ( 'NONE',  ( -1.371772415827590191E-14, -64.85621347262016911, -24.99999966871768819 ) ) ;
#27004=VECTOR ( 'NONE', #88775, 1000.000000000000000 ) ;
#27040=CARTESIAN_POINT ( 'NONE',  ( 11.30153831258469843, -180.0000000000000000, -23.00000000000000000 ) ) ;
#27126=ORIENTED_EDGE ( 'NONE', *, *, #107016, .F. ) ;
#27132=CARTESIAN_POINT ( 'NONE',  ( 37.99999999999999289, 2.893978650043524126E-14, -4.749999994537627224 ) ) ;
#27138=DIRECTION ( 'NONE',  ( 1.000000000000000000, -3.552713678800500929E-15, 0.000000000000000000 ) ) ;
#27156=CARTESIAN_POINT ( 'NONE',  ( -22.44763431097441142, 1.469699867062036480, -58.07555020237587939 ) ) ;
#27162=CYLINDRICAL_SURFACE ( 'NONE', #127105, 1.500000000000001332 ) ;
#27169=CARTESIAN_POINT ( 'NONE',  ( 19.97888994334919843, -34.65319547504301312, 0.000000000000000000 ) ) ;
#27182=CARTESIAN_POINT ( 'NONE',  ( 36.91746824999999177, 2.880721459617395097E-14, -2.124999997268813168 ) ) ;
#27204=CARTESIAN_POINT ( 'NONE',  ( -30.11221142034060350, -26.30828378221708519, -17.15571736053662377 ) ) ;
#27218=CARTESIAN_POINT ( 'NONE',  ( 22.10945809693574304, -1.344113590474677267, -55.87741762761908859 ) ) ;
#27225=CARTESIAN_POINT ( 'NONE',  ( 10.59477242850415024, -90.60836494048558620, -25.00000000000000000 ) ) ;
#27253=EDGE_LOOP ( 'NONE', ( #10796, #34522, #184016, #2962, #187341 ) ) ;
#27274=LINE ( 'NONE', #197115, #168112 ) ;
#27336=CARTESIAN_POINT ( 'NONE',  ( 30.74264578624799782, 22.33583958711400541, -6.800000000000000711 ) ) ;
#27340=CARTESIAN_POINT ( 'NONE',  ( -20.53360937444638168, -31.96911244174559386, -23.96531494639239313 ) ) ;
#27373=CIRCLE ( 'NONE', #46676, 16.70000000000002061 ) ;
#27386=CARTESIAN_POINT ( 'NONE',  ( 0.000000000000000000, -165.0000000000000000, 12.00000000000000355 ) ) ;
#27401=CARTESIAN_POINT ( 'NONE',  ( 0.000000000000000000, 0.000000000000000000, -62.58071313852362039 ) ) ;
#27431=DIRECTION ( 'NONE',  ( 1.000000000000000000, 0.000000000000000000, 0.000000000000000000 ) ) ;
#27614=ADVANCED_FACE ( 'NONE', ( #7028 ), #58763, .T. ) ;
#27627=DIRECTION ( 'NONE',  ( 1.000000000000000000, 0.000000000000000000, 0.000000000000000000 ) ) ;
#27638=CARTESIAN_POINT ( 'NONE',  ( -0.1121107154831215841, -24.30000000000003624, -54.21489346206830362 ) ) ;
#27640=DIRECTION ( 'NONE',  ( -0.000000000000000000, -0.000000000000000000, 1.000000000000000000 ) ) ;
#27657=CARTESIAN_POINT ( 'NONE',  ( 30.74264578624799782, 22.33583958711400541, -8.800000000000000711 ) ) ;
#27686=ORIENTED_EDGE ( 'NONE', *, *, #95255, .F. ) ;
#27708=VERTEX_POINT ( 'NONE', #37380 ) ;
#27712=CARTESIAN_POINT ( 'NONE',  ( -36.91746825000001309, -11.99521256947794789, -10.52499999726881441 ) ) ;
#27850=VERTEX_POINT ( 'NONE', #66720 ) ;
#27853=ADVANCED_FACE ( 'NONE', ( #142563, #160727 ), #22219, .T. ) ;
#27870=CARTESIAN_POINT ( 'NONE',  ( -14.62203461105279700, -15.93801742227414486, -58.64843802457497901 ) ) ;
#27888=CARTESIAN_POINT ( 'NONE',  ( -32.05804330925093382, -23.92378017333652451, -20.06701077757416840 ) ) ;
#27906=CARTESIAN_POINT ( 'NONE',  ( 2.802625768539491968, -39.09149893265183806, -33.00000000000000000 ) ) ;
#27924=VERTEX_POINT ( 'NONE', #157747 ) ;
#27937=CIRCLE ( 'NONE', #150601, 13.70000000000001528 ) ;
#27944=ADVANCED_FACE ( 'NONE', ( #23224 ), #84867, .T. ) ;
#27949=CARTESIAN_POINT ( 'NONE',  ( -11.30153831258470731, -180.0000000000000000, -25.00000000000000000 ) ) ;
#27962=CARTESIAN_POINT ( 'NONE',  ( 17.18269478283314911, 17.18269478283310647, -56.77278709839600879 ) ) ;
#27984=B_SPLINE_CURVE_WITH_KNOTS ( 'NONE', 3,
 ( #148521, #146497, #176868, #55502, #194038, #22171, #10011, #195029, #83821, #7988, #116175, #145501, #6982, #131338, #54503, #179875, #68662, #181852, #197028, #109714, #88830, #196041, #141045, #150523 ),
 .UNSPECIFIED., .F., .F.,
 ( 4, 2, 2, 2, 2, 2, 2, 2, 2, 2, 2, 4 ),
 ( 1.968491853561852430E-07, 0.0003260565056758578189, 0.0006519161621663594397, 0.0009777758186568610062, 0.001303635475147362681, 0.001955354788128363646, 0.002607074101109364394, 0.003258793414090365576, 0.003910512727071366323, 0.004562232040052367071, 0.004888091696542867445, 0.005213951353033367819 ),
 .UNSPECIFIED. ) ;
#28022=ORIENTED_EDGE ( 'NONE', *, *, #98879, .F. ) ;
#28026=( LENGTH_UNIT ( ) NAMED_UNIT ( * ) SI_UNIT ( .MILLI., .METRE. ) );
#28034=VECTOR ( 'NONE', #197159, 1000.000000000000000 ) ;
#28066=EDGE_CURVE ( 'NONE', #48561, #28823, #172825, .T. ) ;
#28068=ORIENTED_EDGE ( 'NONE', *, *, #134694, .F. ) ;
#28080=CARTESIAN_POINT ( 'NONE',  ( -17.60430054815012113, 16.43460366218429414, -54.39459263522237364 ) ) ;
#28113=DIRECTION ( 'NONE',  ( -1.000000000000000000, 0.000000000000000000, -4.336808689942016750E-16 ) ) ;
#28130=EDGE_LOOP ( 'NONE', ( #185336, #131114, #86532, #183362 ) ) ;
#28136=CARTESIAN_POINT ( 'NONE',  ( 29.86685920354754842, -21.69954338932559068, -2.324999997268813345 ) ) ;
#28169=CIRCLE ( 'NONE', #166867, 61.99999999999998579 ) ;
#28203=ORIENTED_EDGE ( 'NONE', *, *, #79617, .T. ) ;
#28209=CARTESIAN_POINT ( 'NONE',  ( -27.67003201002285806, -28.46598819372283984, -20.09023003179696332 ) ) ;
#28211=VERTEX_POINT ( 'NONE', #132395 ) ;
#28225=CARTESIAN_POINT ( 'NONE',  ( 24.30000000000003624, -0.1121107154831149089, -54.21489346206828230 ) ) ;
#28245=DIRECTION ( 'NONE',  ( 1.000000000000000000, 0.000000000000000000, 3.469446951953612217E-15 ) ) ;
#28312=AXIS2_PLACEMENT_3D ( 'NONE', #41777, #70107, #193458 ) ;
#28341=CARTESIAN_POINT ( 'NONE',  ( -22.96834507599308139, 21.15706064682967380, -46.65423976109394744 ) ) ;
#28345=CYLINDRICAL_SURFACE ( 'NONE', #138251, 16.70000000000002061 ) ;
#28378=CARTESIAN_POINT ( 'NONE',  ( -8.788389965099090873, 0.9205664139721330130, -61.95844424577442311 ) ) ;
#28400=DIRECTION ( 'NONE',  ( -0.000000000000000000, -0.000000000000000000, 1.000000000000000000 ) ) ;
#28405=CARTESIAN_POINT ( 'NONE',  ( -3.874011537017815421, -5.374011537017721274, -64.44758591613756948 ) ) ;
#28409=EDGE_CURVE ( 'NONE', #196359, #111207, #196092, .T. ) ;
#28430=CARTESIAN_POINT ( 'NONE',  ( -6.873473828371201577, 5.267258167721591278, -64.05152134952703591 ) ) ;
#28465=EDGE_LOOP ( 'NONE', ( #148974, #121662, #36817, #23839 ) ) ;
#28532=CARTESIAN_POINT ( 'NONE',  ( -7.503727747132419523, 1.500047742438238352, -64.26135111332263250 ) ) ;
#28572=ADVANCED_FACE ( 'NONE', ( #133387 ), #25243, .F. ) ;
#28585=ORIENTED_EDGE ( 'NONE', *, *, #96802, .T. ) ;
#28614=DIRECTION ( 'NONE',  ( -1.000000000000000000, 0.000000000000000000, 0.000000000000000000 ) ) ;
#28621=CARTESIAN_POINT ( 'NONE',  ( 15.06137443927351249, -15.06137443927345210, -58.85720012050613548 ) ) ;
#28624=CARTESIAN_POINT ( 'NONE',  ( -3.921794856358155723, -4.985877495913942248, -64.49392664332130209 ) ) ;
#28639=EDGE_CURVE ( 'NONE', #138825, #39558, #39383, .T. ) ;
#28643=CARTESIAN_POINT ( 'NONE',  ( -11.74264578624800670, 36.14014761921585972, -6.400000000000000355 ) ) ;
#28673=VERTEX_POINT ( 'NONE', #165734 ) ;
#28700=CARTESIAN_POINT ( 'NONE',  ( 0.7811817504636909826, 13.90344567069866599, -62.49835084440437072 ) ) ;
#28742=EDGE_CURVE ( 'NONE', #178146, #15137, #54903, .T. ) ;
#28758=CARTESIAN_POINT ( 'NONE',  ( 1.473582404419343517, 30.72737312094908901, -50.56799658405696363 ) ) ;
#28784=DIRECTION ( 'NONE',  ( 1.000000000000000000, 0.000000000000000000, 0.000000000000000000 ) ) ;
#28820=ORIENTED_EDGE ( 'NONE', *, *, #170016, .T. ) ;
#28823=VERTEX_POINT ( 'NONE', #187617 ) ;
#28831=EDGE_CURVE ( 'NONE', #193677, #173655, #150189, .T. ) ;
#28833=CARTESIAN_POINT ( 'NONE',  ( -23.76806875053281942, -29.07479876791513362, -18.77372378131338948 ) ) ;
#28838=ORIENTED_EDGE ( 'NONE', *, *, #121940, .F. ) ;
#28850=CARTESIAN_POINT ( 'NONE',  ( -3.503282210674349528, -48.86437366581481001, -23.00000000000000000 ) ) ;
#28872=CARTESIAN_POINT ( 'NONE',  ( 36.91746824999999177, 11.99521256947799230, -7.524999997268813523 ) ) ;
#28880=ORIENTED_EDGE ( 'NONE', *, *, #99957, .F. ) ;
#28891=CARTESIAN_POINT ( 'NONE',  ( 3.503282210674364627, -48.86437366581479580, -25.00000000000000000 ) ) ;
#28909=ORIENTED_EDGE ( 'NONE', *, *, #116672, .F. ) ;
#28973=CARTESIAN_POINT ( 'NONE',  ( 21.30000000000002913, -7.567280135845077329E-14, -64.92279855667830191 ) ) ;
#28986=AXIS2_PLACEMENT_3D ( 'NONE', #113724, #84387, #86401 ) ;
#29006=VERTEX_POINT ( 'NONE', #79415 ) ;
#29018=CIRCLE ( 'NONE', #100123, 61.99999999999998579 ) ;
#29077=LINE ( 'NONE', #152399, #192837 ) ;
#29093=CARTESIAN_POINT ( 'NONE',  ( -1.220661533321835801, -14.30620887846973055, -60.18359034246772410 ) ) ;
#29107=ORIENTED_EDGE ( 'NONE', *, *, #68319, .T. ) ;
#29115=CARTESIAN_POINT ( 'NONE',  ( 36.91746824999999177, 2.880721459617395097E-14, -6.124999997268813168 ) ) ;
#29140=CARTESIAN_POINT ( 'NONE',  ( -21.30000000000002913, 0.1105695005020707194, -58.85720012050614258 ) ) ;
#29165=EDGE_CURVE ( 'NONE', #49313, #196867, #156659, .T. ) ;
#29167=CARTESIAN_POINT ( 'NONE',  ( 36.91746824999999177, 2.880721459617395097E-14, -10.12499999726881583 ) ) ;
#29189=CARTESIAN_POINT ( 'NONE',  ( -35.06017246933182463, -19.40171014085577283, -22.29041292151830334 ) ) ;
#29190=ORIENTED_EDGE ( 'NONE', *, *, #125853, .F. ) ;
#29237=ORIENTED_EDGE ( 'NONE', *, *, #129082, .F. ) ;
#29313=CARTESIAN_POINT ( 'NONE',  ( -4.384162112346980500, 4.242540618128916918, -62.50719930893271226 ) ) ;
#29317=CARTESIAN_POINT ( 'NONE',  ( -21.88112277201193123, 20.03432139805442702, -48.74685162679677575 ) ) ;
#29320=DIRECTION ( 'NONE',  ( 1.000000000000000000, 0.000000000000000000, 0.000000000000000000 ) ) ;
#29329=EDGE_CURVE ( 'NONE', #183247, #158096, #119715, .T. ) ;
#29365=CARTESIAN_POINT ( 'NONE',  ( -38.00000000000000711, 2.893978650043524126E-14, -25.00000000000000000 ) ) ;
#29383=CARTESIAN_POINT ( 'NONE',  ( 9.100000000000001421, 0.000000000000000000, -63.95112321872120731 ) ) ;
#29388=ORIENTED_EDGE ( 'NONE', *, *, #195257, .F. ) ;
#29408=CARTESIAN_POINT ( 'NONE',  ( -6.719938155502488186, 4.704672000039124669, -64.14994679864909699 ) ) ;
#29440=DIRECTION ( 'NONE',  ( 1.000000000000000000, 6.391086490440868450E-16, 0.000000000000000000 ) ) ;
#29470=CARTESIAN_POINT ( 'NONE',  ( 22.99604614807110181, -21.49604614807104142, -49.67998909148434450 ) ) ;
#29475=CARTESIAN_POINT ( 'NONE',  ( 2.577820198429831642E-15, 9.100000000000001421, -61.89430850415821794 ) ) ;
#29502=CARTESIAN_POINT ( 'NONE',  ( 10.74802307403555623, 10.74802307403551360, -64.92279855667830191 ) ) ;
#29508=CARTESIAN_POINT ( 'NONE',  ( -6.139823915386823927, 0.3964520562364309830, -64.52448473163053677 ) ) ;
#29523=B_SPLINE_CURVE_WITH_KNOTS ( 'NONE', 3,
 ( #194076, #28225, #39371, #11044, #10047, #181887, #103045, #177903, #57550, #102046, #193063, #119219, #26221, #27218, #164727, #8026, #162715, #180904, #117211, #131375, #54539, #166721 ),
 .UNSPECIFIED., .F., .F.,
 ( 4, 2, 2, 2, 2, 2, 2, 2, 2, 2, 4 ),
 ( 1.967889507820273575E-07, 0.0003311341139580519974, 0.0006620714389653219612, 0.0009930087639725918708, 0.001323946088979861780, 0.002647695389008961585, 0.003309570039023516149, 0.003971444689038069846, 0.004633319339052623977, 0.004964256664059899307, 0.005295193989067173770 ),
 .UNSPECIFIED. ) ;
#29561=ORIENTED_EDGE ( 'NONE', *, *, #22985, .T. ) ;
#29563=ORIENTED_EDGE ( 'NONE', *, *, #80974, .T. ) ;
#29572=CARTESIAN_POINT ( 'NONE',  ( 16.68945015508927554, -0.2045547421925976994, -61.35148950497489295 ) ) ;
#29587=CARTESIAN_POINT ( 'NONE',  ( -24.30000000000003268, 2.668083032619853614E-13, -54.21489346206828230 ) ) ;
#29594=CARTESIAN_POINT ( 'NONE',  ( 10.65638358537376362, -44.90791467878717924, -23.56120423312990297 ) ) ;
#29598=CARTESIAN_POINT ( 'NONE',  ( -1.500606516337470886, -22.62812085840269560, -55.49205433527804132 ) ) ;
#29612=VERTEX_POINT ( 'NONE', #187355 ) ;
#29615=CARTESIAN_POINT ( 'NONE',  ( 37.99999999999999289, 2.893978650043524126E-14, -3.000000000000000000 ) ) ;
#29620=CARTESIAN_POINT ( 'NONE',  ( 0.000000000000000000, 0.000000000000000000, -64.92279855667830191 ) ) ;
#29639=EDGE_LOOP ( 'NONE', ( #1419, #158329 ) ) ;
#29641=CARTESIAN_POINT ( 'NONE',  ( 18.67464278970748381, -33.09908666442214553, -25.63618526508991380 ) ) ;
#29749=CARTESIAN_POINT ( 'NONE',  ( 11.30153831258470731, -188.0000000000000000, -25.00000000000000000 ) ) ;
#29757=CARTESIAN_POINT ( 'NONE',  ( -22.41419083229811804, -22.69922180740366358, -49.13275782002544645 ) ) ;
#29807=CARTESIAN_POINT ( 'NONE',  ( -12.38288446667173837, -41.98357824128019899, -20.85955585120584033 ) ) ;
#29830=CARTESIAN_POINT ( 'NONE',  ( 1.500000000004064082, 7.599999999999568878, -62.20201607440122871 ) ) ;
#29833=CARTESIAN_POINT ( 'NONE',  ( 1.500000000000005329, 15.20000000000001883, -61.96904110198155280 ) ) ;
#29838=CARTESIAN_POINT ( 'NONE',  ( 26.46959431505287341, -27.26463967846483527, -11.00411086000093519 ) ) ;
#29848=CARTESIAN_POINT ( 'NONE',  ( -11.40812507854755609, 35.11059874428196537, -9.024999997268814411 ) ) ;
#29858=CARTESIAN_POINT ( 'NONE',  ( 5.374011537017778117, -5.374011537017756801, -64.92279855667830191 ) ) ;
#29944=CARTESIAN_POINT ( 'NONE',  ( 1.022580077288041090E-15, 16.70000000000002061, -61.34707691135562868 ) ) ;
#29952=CARTESIAN_POINT ( 'NONE',  ( 11.80868324581537543, 11.80868324581533990, -64.92279855667830191 ) ) ;
#30056=VECTOR ( 'NONE', #139006, 1000.000000000000000 ) ;
#30057=CARTESIAN_POINT ( 'NONE',  ( 0.2076433133274071252, 13.70000000000001528, -60.44446360152740993 ) ) ;
#30070=CARTESIAN_POINT ( 'NONE',  ( 17.57923699280061314, -16.49001817116781865, -54.37788754106805555 ) ) ;
#30073=CARTESIAN_POINT ( 'NONE',  ( -0.7820921006973207135, -16.49581645235993221, -59.22453004090982631 ) ) ;
#30079=CARTESIAN_POINT ( 'NONE',  ( -20.37894794865908921, -22.50499723050164746, -47.85318311809130165 ) ) ;
#30096=CARTESIAN_POINT ( 'NONE',  ( 29.86685920354754842, -21.69954338932559068, -4.324999997268814234 ) ) ;
#30108=CARTESIAN_POINT ( 'NONE',  ( 5.169469635059304125, 6.863180944108024484, -62.01598399707661002 ) ) ;
#30118=CARTESIAN_POINT ( 'NONE',  ( -21.52594032250404865, 0.8193109935769098406, -58.70475745007092883 ) ) ;
#30142=CARTESIAN_POINT ( 'NONE',  ( 22.81625015709510151, -31.40387420917324590, -10.42499999726881299 ) ) ;
#30145=CARTESIAN_POINT ( 'NONE',  ( 1.046079508147533810, 23.87944126242780740, -57.07319907805452175 ) ) ;
#30171=ADVANCED_FACE ( 'NONE', ( #143796 ), #78149, .F. ) ;
#30180=CARTESIAN_POINT ( 'NONE',  ( 26.46959431505287341, -27.26463967846483527, -11.00411086000093519 ) ) ;
#30215=ORIENTED_EDGE ( 'NONE', *, *, #187746, .F. ) ;
#30224=VECTOR ( 'NONE', #12332, 1000.000000000000000 ) ;
#30292=CARTESIAN_POINT ( 'NONE',  ( -32.09281931051391012, -20.34824190692417289, -24.99999999999999289 ) ) ;
#30294=AXIS2_PLACEMENT_3D ( 'NONE', #32584, #2232, #63914 ) ;
#30333=CARTESIAN_POINT ( 'NONE',  ( -7.503800738396974701, 1.500046863536517172, -62.22166870076607381 ) ) ;
#30345=CARTESIAN_POINT ( 'NONE',  ( 0.000000000000000000, 0.000000000000000000, -56.46919128290398504 ) ) ;
#30357=CARTESIAN_POINT ( 'NONE',  ( 5.000000000000000000, 0.000000000000000000, -18.00000000000000000 ) ) ;
#30391=CARTESIAN_POINT ( 'NONE',  ( -10.06251177737617120, -45.32665049860681705, -23.77652626631511978 ) ) ;
#30423=ORIENTED_EDGE ( 'NONE', *, *, #138817, .F. ) ;
#30452=CARTESIAN_POINT ( 'NONE',  ( 22.55670631985092456, -22.55670631985084995, -49.13275782002545355 ) ) ;
#30466=CARTESIAN_POINT ( 'NONE',  ( 0.000000000000000000, 0.000000000000000000, -35.00000000000000000 ) ) ;
#30490=CARTESIAN_POINT ( 'NONE',  ( -6.100000000000009415, 0.2000799437545254522, -64.53213882399991519 ) ) ;
#30540=ORIENTED_EDGE ( 'NONE', *, *, #100204, .T. ) ;
#30575=CARTESIAN_POINT ( 'NONE',  ( 0.000000000000000000, 0.000000000000000000, -64.92279855667830191 ) ) ;
#30585=CARTESIAN_POINT ( 'NONE',  ( -0.5392447798056579922, -21.39623730026199411, -56.39940532337661949 ) ) ;
#30590=CARTESIAN_POINT ( 'NONE',  ( 11.30153831258470731, -190.0000000000000000, -25.00000000000000000 ) ) ;
#30602=EDGE_LOOP ( 'NONE', ( #35051, #142222, #192547, #91547 ) ) ;
#30605=CARTESIAN_POINT ( 'NONE',  ( 30.74264578624799782, 22.33583958711400541, -6.800000000000000711 ) ) ;
#30631=CARTESIAN_POINT ( 'NONE',  ( 10.75775780537444959, -37.01749054246350568, -23.73535027651007567 ) ) ;
#30659=VERTEX_POINT ( 'NONE', #182137 ) ;
#30677=VECTOR ( 'NONE', #79195, 1000.000000000000000 ) ;
#30682=EDGE_CURVE ( 'NONE', #164148, #135024, #143637, .T. ) ;
#30700=CARTESIAN_POINT ( 'NONE',  ( 193.3062444957835453, -155.7167183371837496, -25.00000000000000000 ) ) ;
#30709=CIRCLE ( 'NONE', #1684, 9.100000000000001421 ) ;
#30749=CONICAL_SURFACE ( 'NONE', #143726, 2.500000000000000000, 1.029744258676656976 ) ;
#30800=CARTESIAN_POINT ( 'NONE',  ( -12.88217944815594684, -35.43691452638693562, -29.79217952741210951 ) ) ;
#30827=DIRECTION ( 'NONE',  ( 0.000000000000000000, 0.000000000000000000, 1.000000000000000000 ) ) ;
#30838=EDGE_CURVE ( 'NONE', #177278, #34604, #192007, .T. ) ;
#30853=CARTESIAN_POINT ( 'NONE',  ( -9.100000000000001421, 9.789526074884739315E-14, -64.92279855667830191 ) ) ;
#30862=CARTESIAN_POINT ( 'NONE',  ( 3.964304649043745243, -40.57928608015685512, -25.32305239479493508 ) ) ;
#30864=CIRCLE ( 'NONE', #137370, 69.99999999999998579 ) ;
#30897=EDGE_CURVE ( 'NONE', #45388, #139989, #56501, .T. ) ;
#30915=FACE_OUTER_BOUND ( 'NONE', #76581, .T. ) ;
#30976=ORIENTED_EDGE ( 'NONE', *, *, #101847, .F. ) ;
#31071=CARTESIAN_POINT ( 'NONE',  ( -1.211883243535121890, -16.08916976210839067, -59.40465844715060229 ) ) ;
#31078=CARTESIAN_POINT ( 'NONE',  ( -20.88951479300308733, -22.87381821414430405, -47.01046684957792365 ) ) ;
#31093=CARTESIAN_POINT ( 'NONE',  ( -29.86685920354755552, 21.69954338932564397, -5.324999997268814234 ) ) ;
#31117=CARTESIAN_POINT ( 'NONE',  ( -24.30000000000003268, 2.668083032619853614E-13, -56.77278709839600879 ) ) ;
#31142=CARTESIAN_POINT ( 'NONE',  ( -29.86685920354755552, 21.69954338932564397, -9.324999997268813345 ) ) ;
#31194=B_SPLINE_CURVE_WITH_KNOTS ( 'NONE', 3,
 ( #137251, #32071, #92725, #46239, #62385, #75575, #30079, #94721, #154414, #31078, #140225, #185754, #107893, #198937, #138249, #168581, #126062, #199933, #63394, #110887 ),
 .UNSPECIFIED., .F., .F.,
 ( 4, 2, 2, 2, 2, 2, 2, 2, 2, 4 ),
 ( 0.001320702335622901420, 0.001953861884282702497, 0.002587021432942503141, 0.003220180981602304218, 0.003853340530262105296, 0.004486500078921906373, 0.005119659627581707451, 0.005752819176241508528, 0.006069398950571413404, 0.006385978724901320014 ),
 .UNSPECIFIED. ) ;
#31263=ADVANCED_FACE ( 'NONE', ( #64745 ), #186116, .F. ) ;
#31320=EDGE_CURVE ( 'NONE', #12839, #85226, #27373, .T. ) ;
#31329=CARTESIAN_POINT ( 'NONE',  ( -9.100000000000001421, 9.789526074884739315E-14, -61.89430850415821794 ) ) ;
#31363=VERTEX_POINT ( 'NONE', #189105 ) ;
#31389=CARTESIAN_POINT ( 'NONE',  ( -8.207766490800743497, -46.52841682978064597, -24.35011552987000272 ) ) ;
#31417=DIRECTION ( 'NONE',  ( -0.000000000000000000, -0.000000000000000000, 1.000000000000000000 ) ) ;
#31427=CARTESIAN_POINT ( 'NONE',  ( -15.93273212980863462, 1.322671946311657187, -61.66661032175890256 ) ) ;
#31445=CIRCLE ( 'NONE', #57309, 8.000000000000001776 ) ;
#31446=LINE ( 'NONE', #169954, #194649 ) ;
#31449=CARTESIAN_POINT ( 'NONE',  ( -12.73749492396214578, -155.7167183371837496, -25.00000000000000000 ) ) ;
#31461=DIRECTION ( 'NONE',  ( -0.000000000000000000, -0.000000000000000000, -1.000000000000000000 ) ) ;
#31489=CARTESIAN_POINT ( 'NONE',  ( -11.78083973539056473, -37.76997396076110647, -30.94638762609308458 ) ) ;
#31555=ADVANCED_FACE ( 'NONE', ( #172930 ), #2072, .F. ) ;
#31579=EDGE_CURVE ( 'NONE', #53136, #190734, #117184, .T. ) ;
#31580=CARTESIAN_POINT ( 'NONE',  ( 15.01195240492206473, -1.500078752102888879, -59.87740586969341905 ) ) ;
#31585=LINE ( 'NONE', #79065, #34035 ) ;
#31592=AXIS2_PLACEMENT_3D ( 'NONE', #83833, #192029, #161694 ) ;
#31625=CARTESIAN_POINT ( 'NONE',  ( 20.74701606029799450, -32.99105665080598015, -17.50853973932387930 ) ) ;
#31653=ORIENTED_EDGE ( 'NONE', *, *, #145117, .F. ) ;
#31655=EDGE_CURVE ( 'NONE', #127799, #156928, #80998, .T. ) ;
#31696=CARTESIAN_POINT ( 'NONE',  ( 8.788389965099115742, -0.9205664139720534100, -61.95844424577443021 ) ) ;
#31715=DIRECTION ( 'NONE',  ( -0.000000000000000000, -0.000000000000000000, 1.000000000000000000 ) ) ;
#31716=CARTESIAN_POINT ( 'NONE',  ( 1.038764921308847677, 31.48673128579449099, -49.64798258954322563 ) ) ;
#31792=CARTESIAN_POINT ( 'NONE',  ( -14.90098780495876696, -35.24605353402532160, -22.56189394118115743 ) ) ;
#31814=CARTESIAN_POINT ( 'NONE',  ( 22.99604614807110181, -21.49604614807103786, -46.28618945597792589 ) ) ;
#31817=CARTESIAN_POINT ( 'NONE',  ( 4.064918688780018385, 6.131632772416324428, -64.31816925299779086 ) ) ;
#31823=CARTESIAN_POINT ( 'NONE',  ( 21.98965532995689642, -20.07258295882801491, -51.71301205850239313 ) ) ;
#31851=CARTESIAN_POINT ( 'NONE',  ( 25.79201298823733879, -30.25621121864868357, -20.58051720723745248 ) ) ;
#31909=CARTESIAN_POINT ( 'NONE',  ( 30.74264578624799782, 22.33583958711400541, -2.799999999999999822 ) ) ;
#31934=CARTESIAN_POINT ( 'NONE',  ( -3.573655867282028392E-15, 2.428612866367529932E-14, -25.00000000000000000 ) ) ;
#31935=LINE ( 'NONE', #28973, #127387 ) ;
#32044=LINE ( 'NONE', #124028, #88561 ) ;
#32061=DIRECTION ( 'NONE',  ( 0.000000000000000000, 0.000000000000000000, 1.000000000000000000 ) ) ;
#32065=FACE_BOUND ( 'NONE', #198523, .T. ) ;
#32071=CARTESIAN_POINT ( 'NONE',  ( -19.99604614807109826, -21.65519653700129155, -48.98449577164771540 ) ) ;
#32080=ORIENTED_EDGE ( 'NONE', *, *, #150187, .T. ) ;
#32086=CARTESIAN_POINT ( 'NONE',  ( -29.86685920354755197, -21.69954338932560134, -4.924999997268813878 ) ) ;
#32133=CARTESIAN_POINT ( 'NONE',  ( -36.91746825000000598, 2.428612866367529932E-14, -11.12499999726881228 ) ) ;
#32135=CARTESIAN_POINT ( 'NONE',  ( 22.81625015709509441, 31.40387420917330275, -5.824999997268813345 ) ) ;
#32136=CARTESIAN_POINT ( 'NONE',  ( 1.500000000000323519, 7.794094698433090329, -64.20511667583481596 ) ) ;
#32137=AXIS2_PLACEMENT_3D ( 'NONE', #14292, #135670, #151821 ) ;
#32144=CARTESIAN_POINT ( 'NONE',  ( -11.67072985713514299, 9.561620553927742350, -62.04564570087489983 ) ) ;
#32159=ORIENTED_EDGE ( 'NONE', *, *, #140691, .F. ) ;
#32194=EDGE_CURVE ( 'NONE', #45716, #149545, #78987, .T. ) ;
#32289=CARTESIAN_POINT ( 'NONE',  ( -24.23981148858510792, 0.4346045811325345842, -54.26183423998841704 ) ) ;
#32336=CARTESIAN_POINT ( 'NONE',  ( 21.35939100396078771, -0.4315818942738698927, -58.81718527612542147 ) ) ;
#32357=ORIENTED_EDGE ( 'NONE', *, *, #181589, .F. ) ;
#32420=CARTESIAN_POINT ( 'NONE',  ( -0.9974278668897548217, -8.724588103088160906, -61.97156292062778249 ) ) ;
#32444=AXIS2_PLACEMENT_3D ( 'NONE', #54590, #84911, #162767 ) ;
#32449=EDGE_CURVE ( 'NONE', #158096, #89826, #62820, .T. ) ;
#32483=CARTESIAN_POINT ( 'NONE',  ( -8.945614359730852172, 0.6701480022147746629, -63.98123544873404711 ) ) ;
#32565=( BOUNDED_CURVE ( )  B_SPLINE_CURVE ( 2, ( #90162, #139631, #108308, #152825, #154816, #75000, #186171, #168978, #121491, #151845, #140636 ),
 .UNSPECIFIED., .F., .F. ) 
 B_SPLINE_CURVE_WITH_KNOTS ( ( 3, 2, 2, 2, 2, 3 ),
 ( 0.2000000000000000111, 0.2200000000000000011, 0.2400000000000000189, 0.2600000000000000644, 0.2800000000000000822, 0.3000000000000000444 ),
 .UNSPECIFIED. ) 
 CURVE ( )  GEOMETRIC_REPRESENTATION_ITEM ( )  RATIONAL_B_SPLINE_CURVE ( ( 1.000000000000000000, 0.9510565162951535312, 1.000000000000000000, 0.9510565162951535312, 1.000000000000000000, 0.9510565162951535312, 1.000000000000000000, 0.9510565162951535312, 1.000000000000000000, 0.9510565162951534202, 1.000000000000000222 ) ) 
 REPRESENTATION_ITEM ( '' )  );
#32567=DIRECTION ( 'NONE',  ( -0.000000000000000000, -0.000000000000000000, 1.000000000000000000 ) ) ;
#32571=DIRECTION ( 'NONE',  ( -0.000000000000000000, -0.000000000000000000, 1.000000000000000000 ) ) ;
#32579=FACE_BOUND ( 'NONE', #71168, .T. ) ;
#32584=CARTESIAN_POINT ( 'NONE',  ( -3.573655867282028392E-15, 2.428612866367529932E-14, -25.00000000000000000 ) ) ;
#32592=EDGE_CURVE ( 'NONE', #23346, #56239, #53157, .T. ) ;
#32618=CARTESIAN_POINT ( 'NONE',  ( 23.37981185087573976, -29.75599608462244561, -21.51565039292758286 ) ) ;
#32647=B_SPLINE_CURVE_WITH_KNOTS ( 'NONE', 3,
 ( #81791, #36301, #161656, #159648, #50501, #66648, #190010, #145478 ),
 .UNSPECIFIED., .F., .F.,
 ( 4, 2, 2, 4 ),
 ( 2.775519118949223281E-07, 0.0006604899437673964792, 0.0009905961396951489494, 0.001320702335622901420 ),
 .UNSPECIFIED. ) ;
#32689=CARTESIAN_POINT ( 'NONE',  ( 6.293264767923585801, -0.7627558185761198484, -62.46802126132829613 ) ) ;
#32734=CARTESIAN_POINT ( 'NONE',  ( -20.29917818118329720, -22.40963075479333355, -51.18760544280081604 ) ) ;
#32770=ORIENTED_EDGE ( 'NONE', *, *, #183088, .F. ) ;
#32785=CARTESIAN_POINT ( 'NONE',  ( -24.54856932377555268, -28.36614238946897970, -18.58410241722922862 ) ) ;
#32808=EDGE_CURVE ( 'NONE', #36107, #119352, #95152, .T. ) ;
#32809=CARTESIAN_POINT ( 'NONE',  ( 38.00000000000000000, -12.34694845685040754, -9.099999999999999645 ) ) ;
#32826=LINE ( 'NONE', #141972, #136799 ) ;
#32836=CARTESIAN_POINT ( 'NONE',  ( 36.91746825000000598, -11.99521256947793546, -5.724999997268813701 ) ) ;
#32846=CARTESIAN_POINT ( 'NONE',  ( 18.08554851550187337, -38.44972689946076372, -20.08432885666353229 ) ) ;
#32865=EDGE_LOOP ( 'NONE', ( #20596, #55441, #88903, #13254 ) ) ;
#32893=CARTESIAN_POINT ( 'NONE',  ( -16.46419947420532282, -17.59054176770899147, -54.38591257391895795 ) ) ;
#32930=LINE ( 'NONE', #29952, #40231 ) ;
#32959=EDGE_CURVE ( 'NONE', #141549, #94189, #180925, .T. ) ;
#32963=ORIENTED_EDGE ( 'NONE', *, *, #43025, .F. ) ;
#33040=CARTESIAN_POINT ( 'NONE',  ( -38.00000000000000711, 2.428612866367529932E-14, -6.000000000000000000 ) ) ;
#33060=FACE_BOUND ( 'NONE', #127771, .T. ) ;
#33074=ORIENTED_EDGE ( 'NONE', *, *, #173264, .T. ) ;
#33076=DIRECTION ( 'NONE',  ( 0.000000000000000000, -1.000000000000000000, 0.000000000000000000 ) ) ;
#33080=CARTESIAN_POINT ( 'NONE',  ( 29.86685920354754487, 21.69954338932564752, -7.924999997268814766 ) ) ;
#33130=CARTESIAN_POINT ( 'NONE',  ( 11.40812507854755253, -35.11059874428192273, -2.524999997268813523 ) ) ;
#33131=CARTESIAN_POINT ( 'NONE',  ( -22.68575836265095447, 20.56805782000746063, -50.73663675503804882 ) ) ;
#33218=LINE ( 'NONE', #126212, #150060 ) ;
#33258=CARTESIAN_POINT ( 'NONE',  ( 0.9274610294345855266, 6.404617898468148773, -62.44543528848620895 ) ) ;
#33282=CARTESIAN_POINT ( 'NONE',  ( -24.30000000000003268, 2.668083032619853614E-13, -54.21489346206828230 ) ) ;
#33297=CARTESIAN_POINT ( 'NONE',  ( 0.000000000000000000, 0.000000000000000000, -65.00100000000003320 ) ) ;
#33317=CARTESIAN_POINT ( 'NONE',  ( -38.00000000000000711, 2.428612866367529932E-14, -1.749999994537626558 ) ) ;
#33349=EDGE_LOOP ( 'NONE', ( #103795, #87497, #161848, #120277 ) ) ;
#33399=ADVANCED_FACE ( 'NONE', ( #199820 ), #188873, .F. ) ;
#33415=CARTESIAN_POINT ( 'NONE',  ( -16.38029848613151174, 0.9460486868806974314, -61.48057501744757758 ) ) ;
#33435=CARTESIAN_POINT ( 'NONE',  ( 11.30153831258471797, -180.0000000000000000, -15.00000000000000178 ) ) ;
#33450=CARTESIAN_POINT ( 'NONE',  ( -6.328208617727321794, -6.541134799867854177, -61.89430850415823215 ) ) ;
#33456=CIRCLE ( 'NONE', #59153, 16.70000000000002061 ) ;
#33479=CARTESIAN_POINT ( 'NONE',  ( -9.441188956457237325, -38.26011958722978079, -31.87100816096939582 ) ) ;
#33527=ORIENTED_EDGE ( 'NONE', *, *, #132358, .F. ) ;
#33545=CIRCLE ( 'NONE', #136886, 31.90000000000003411 ) ;
#33562=CARTESIAN_POINT ( 'NONE',  ( 4.215739103160468737, -48.58376198229545651, -25.00000000000000711 ) ) ;
#33607=CARTESIAN_POINT ( 'NONE',  ( 19.06840828308530433, -32.80151167437067983, -20.74459427420917379 ) ) ;
#33636=ORIENTED_EDGE ( 'NONE', *, *, #6795, .T. ) ;
#33644=DIRECTION ( 'NONE',  ( -1.000000000000000000, -1.071875439572228152E-15, -5.204170427930421283E-16 ) ) ;
#33672=CARTESIAN_POINT ( 'NONE',  ( 9.021779378622690970, -0.4881926659581901640, -61.91041879129569026 ) ) ;
#33762=ORIENTED_EDGE ( 'NONE', *, *, #94686, .F. ) ;
#33774=CARTESIAN_POINT ( 'NONE',  ( -31.47295357026017726, -21.29310327862334518, -24.13113353489229596 ) ) ;
#33796=CARTESIAN_POINT ( 'NONE',  ( -11.74264578624799782, -36.14014761921581709, -9.600000000000001421 ) ) ;
#33804=CARTESIAN_POINT ( 'NONE',  ( 21.56593590501845981, -19.98930001671141454, -52.11784087944676003 ) ) ;
#33822=CARTESIAN_POINT ( 'NONE',  ( -36.91746825000001309, -11.99521256947794789, -6.524999997268810858 ) ) ;
#33832=CARTESIAN_POINT ( 'NONE',  ( 14.22875182907821490, -42.06737590809383676, -22.02417070750506412 ) ) ;
#33886=CARTESIAN_POINT ( 'NONE',  ( -22.81625015709509441, -31.40387420917324590, -8.824999997268811569 ) ) ;
#33921=DIRECTION ( 'NONE',  ( -1.000000000000000000, 0.000000000000000000, 0.000000000000000000 ) ) ;
#33952=ORIENTED_EDGE ( 'NONE', *, *, #183981, .F. ) ;
#34012=AXIS2_PLACEMENT_3D ( 'NONE', #35382, #22208, #49560 ) ;
#34035=VECTOR ( 'NONE', #63909, 1000.000000000000000 ) ;
#34049=CARTESIAN_POINT ( 'NONE',  ( 1.500000000000347500, 7.793921569590667175, -62.16239983623972165 ) ) ;
#34052=CYLINDRICAL_SURFACE ( 'NONE', #54020, 1.499999999999997780 ) ;
#34067=ORIENTED_EDGE ( 'NONE', *, *, #182492, .F. ) ;
#34072=CARTESIAN_POINT ( 'NONE',  ( -22.81625015709509441, -31.40387420917324590, -8.824999997268811569 ) ) ;
#34084=CARTESIAN_POINT ( 'NONE',  ( 6.434671708797586653, 6.434671708797580436, -61.89430850415821794 ) ) ;
#34121=CARTESIAN_POINT ( 'NONE',  ( -11.40812507854754720, -35.11059874428192273, -6.724999997268813701 ) ) ;
#34129=CARTESIAN_POINT ( 'NONE',  ( 18.83841601638290086, -33.00795687112466936, -25.49111855720866160 ) ) ;
#34208=DIRECTION ( 'NONE',  ( -0.000000000000000000, 0.000000000000000000, 1.000000000000000000 ) ) ;
#34229=CARTESIAN_POINT ( 'NONE',  ( -69.65682714487590488, -71.74905178543390605, -10.00000000000000000 ) ) ;
#34268=DIRECTION ( 'NONE',  ( 1.000000000000000000, 0.000000000000000000, 0.000000000000000000 ) ) ;
#34290=DIRECTION ( 'NONE',  ( 0.000000000000000000, 0.000000000000000000, 1.000000000000000000 ) ) ;
#34308=CARTESIAN_POINT ( 'NONE',  ( 30.74264578624800137, -22.33583958711395212, -2.949999994537626957 ) ) ;
#34318=CARTESIAN_POINT ( 'NONE',  ( 21.65131445265850729, -0.9841389949901845347, -58.61993113718296655 ) ) ;
#34320=CARTESIAN_POINT ( 'NONE',  ( -1.468823602708420273, -30.74735067906812702, -50.54421433284817056 ) ) ;
#34336=AXIS2_PLACEMENT_3D ( 'NONE', #9187, #40513, #160858 ) ;
#34342=VERTEX_POINT ( 'NONE', #62029 ) ;
#34399=CARTESIAN_POINT ( 'NONE',  ( -26.46959431505283789, -27.26463967846487435, -15.00000000000000178 ) ) ;
#34401=DIRECTION ( 'NONE',  ( 1.000000000000000000, 0.000000000000000000, -0.000000000000000000 ) ) ;
#34409=CARTESIAN_POINT ( 'NONE',  ( -15.29519331188519082, 1.499966876286098927, -61.92990168432675091 ) ) ;
#34443=CARTESIAN_POINT ( 'NONE',  ( 4.000000000000000888, -105.0000000000000000, -23.00000000000000000 ) ) ;
#34471=CARTESIAN_POINT ( 'NONE',  ( -2.802625768539467543, -39.09149893265183806, -33.00000000000000000 ) ) ;
#34522=ORIENTED_EDGE ( 'NONE', *, *, #30897, .T. ) ;
#34534=CARTESIAN_POINT ( 'NONE',  ( 14.46726734353924648, -1.322814319813029993, -62.26916108939695960 ) ) ;
#34564=FACE_BOUND ( 'NONE', #47532, .T. ) ;
#34600=CARTESIAN_POINT ( 'NONE',  ( 26.28653040952099218, -27.04268878403684084, -20.33571853020390208 ) ) ;
#34604=VERTEX_POINT ( 'NONE', #124708 ) ;
#34635=DIRECTION ( 'NONE',  ( -1.084202172485503448E-15, 1.000000000000000000, 0.000000000000000000 ) ) ;
#34666=CARTESIAN_POINT ( 'NONE',  ( 8.724588103088175117, -0.9974278668897691436, -61.97156292062779670 ) ) ;
#34676=CARTESIAN_POINT ( 'NONE',  ( 0.000000000000000000, -64.82615989628266107, -23.00000000000000000 ) ) ;
#34682=EDGE_CURVE ( 'NONE', #25217, #173153, #195377, .T. ) ;
#34710=CARTESIAN_POINT ( 'NONE',  ( -28.98447489709222680, -24.58636592488624117, -17.12158557651119750 ) ) ;
#34712=CARTESIAN_POINT ( 'NONE',  ( -5.000000000000003553, 37.66961640367474473, -15.00000000000000000 ) ) ;
#34746=ORIENTED_EDGE ( 'NONE', *, *, #70721, .T. ) ;
#34757=AXIS2_PLACEMENT_3D ( 'NONE', #66686, #190046, #97991 ) ;
#34762=EDGE_CURVE ( 'NONE', #126376, #111207, #124333, .T. ) ;
#34764=CARTESIAN_POINT ( 'NONE',  ( -31.56233167169803622, -22.40491105029811081, -17.28239568967446971 ) ) ;
#34776=EDGE_CURVE ( 'NONE', #130796, #45831, #1351, .T. ) ;
#34783=AXIS2_PLACEMENT_3D ( 'NONE', #1746, #108929, #154442 ) ;
#34787=CARTESIAN_POINT ( 'NONE',  ( -30.59399807301414498, 1.495846735942831351, -47.49088840515941001 ) ) ;
#34809=EDGE_LOOP ( 'NONE', ( #51909, #180120, #35049, #99705, #63 ) ) ;
#34811=CARTESIAN_POINT ( 'NONE',  ( 29.86685920354754842, -21.69954338932559068, -3.824999997268813345 ) ) ;
#34821=CARTESIAN_POINT ( 'NONE',  ( 15.50653001718876745, -40.92458772717220228, -21.39878705119478042 ) ) ;
#34868=CARTESIAN_POINT ( 'NONE',  ( -15.72645790992315717, -17.57596900401679818, -54.79584306608744271 ) ) ;
#34872=CARTESIAN_POINT ( 'NONE',  ( -5.950531402560715689E-15, 38.81732327939063509, -1.124999997268812946 ) ) ;
#34928=EDGE_CURVE ( 'NONE', #103031, #128045, #91988, .T. ) ;
#34931=CARTESIAN_POINT ( 'NONE',  ( -19.38985940809734032, -32.68077955211932561, -25.00000000000009592 ) ) ;
#34935=CIRCLE ( 'NONE', #112429, 38.00000000000000000 ) ;
#35049=ORIENTED_EDGE ( 'NONE', *, *, #82833, .F. ) ;
#35051=ORIENTED_EDGE ( 'NONE', *, *, #181354, .T. ) ;
#35053=CARTESIAN_POINT ( 'NONE',  ( 15.06137443927351249, -15.06137443927345210, -64.92279855667830191 ) ) ;
#35057=CARTESIAN_POINT ( 'NONE',  ( -29.86685920354755552, 21.69954338932564397, -7.324999997268814234 ) ) ;
#35092=B_SPLINE_CURVE_WITH_KNOTS ( 'NONE', 3,
 ( #84852, #173908, #53530, #35377, #116208, #66703, #68695, #115208, #176900, #70710, #132378, #174891, #193058, #160712, #145534, #194072, #162711, #97029, #24216, #55533, #20199, #147554 ),
 .UNSPECIFIED., .F., .F.,
 ( 4, 2, 2, 2, 2, 2, 2, 2, 2, 2, 4 ),
 ( 2.787258305036405189E-07, 0.0003055402697144840151, 0.0006108018135984643248, 0.001221324901366421800, 0.001831847989134385022, 0.002137109533018368909, 0.002442371076902352580, 0.003052894164670316886, 0.003663417252438281192, 0.004273940340206244630, 0.004884463427974209369 ),
 .UNSPECIFIED. ) ;
#35104=DIRECTION ( 'NONE',  ( -0.000000000000000000, -0.000000000000000000, -1.000000000000000000 ) ) ;
#35107=CARTESIAN_POINT ( 'NONE',  ( 11.40812507854754365, 35.11059874428196537, -1.724999997268813479 ) ) ;
#35114=CYLINDRICAL_SURFACE ( 'NONE', #14428, 1.500000000000001332 ) ;
#35183=ORIENTED_EDGE ( 'NONE', *, *, #161479, .F. ) ;
#35246=B_SPLINE_CURVE_WITH_KNOTS ( 'NONE', 3,
 ( #47320, #34129, #110957, #1793, #93801, #111956, #63471, #125146, #186845, #95788, #157474, #65447, #18967, #143271, #48314, #80613 ),
 .UNSPECIFIED., .F., .F.,
 ( 4, 2, 2, 2, 2, 2, 2, 4 ),
 ( 0.02045126265315338338, 0.02288269579900681361, 0.02531412894486024384, 0.03017699523656709737, 0.03260842838242052066, 0.03382414495534723231, 0.03503986152827393008, 0.03990272781998075585 ),
 .UNSPECIFIED. ) ;
#35291=CARTESIAN_POINT ( 'NONE',  ( 30.12056840655111856, -26.02156742258010880, -20.94459150989510476 ) ) ;
#35293=EDGE_CURVE ( 'NONE', #22185, #6817, #160018, .T. ) ;
#35308=LINE ( 'NONE', #190986, #198579 ) ;
#35354=CARTESIAN_POINT ( 'NONE',  ( -0.2682394567894307302, -31.88110949919181181, -45.67705988491092484 ) ) ;
#35365=CARTESIAN_POINT ( 'NONE',  ( -8.817897698975500020, -38.37206457205380161, -32.07286502659091809 ) ) ;
#35366=ORIENTED_EDGE ( 'NONE', *, *, #152623, .T. ) ;
#35377=CARTESIAN_POINT ( 'NONE',  ( 9.438666190699255054, 10.00917710959072160, -62.55979675456843836 ) ) ;
#35382=CARTESIAN_POINT ( 'NONE',  ( -3.573655867282028392E-15, 2.428612866367529932E-14, -25.00000000000000000 ) ) ;
#35397=CARTESIAN_POINT ( 'NONE',  ( -15.01118352434399483, 1.500065973499320027, -62.04667436142315751 ) ) ;
#35429=CYLINDRICAL_SURFACE ( 'NONE', #109809, 1.499999999999997780 ) ;
#35493=LINE ( 'NONE', #97143, #74187 ) ;
#35552=FACE_BOUND ( 'NONE', #163398, .T. ) ;
#35557=CARTESIAN_POINT ( 'NONE',  ( -15.92681084339657716, 1.315686079477422554, -59.47631410104521166 ) ) ;
#35567=CARTESIAN_POINT ( 'NONE',  ( 3.766062262543149401E-15, -39.95556452105413570, -9.500000000000001776 ) ) ;
#35576=AXIS2_PLACEMENT_3D ( 'NONE', #85517, #100683, #107648 ) ;
#35617=EDGE_LOOP ( 'NONE', ( #88053, #55741, #147933, #197719 ) ) ;
#35703=CARTESIAN_POINT ( 'NONE',  ( -19.99604614807126524, -21.49604614807087799, -52.16759353428663104 ) ) ;
#35754=CARTESIAN_POINT ( 'NONE',  ( -25.38628342471223576, -27.91043139587360145, -20.44818103819420330 ) ) ;
#35769=VERTEX_POINT ( 'NONE', #89167 ) ;
#35783=LINE ( 'NONE', #110632, #8068 ) ;
#35799=ORIENTED_EDGE ( 'NONE', *, *, #47298, .T. ) ;
#35801=CARTESIAN_POINT ( 'NONE',  ( -29.86685920354755552, 21.69954338932564397, -4.824999997268814234 ) ) ;
#35811=CARTESIAN_POINT ( 'NONE',  ( 21.89035704508949465, -33.26311937565159127, -20.38189100991405311 ) ) ;
#35858=VERTEX_POINT ( 'NONE', #8341 ) ;
#35863=CARTESIAN_POINT ( 'NONE',  ( -36.91746825000001309, 11.99521256947798342, -9.224999997268813701 ) ) ;
#35894=EDGE_CURVE ( 'NONE', #114764, #144280, #118527, .T. ) ;
#35896=CARTESIAN_POINT ( 'NONE',  ( 12.24802307403557933, -10.74802307403627921, -61.53034260416801260 ) ) ;
#35897=DIRECTION ( 'NONE',  ( -0.000000000000000000, -0.000000000000000000, -1.000000000000000000 ) ) ;
#35973=EDGE_LOOP ( 'NONE', ( #167141, #159163, #107902, #109361, #191043, #43991 ) ) ;
#36005=CARTESIAN_POINT ( 'NONE',  ( 21.51934928555110460, 22.99905646750775290, -46.25979504214461713 ) ) ;
#36020=CARTESIAN_POINT ( 'NONE',  ( 0.9909172445849734334, 21.65732038466284948, -56.20941306831223727 ) ) ;
#36029=CARTESIAN_POINT ( 'NONE',  ( 11.80868324581537543, 11.80868324581533990, -59.13370768023891344 ) ) ;
#36031=CARTESIAN_POINT ( 'NONE',  ( -22.81625015709509441, -31.40387420917324590, -4.324999997268813345 ) ) ;
#36045=CARTESIAN_POINT ( 'NONE',  ( 22.81625015709509441, 31.40387420917330275, -7.824999997268813345 ) ) ;
#36092=CARTESIAN_POINT ( 'NONE',  ( -11.40812507854754720, -35.11059874428192273, -4.724999997268812812 ) ) ;
#36107=VERTEX_POINT ( 'NONE', #56852 ) ;
#36131=ADVANCED_FACE ( 'NONE', ( #38683 ), #102348, .T. ) ;
#36208=ORIENTED_EDGE ( 'NONE', *, *, #79274, .F. ) ;
#36235=CARTESIAN_POINT ( 'NONE',  ( -3.503282210674343311, -48.86437366581480291, -22.99999999999999645 ) ) ;
#36241=CARTESIAN_POINT ( 'NONE',  ( -1.491051326732881099, -15.38891197842626468, -61.89130710690760395 ) ) ;
#36257=CARTESIAN_POINT ( 'NONE',  ( 17.62203461105334767, -16.12203461105336189, -54.55577602037946150 ) ) ;
#36261=CARTESIAN_POINT ( 'NONE',  ( 10.74802307403555268, -10.74802307403551715, -64.92279855667830191 ) ) ;
#36272=CARTESIAN_POINT ( 'NONE',  ( 28.45933917494778953, -27.69424206401129851, -20.18904788101062664 ) ) ;
#36285=FACE_OUTER_BOUND ( 'NONE', #152991, .T. ) ;
#36301=CARTESIAN_POINT ( 'NONE',  ( -20.27679576775602754, -20.59397618482648440, -49.67367017693150189 ) ) ;
#36328=ORIENTED_EDGE ( 'NONE', *, *, #72845, .F. ) ;
#36345=CARTESIAN_POINT ( 'NONE',  ( -22.02428569922414781, -33.37003842005439935, -23.53509012974684111 ) ) ;
#36400=CARTESIAN_POINT ( 'NONE',  ( -19.38985940809734032, -32.68077955211932561, -25.00000000000009592 ) ) ;
#36409=CARTESIAN_POINT ( 'NONE',  ( -4.287918369368176386, -6.449379854004495982, -62.20361152659754111 ) ) ;
#36413=CARTESIAN_POINT ( 'NONE',  ( 37.99999999999999289, 2.428612866367529932E-14, -25.00000000000000000 ) ) ;
#36474=CARTESIAN_POINT ( 'NONE',  ( -17.06285122369598284, -17.30253834197026919, -56.77278709839600879 ) ) ;
#36490=EDGE_LOOP ( 'NONE', ( #115957, #52747, #47800, #119586 ) ) ;
#36523=AXIS2_PLACEMENT_3D ( 'NONE', #14685, #155180, #78319 ) ;
#36539=DIRECTION ( 'NONE',  ( 0.000000000000000000, 0.000000000000000000, -1.000000000000000000 ) ) ;
#36546=VERTEX_POINT ( 'NONE', #155597 ) ;
#36550=AXIS2_PLACEMENT_3D ( 'NONE', #190587, #37901, #145063 ) ;
#36560=VERTEX_POINT ( 'NONE', #154602 ) ;
#36572=EDGE_CURVE ( 'NONE', #41844, #115644, #112151, .T. ) ;
#36574=DIRECTION ( 'NONE',  ( 0.000000000000000000, 0.000000000000000000, 1.000000000000000000 ) ) ;
#36601=ORIENTED_EDGE ( 'NONE', *, *, #48904, .F. ) ;
#36635=PLANE ( 'NONE',  #178759 ) ;
#36648=EDGE_CURVE ( 'NONE', #130499, #75168, #127503, .T. ) ;
#36684=CARTESIAN_POINT ( 'NONE',  ( 9.562403590618709259, 11.67169337655810502, -59.87610203618464766 ) ) ;
#36716=B_SPLINE_CURVE_WITH_KNOTS ( 'NONE', 3,
 ( #198930, #48232, #1712, #155403, #105912, #30073, #152415, #185748, #31071, #13903, #17897, #707, #122070, #107887, #14906, #183762, #109887, #167598, #29093, #90732, #169574, #154408, #15902, #16893 ),
 .UNSPECIFIED., .F., .F.,
 ( 4, 2, 2, 2, 2, 2, 2, 2, 2, 2, 2, 4 ),
 ( 1.970462154302192724E-07, 0.0003069708713091119884, 0.0006137446964027936649, 0.001227292346590153549, 0.001534066171683836580, 0.001840839996777519178, 0.002147613821871202210, 0.002454387646964885459, 0.003067935297152254558, 0.003681482947339624525, 0.004295030597526993191, 0.004908578247714363157 ),
 .UNSPECIFIED. ) ;
#36728=ORIENTED_EDGE ( 'NONE', *, *, #111893, .F. ) ;
#36738=CARTESIAN_POINT ( 'NONE',  ( -29.42957871419942961, -23.46871120497985785, -19.15262919804619557 ) ) ;
#36755=AXIS2_PLACEMENT_3D ( 'NONE', #5691, #84520, #24887 ) ;
#36765=LINE ( 'NONE', #101437, #153154 ) ;
#36779=AXIS2_PLACEMENT_3D ( 'NONE', #50383, #158537, #22024 ) ;
#36787=CARTESIAN_POINT ( 'NONE',  ( 3.556970738554033499E-15, -38.81732327939057825, -4.124999997268814056 ) ) ;
#36798=CARTESIAN_POINT ( 'NONE',  ( 30.11221142034223419, -26.30828378221802666, -17.15571736052815410 ) ) ;
#36817=ORIENTED_EDGE ( 'NONE', *, *, #76459, .T. ) ;
#36836=DIRECTION ( 'NONE',  ( -0.000000000000000000, 0.000000000000000000, 1.000000000000000000 ) ) ;
#36846=DIRECTION ( 'NONE',  ( 0.000000000000000000, 0.000000000000000000, 1.000000000000000000 ) ) ;
#36849=CARTESIAN_POINT ( 'NONE',  ( 36.91746824999999177, 2.880721459617395097E-14, -1.624999997268813390 ) ) ;
#36863=ORIENTED_EDGE ( 'NONE', *, *, #90031, .F. ) ;
#36885=CARTESIAN_POINT ( 'NONE',  ( 31.42649584489977244, -1.097581692000379583, -49.72218688481374471 ) ) ;
#36896=AXIS2_PLACEMENT_3D ( 'NONE', #118637, #180329, #17408 ) ;
#36987=ORIENTED_EDGE ( 'NONE', *, *, #76762, .F. ) ;
#36990=AXIS2_PLACEMENT_3D ( 'NONE', #84875, #24243, #130374 ) ;
#37017=CARTESIAN_POINT ( 'NONE',  ( -30.65641173115115947, -25.45263461537911098, -21.37460845010010146 ) ) ;
#37018=CARTESIAN_POINT ( 'NONE',  ( 0.4369134036781218144, 21.36090571693007334, -56.42503783362397485 ) ) ;
#37021=FACE_BOUND ( 'NONE', #112637, .T. ) ;
#37027=DIRECTION ( 'NONE',  ( -0.000000000000000000, -0.000000000000000000, 1.000000000000000000 ) ) ;
#37029=CARTESIAN_POINT ( 'NONE',  ( 11.40812507854754365, 35.11059874428196537, -5.224999997268813701 ) ) ;
#37037=VECTOR ( 'NONE', #118877, 1000.000000000000000 ) ;
#37038=EDGE_LOOP ( 'NONE', ( #35366, #25455, #100433, #167919, #52391 ) ) ;
#37093=CARTESIAN_POINT ( 'NONE',  ( -20.83652723102587245, 20.12987255291484345, -52.58065409862962269 ) ) ;
#37197=EDGE_CURVE ( 'NONE', #147808, #22341, #66563, .T. ) ;
#37219=VECTOR ( 'NONE', #80563, 1000.000000000000000 ) ;
#37222=CARTESIAN_POINT ( 'NONE',  ( -15.70878279763969765, 14.67621740152104870, -56.33456566391307518 ) ) ;
#37240=CARTESIAN_POINT ( 'NONE',  ( -6.907351198298408157, -38.20768336775255136, -23.99027881317066857 ) ) ;
#37246=CARTESIAN_POINT ( 'NONE',  ( -1.464556741314096966, -14.82342540975557021, -62.12362001602810579 ) ) ;
#37262=CARTESIAN_POINT ( 'NONE',  ( 17.46158047089203791, -15.43343858725516426, -55.01551020149706517 ) ) ;
#37276=ORIENTED_EDGE ( 'NONE', *, *, #14918, .F. ) ;
#37279=DIRECTION ( 'NONE',  ( 1.000000000000000000, 0.000000000000000000, 0.000000000000000000 ) ) ;
#37281=CARTESIAN_POINT ( 'NONE',  ( -38.00000000000001421, -12.34694845685042708, -3.649999994537627135 ) ) ;
#37292=DIRECTION ( 'NONE',  ( -0.000000000000000000, -0.000000000000000000, 1.000000000000000000 ) ) ;
#37295=CARTESIAN_POINT ( 'NONE',  ( 26.88621168971713615, -26.45719545518169014, -20.39628335082762334 ) ) ;
#37310=VECTOR ( 'NONE', #105213, 1000.000000000000000 ) ;
#37331=DIRECTION ( 'NONE',  ( 0.000000000000000000, 0.000000000000000000, 1.000000000000000000 ) ) ;
#37334=CIRCLE ( 'NONE', #124515, 28.90000000000004476 ) ;
#37339=CARTESIAN_POINT ( 'NONE',  ( -1.249513161672007433, -29.56482114129871519, -48.84067647644814514 ) ) ;
#37345=ORIENTED_EDGE ( 'NONE', *, *, #110412, .T. ) ;
#37351=FACE_OUTER_BOUND ( 'NONE', #13676, .T. ) ;
#37363=CARTESIAN_POINT ( 'NONE',  ( -10.59477242850411649, -90.60836494048552936, -25.00000000000000000 ) ) ;
#37380=CARTESIAN_POINT ( 'NONE',  ( 6.434671708797603529, -6.434671708797564449, -61.89430850415821794 ) ) ;
#37462=EDGE_CURVE ( 'NONE', #154699, #126159, #6873, .T. ) ;
#37500=ORIENTED_EDGE ( 'NONE', *, *, #14301, .T. ) ;
#37515=AXIS2_PLACEMENT_3D ( 'NONE', #125327, #2966, #3948 ) ;
#37517=CARTESIAN_POINT ( 'NONE',  ( 14.01879992551668863, -0.9453496423219486244, -62.45159313300391091 ) ) ;
#37542=CARTESIAN_POINT ( 'NONE',  ( -30.74264578624800492, -22.33583958711396278, -5.549999994537627046 ) ) ;
#37553=VECTOR ( 'NONE', #181340, 1000.000000000000000 ) ;
#37582=EDGE_LOOP ( 'NONE', ( #14136, #9844, #60722, #185549, #37276 ) ) ;
#37584=CARTESIAN_POINT ( 'NONE',  ( 30.69486229629358576, -23.16037512311203272, -17.06287707314307411 ) ) ;
#37689=DIRECTION ( 'NONE',  ( -0.000000000000000000, -0.000000000000000000, 1.000000000000000000 ) ) ;
#37692=LINE ( 'NONE', #132706, #147502 ) ;
#37736=ADVANCED_FACE ( 'NONE', ( #39224 ), #100880, .F. ) ;
#37777=CARTESIAN_POINT ( 'NONE',  ( 4.458020396767582660, 6.565813341170965600, -64.20492216656606388 ) ) ;
#37800=CARTESIAN_POINT ( 'NONE',  ( 11.74264578624799427, 36.14014761921585972, -0.5999999999999999778 ) ) ;
#37807=EDGE_CURVE ( 'NONE', #38805, #101645, #68827, .T. ) ;
#37821=ADVANCED_FACE ( 'NONE', ( #197900 ), #133225, .F. ) ;
#37833=ORIENTED_EDGE ( 'NONE', *, *, #143190, .F. ) ;
#37849=VECTOR ( 'NONE', #114087, 1000.000000000000000 ) ;
#37853=DIRECTION ( 'NONE',  ( 1.000000000000000000, 0.000000000000000000, 0.000000000000000000 ) ) ;
#37866=CARTESIAN_POINT ( 'NONE',  ( -11.40812507854754720, -35.11059874428192273, -2.224999997268813701 ) ) ;
#37901=DIRECTION ( 'NONE',  ( 6.391086490440868450E-16, -1.000000000000000000, 0.000000000000000000 ) ) ;
#37922=CARTESIAN_POINT ( 'NONE',  ( 28.90000000000004476, -9.625633623500122352E-14, -64.92279855667830191 ) ) ;
#37931=ORIENTED_EDGE ( 'NONE', *, *, #39985, .F. ) ;
#37941=B_SPLINE_CURVE_WITH_KNOTS ( 'NONE', 3,
 ( #112697, #141054, #159191, #83350, #110711, #145026, #52024, #109723, #34868, #4506, #2540, #32893, #144031, #111711, #157227, #172393 ),
 .UNSPECIFIED., .F., .F.,
 ( 4, 2, 2, 2, 2, 2, 2, 4 ),
 ( 0.001225964299381153508, 0.002243048150408413245, 0.002751590075922042029, 0.003260132001435670814, 0.003768673926949299598, 0.004277215852462927514, 0.004785757777976557166, 0.005294299703490185083 ),
 .UNSPECIFIED. ) ;
#37950=AXIS2_PLACEMENT_3D ( 'NONE', #11450, #104437, #137743 ) ;
#37976=VECTOR ( 'NONE', #50487, 1000.000000000000000 ) ;
#37993=AXIS2_PLACEMENT_3D ( 'NONE', #73609, #43256, #9937 ) ;
#38016=CARTESIAN_POINT ( 'NONE',  ( 20.99774934350697109, 22.92000981050135877, -46.85949206705566183 ) ) ;
#38026=LINE ( 'NONE', #97663, #62869 ) ;
#38040=DIRECTION ( 'NONE',  ( -0.000000000000000000, -0.000000000000000000, 1.000000000000000000 ) ) ;
#38042=CARTESIAN_POINT ( 'NONE',  ( 11.40812507854754365, 35.11059874428196537, -3.224999997268813701 ) ) ;
#38086=CIRCLE ( 'NONE', #31592, 21.30000000000002913 ) ;
#38101=CARTESIAN_POINT ( 'NONE',  ( 29.79829367730021872, -1.376802789500971347, -48.54110828511540632 ) ) ;
#38105=CARTESIAN_POINT ( 'NONE',  ( -22.55670631985092456, 22.55670631985084995, -49.13275782002545355 ) ) ;
#38121=EDGE_LOOP ( 'NONE', ( #191720, #79259, #33762, #109984, #5698, #146204 ) ) ;
#38175=EDGE_LOOP ( 'NONE', ( #67663, #43732, #128356, #192810 ) ) ;
#38213=CARTESIAN_POINT ( 'NONE',  ( -38.00000000000000711, 2.428612866367529932E-14, -1.749999994537626558 ) ) ;
#38247=CARTESIAN_POINT ( 'NONE',  ( -7.282160400437569514, -46.44936954762594183, -22.53643251332787756 ) ) ;
#38270=CARTESIAN_POINT ( 'NONE',  ( -30.74735067906812702, 1.468823602708742238, -50.54421433284819898 ) ) ;
#38286=DIRECTION ( 'NONE',  ( 0.000000000000000000, 0.000000000000000000, 1.000000000000000000 ) ) ;
#38288=CARTESIAN_POINT ( 'NONE',  ( -38.00000000000000711, 2.428612866367529932E-14, -5.749999994537626336 ) ) ;
#38297=DIRECTION ( 'NONE',  ( 0.000000000000000000, 0.000000000000000000, 1.000000000000000000 ) ) ;
#38301=DIRECTION ( 'NONE',  ( 0.000000000000000000, 0.000000000000000000, 1.000000000000000000 ) ) ;
#38304=ORIENTED_EDGE ( 'NONE', *, *, #77897, .T. ) ;
#38305=CARTESIAN_POINT ( 'NONE',  ( 25.65937876999948841, -27.64914803190701420, -20.38451907593468349 ) ) ;
#38359=CARTESIAN_POINT ( 'NONE',  ( -4.755560754640141496, -48.37114524154433326, -24.99999999999999289 ) ) ;
#38360=ORIENTED_EDGE ( 'NONE', *, *, #198190, .F. ) ;
#38431=LINE ( 'NONE', #100087, #97070 ) ;
#38432=EDGE_CURVE ( 'NONE', #89770, #142110, #98784, .T. ) ;
#38458=CARTESIAN_POINT ( 'NONE',  ( 4.313351365237961588, -4.313351365237934054, -62.50719930893269805 ) ) ;
#38510=ORIENTED_EDGE ( 'NONE', *, *, #48810, .T. ) ;
#38514=ORIENTED_EDGE ( 'NONE', *, *, #166752, .F. ) ;
#38569=ORIENTED_EDGE ( 'NONE', *, *, #170098, .T. ) ;
#38581=ORIENTED_EDGE ( 'NONE', *, *, #76696, .T. ) ;
#38592=DIRECTION ( 'NONE',  ( 1.000000000000000000, 1.776356839400250465E-15, 0.000000000000000000 ) ) ;
#38595=CARTESIAN_POINT ( 'NONE',  ( 30.24683373042637768, -22.89668476416391485, -22.64123003231907205 ) ) ;
#38599=ORIENTED_EDGE ( 'NONE', *, *, #34776, .F. ) ;
#38619=CARTESIAN_POINT ( 'NONE',  ( -11.80868324581538253, 11.80868324581533457, -59.13370768023891344 ) ) ;
#38625=CIRCLE ( 'NONE', #103159, 10.00000000000000000 ) ;
#38655=CYLINDRICAL_SURFACE ( 'NONE', #81573, 59.99999999999998579 ) ;
#38659=DIRECTION ( 'NONE',  ( -1.000000000000000000, -1.953992523340275511E-14, 0.000000000000000000 ) ) ;
#38683=FACE_OUTER_BOUND ( 'NONE', #2723, .T. ) ;
#38749=ORIENTED_EDGE ( 'NONE', *, *, #44126, .T. ) ;
#38751=ORIENTED_EDGE ( 'NONE', *, *, #78302, .T. ) ;
#38772=CIRCLE ( 'NONE', #61278, 216.0437394197456342 ) ;
#38777=VERTEX_POINT ( 'NONE', #178423 ) ;
#38788=CARTESIAN_POINT ( 'NONE',  ( -11.74264578624799782, -36.14014761921581709, -7.349999994537626868 ) ) ;
#38792=DIRECTION ( 'NONE',  ( 0.000000000000000000, 0.000000000000000000, 1.000000000000000000 ) ) ;
#38799=FACE_OUTER_BOUND ( 'NONE', #58169, .T. ) ;
#38805=VERTEX_POINT ( 'NONE', #67228 ) ;
#38808=CARTESIAN_POINT ( 'NONE',  ( 22.81625015709510151, -31.40387420917324590, -9.924999997268814766 ) ) ;
#38817=CARTESIAN_POINT ( 'NONE',  ( 28.61471831746382222, -27.54183658529444756, -20.22090314799459776 ) ) ;
#38837=ORIENTED_EDGE ( 'NONE', *, *, #52114, .F. ) ;
#38841=ADVANCED_FACE ( 'NONE', ( #175415 ), #24748, .F. ) ;
#38861=EDGE_CURVE ( 'NONE', #59419, #106915, #156968, .T. ) ;
#38869=CARTESIAN_POINT ( 'NONE',  ( 36.91746825000000598, -11.99521256947793546, -9.724999997268813701 ) ) ;
#38902=PLANE ( 'NONE',  #36550 ) ;
#38950=AXIS2_PLACEMENT_3D ( 'NONE', #9598, #11606, #56086 ) ;
#39014=DIRECTION ( 'NONE',  ( -0.000000000000000000, -0.000000000000000000, 1.000000000000000000 ) ) ;
#39023=CARTESIAN_POINT ( 'NONE',  ( -1.022580077288041090E-15, -16.70000000000002061, -59.13370768023891344 ) ) ;
#39110=CARTESIAN_POINT ( 'NONE',  ( 14.68143632974469881, 16.57870055856060887, -58.31140971112360205 ) ) ;
#39224=FACE_OUTER_BOUND ( 'NONE', #86665, .T. ) ;
#39245=CARTESIAN_POINT ( 'NONE',  ( 9.797797781461023092, -9.576928023050404803, -62.58071313852363460 ) ) ;
#39283=CARTESIAN_POINT ( 'NONE',  ( 23.48529157249600630, -32.32473071737749137, -9.049999994537627046 ) ) ;
#39292=DIRECTION ( 'NONE',  ( -0.000000000000000000, -0.000000000000000000, 1.000000000000000000 ) ) ;
#39300=CARTESIAN_POINT ( 'NONE',  ( 0.000000000000000000, 0.000000000000000000, -52.65483682830183199 ) ) ;
#39312=LINE ( 'NONE', #120140, #78770 ) ;
#39322=DIRECTION ( 'NONE',  ( -0.1178549842436472511, 0.9930308165857339997, -0.000000000000000000 ) ) ;
#39333=CARTESIAN_POINT ( 'NONE',  ( -5.950531402560715689E-15, 38.81732327939063509, -3.624999997268813168 ) ) ;
#39343=CARTESIAN_POINT ( 'NONE',  ( -1.069973119862968947, -29.34370184275725180, -49.12095057784389951 ) ) ;
#39356=CARTESIAN_POINT ( 'NONE',  ( -8.863853373469556374, -46.11448583660600065, -24.15755306339368147 ) ) ;
#39371=CARTESIAN_POINT ( 'NONE',  ( 24.28759355007372989, -0.2213677808126924551, -54.22458008397516949 ) ) ;
#39383=LINE ( 'NONE', #104054, #69481 ) ;
#39445=CARTESIAN_POINT ( 'NONE',  ( 4.647474457565486646E-15, -28.90000000000004476, -52.65483682830183199 ) ) ;
#39480=CARTESIAN_POINT ( 'NONE',  ( -17.18269478283327345, -17.18269478283298568, -56.77278709839600879 ) ) ;
#39485=EDGE_CURVE ( 'NONE', #178697, #59792, #40899, .T. ) ;
#39504=DIRECTION ( 'NONE',  ( -0.000000000000000000, -0.000000000000000000, 1.000000000000000000 ) ) ;
#39526=CARTESIAN_POINT ( 'NONE',  ( -3.573655867282028392E-15, 2.428612866367529932E-14, -24.99999999999997868 ) ) ;
#39530=CARTESIAN_POINT ( 'NONE',  ( 21.44473182883397655, 22.99799039501303355, -49.72310555961296075 ) ) ;
#39558=VERTEX_POINT ( 'NONE', #70121 ) ;
#39581=CARTESIAN_POINT ( 'NONE',  ( 0.000000000000000000, 0.000000000000000000, -56.77278709839600879 ) ) ;
#39588=VERTEX_POINT ( 'NONE', #55947 ) ;
#39646=ORIENTED_EDGE ( 'NONE', *, *, #105416, .F. ) ;
#39724=EDGE_CURVE ( 'NONE', #51296, #74939, #101479, .T. ) ;
#39732=ORIENTED_EDGE ( 'NONE', *, *, #165015, .F. ) ;
#39737=CARTESIAN_POINT ( 'NONE',  ( 23.48529157249600630, -32.32473071737748427, -3.299999999999999822 ) ) ;
#39773=DIRECTION ( 'NONE',  ( -0.000000000000000000, -0.000000000000000000, 1.000000000000000000 ) ) ;
#39794=CARTESIAN_POINT ( 'NONE',  ( 3.556970738554033499E-15, -38.81732327939057825, -8.124999997268814056 ) ) ;
#39816=ORIENTED_EDGE ( 'NONE', *, *, #130059, .F. ) ;
#39848=ORIENTED_EDGE ( 'NONE', *, *, #194281, .F. ) ;
#39853=CARTESIAN_POINT ( 'NONE',  ( -11.40812507854754720, -35.11059874428192273, -6.224999997268812812 ) ) ;
#39936=DIRECTION ( 'NONE',  ( -1.000000000000000000, 0.000000000000000000, 0.000000000000000000 ) ) ;
#39975=ORIENTED_EDGE ( 'NONE', *, *, #94686, .T. ) ;
#39985=EDGE_CURVE ( 'NONE', #142110, #69099, #82259, .T. ) ;
#39990=ORIENTED_EDGE ( 'NONE', *, *, #31579, .T. ) ;
#40017=CARTESIAN_POINT ( 'NONE',  ( -30.12056840655105461, -26.02156742258015854, -20.94459150989508345 ) ) ;
#40027=CARTESIAN_POINT ( 'NONE',  ( -11.40812507854755609, 35.11059874428196537, -3.024999997268813523 ) ) ;
#40084=CARTESIAN_POINT ( 'NONE',  ( 30.27664185797779339, -1.503321482105604456, -47.91583118997746027 ) ) ;
#40097=CARTESIAN_POINT ( 'NONE',  ( 0.000000000000000000, -64.82615989628266107, -25.00000000000000000 ) ) ;
#40099=CARTESIAN_POINT ( 'NONE',  ( 17.10449713765564184, 17.26089242801060664, -56.77278709839600879 ) ) ;
#40103=ORIENTED_EDGE ( 'NONE', *, *, #74517, .F. ) ;
#40121=VECTOR ( 'NONE', #138782, 1000.000000000000000 ) ;
#40159=ORIENTED_EDGE ( 'NONE', *, *, #55093, .F. ) ;
#40216=CARTESIAN_POINT ( 'NONE',  ( -15.81114279943209766, 14.65109730209610461, -56.29481432398279139 ) ) ;
#40231=VECTOR ( 'NONE', #78412, 1000.000000000000000 ) ;
#40237=CARTESIAN_POINT ( 'NONE',  ( -18.37348032455536639, -33.26197007281776052, -21.07589179611765928 ) ) ;
#40254=EDGE_CURVE ( 'NONE', #38777, #89664, #118443, .T. ) ;
#40267=CARTESIAN_POINT ( 'NONE',  ( 4.999999999999999112, 11.45643923738960090, -18.00000000000000000 ) ) ;
#40276=ORIENTED_EDGE ( 'NONE', *, *, #139988, .T. ) ;
#40279=DIRECTION ( 'NONE',  ( -0.000000000000000000, -0.000000000000000000, 1.000000000000000000 ) ) ;
#40283=CARTESIAN_POINT ( 'NONE',  ( -11.74264578624799782, -36.14014761921581709, -5.349999994537626868 ) ) ;
#40290=CARTESIAN_POINT ( 'NONE',  ( 6.542564195780748548, -4.422302296885995077, -62.17069030305508903 ) ) ;
#40299=VERTEX_POINT ( 'NONE', #54949 ) ;
#40300=CARTESIAN_POINT ( 'NONE',  ( -0.8894290736107403061, -29.18776880969891963, -52.33677266386638394 ) ) ;
#40333=CARTESIAN_POINT ( 'NONE',  ( -11.40812507854755609, 35.11059874428196537, -3.524999997268813523 ) ) ;
#40343=DIRECTION ( 'NONE',  ( 1.000000000000000000, 1.776356839400250465E-15, 0.000000000000000000 ) ) ;
#40350=AXIS2_PLACEMENT_3D ( 'NONE', #61043, #31715, #155050 ) ;
#40356=CARTESIAN_POINT ( 'NONE',  ( -26.35186391108957338, -29.45501048291157886, -18.59600737860424857 ) ) ;
#40366=EDGE_LOOP ( 'NONE', ( #109902, #184235, #54907, #2803 ) ) ;
#40372=CARTESIAN_POINT ( 'NONE',  ( -0.1000365528946621507, -9.100000000000004974, -63.95112321872119310 ) ) ;
#40385=VECTOR ( 'NONE', #197575, 1000.000000000000000 ) ;
#40390=AXIS2_PLACEMENT_3D ( 'NONE', #64891, #137754, #187271 ) ;
#40413=DIRECTION ( 'NONE',  ( 1.000000000000000000, 0.000000000000000000, 0.000000000000000000 ) ) ;
#40462=EDGE_CURVE ( 'NONE', #22341, #39558, #127303, .T. ) ;
#40470=DIRECTION ( 'NONE',  ( 1.000000000000000000, 1.776356839400250465E-15, 0.000000000000000000 ) ) ;
#40488=CARTESIAN_POINT ( 'NONE',  ( 11.74264578624799427, 36.14014761921585972, -6.599999999999999645 ) ) ;
#40491=CARTESIAN_POINT ( 'NONE',  ( 0.5182397417203463696, 31.81335209757180138, -45.77644358828415250 ) ) ;
#40503=EDGE_CURVE ( 'NONE', #106382, #156928, #36765, .T. ) ;
#40506=VERTEX_POINT ( 'NONE', #86279 ) ;
#40513=DIRECTION ( 'NONE',  ( -0.000000000000000000, -0.000000000000000000, -1.000000000000000000 ) ) ;
#40545=CARTESIAN_POINT ( 'NONE',  ( -22.55670631985092456, 22.55670631985084995, -49.13275782002545355 ) ) ;
#40546=CLOSED_SHELL ( 'NONE', ( #76335, #33399, #74822, #57481, #190867, #160324, #159714, #69806, #58859, #199293, #143321, #24502, #148472, #56119, #180672, #164208, #196446, #43559, #188878, #71291, #133626, #186837, #127956, #63617, #114807, #31263, #126066, #77190, #174477, #40954, #24020, #42259, #153468, #197319, #46152, #112753, #104846, #27614, #2590, #97525, #95432, #108367, #20485, #1974, #69657, #110248, #164603, #64210, #81082, #153897, #161177, #46895, #25653, #138725, #110024, #54968, #190000, #97654, #153798, #16998, #146823, #171723, #109146, #76948, #146611, #171372, #159534, #160082, #104372, #123909, #170825, #166486, #178238, #112001, #146860, #186014, #722, #21594, #149831, #95180, #103505, #13940, #10682, #85779, #196832, #61320, #185979, #187879, #179456, #99221, #98163, #122343, #24296, #161345, #99828, #166955, #160774, #27944, #42667, #79825, #51155, #188468, #64776, #28572, #75398, #134692, #88676, #184994, #37736, #152432, #104525, #132667, #161301, #159613, #122342, #160562, #144333, #128121, #112277, #74707, #99666, #36131, #91338, #76927, #159804, #191328, #50278, #180767, #74303, #185866, #37821, #54395, #97894, #144962, #137415, #175123, #31555, #22546, #162698, #124120, #158488, #131277, #25829, #65365, #94644, #45288, #113643, #182724, #38841, #185345, #30171, #153602, #189248, #190123, #124477, #190547, #130023, #5079, #86919, #24989, #23022, #193642, #106615, #40874, #6010, #27853, #113957, #130880, #16480, #62499, #128132, #155671, #194812, #157654, #89639, #74609, #170585, #107807, #113512, #173634, #115553, #97465 ) ) ;
#40547=CARTESIAN_POINT ( 'NONE',  ( -10.70204458709375395, -12.25440978676920700, -59.34122310496267261 ) ) ;
#40559=LINE ( 'NONE', #195249, #150372 ) ;
#40563=CARTESIAN_POINT ( 'NONE',  ( 9.051314012904532191, -0.3916721525565275974, -63.96062167512631191 ) ) ;
#40622=ORIENTED_EDGE ( 'NONE', *, *, #186227, .F. ) ;
#40630=EDGE_CURVE ( 'NONE', #135024, #4644, #83271, .T. ) ;
#40758=CARTESIAN_POINT ( 'NONE',  ( 1.500000000002908562, 30.39999999999990266, -50.95361246531977173 ) ) ;
#40781=DIRECTION ( 'NONE',  ( 0.000000000000000000, 0.000000000000000000, 1.000000000000000000 ) ) ;
#40805=CARTESIAN_POINT ( 'NONE',  ( -36.91746825000001309, 11.99521256947798342, -8.724999997268813701 ) ) ;
#40814=CARTESIAN_POINT ( 'NONE',  ( 32.28837973138387696, -23.54499195901921027, -23.03346093386909743 ) ) ;
#40822=PLANE ( 'NONE',  #159466 ) ;
#40827=ORIENTED_EDGE ( 'NONE', *, *, #19616, .T. ) ;
#40864=CARTESIAN_POINT ( 'NONE',  ( 29.86685920354754487, 21.69954338932564752, -5.424999997268813878 ) ) ;
#40868=CARTESIAN_POINT ( 'NONE',  ( 6.703913744606314395, -4.665024204860747759, -64.15759393448441017 ) ) ;
#40874=ADVANCED_FACE ( 'NONE', ( #113837 ), #115860, .F. ) ;
#40899=LINE ( 'NONE', #124433, #172509 ) ;
#40900=FACE_OUTER_BOUND ( 'NONE', #52986, .T. ) ;
#40905=DIRECTION ( 'NONE',  ( 0.000000000000000000, -0.000000000000000000, -1.000000000000000000 ) ) ;
#40929=ORIENTED_EDGE ( 'NONE', *, *, #78228, .T. ) ;
#40936=ORIENTED_EDGE ( 'NONE', *, *, #99054, .F. ) ;
#40954=ADVANCED_FACE ( 'NONE', ( #66355 ), #101680, .F. ) ;
#40990=VERTEX_POINT ( 'NONE', #162356 ) ;
#40993=VERTEX_POINT ( 'NONE', #23857 ) ;
#41006=ORIENTED_EDGE ( 'NONE', *, *, #10071, .F. ) ;
#41041=ORIENTED_EDGE ( 'NONE', *, *, #80739, .T. ) ;
#41045=CARTESIAN_POINT ( 'NONE',  ( -33.56243482129945477, -21.76536163099331489, -24.28098042443967586 ) ) ;
#41057=CARTESIAN_POINT ( 'NONE',  ( 27.86273085795036408, -28.69962071417356242, -15.00000000000000178 ) ) ;
#41067=DIRECTION ( 'NONE',  ( -0.000000000000000000, -0.000000000000000000, 1.000000000000000000 ) ) ;
#41082=VERTEX_POINT ( 'NONE', #97659 ) ;
#41104=CARTESIAN_POINT ( 'NONE',  ( 31.81624771892550285, -0.5097844185666569050, -45.77220262091589831 ) ) ;
#41122=EDGE_LOOP ( 'NONE', ( #75709, #168171, #165391, #55162 ) ) ;
#41177=ORIENTED_EDGE ( 'NONE', *, *, #95674, .T. ) ;
#41195=CARTESIAN_POINT ( 'NONE',  ( -9.656827144875922642, -71.74905178543390605, -15.00000000000000178 ) ) ;
#41271=DIRECTION ( 'NONE',  ( -0.000000000000000000, -0.000000000000000000, -1.000000000000000000 ) ) ;
#41278=AXIS2_PLACEMENT_3D ( 'NONE', #4485, #69170, #66175 ) ;
#41293=CARTESIAN_POINT ( 'NONE',  ( -30.74264578624800492, -22.33583958711396278, -9.549999994537627046 ) ) ;
#41299=DIRECTION ( 'NONE',  ( -1.000000000000000000, 0.000000000000000000, 0.000000000000000000 ) ) ;
#41305=CARTESIAN_POINT ( 'NONE',  ( -12.21811429388712966, 11.10918730048719993, -59.22494048452013971 ) ) ;
#41342=CARTESIAN_POINT ( 'NONE',  ( 36.91746824999999177, 11.99521256947799230, -4.024999997268814411 ) ) ;
#41364=CARTESIAN_POINT ( 'NONE',  ( -22.88436389169415364, -32.73361847831216664, -22.76175135428083962 ) ) ;
#41375=ORIENTED_EDGE ( 'NONE', *, *, #49532, .F. ) ;
#41379=CARTESIAN_POINT ( 'NONE',  ( -1.304723572972834811, -6.853560127763683063, -64.38700459888463001 ) ) ;
#41383=EDGE_CURVE ( 'NONE', #102181, #34342, #106141, .T. ) ;
#41392=CARTESIAN_POINT ( 'NONE',  ( 0.9462312807052283281, 16.38015919949121013, -61.48063308926517578 ) ) ;
#41432=CARTESIAN_POINT ( 'NONE',  ( 0.000000000000000000, 0.000000000000000000, -64.92179855667829713 ) ) ;
#41441=( BOUNDED_SURFACE ( )  B_SPLINE_SURFACE ( 3, 2, ( 
 ( #70582, #174769, #36235 ),
 ( #115083, #8914, #159579 ),
 ( #82732, #144413, #193942 ),
 ( #5899, #83730, #190930 ),
 ( #99902, #175764, #38247 ),
 ( #52407, #37240, #98896 ),
 ( #183494, #77286, #138956 ),
 ( #169294, #435, #62110 ),
 ( #167336, #71577, #152156 ),
 ( #30800, #44978, #184483 ),
 ( #163595, #198666, #60133 ),
 ( #136977, #123773, #29807 ),
 ( #199653, #92449, #121801 ),
 ( #45962, #107616, #139942 ),
 ( #1432, #31792, #148423 ),
 ( #154137, #25096, #106638 ),
 ( #63110, #168311, #15629 ),
 ( #124788, #40237, #194935 ),
 ( #9918, #185472, #46962 ),
 ( #133243, #108621, #170299 ),
 ( #93441, #91443, #56411 ),
 ( #122793, #120807, #155128 ),
 ( #16621, #153131, #14634 ),
 ( #78269, #76293, #101913 ),
 ( #137971, #61119, #86738 ),
 ( #75306, #182506, #43986 ),
 ( #105647, #28833, #90474 ),
 ( #13639, #32785, #174284 ),
 ( #35754, #64115, #144919 ),
 ( #3422, #6401, #173290 ),
 ( #94437, #113578, #109615 ),
 ( #68082, #160098, #175272 ),
 ( #126756, #20581, #82233 ),
 ( #112592, #143923, #5404 ),
 ( #110602, #17617, #95434 ),
 ( #97399, #188459, #127755 ),
 ( #171299, #141931, #65098 ),
 ( #140946, #36738, #19599 ),
 ( #67088, #49940, #34764 ),
 ( #128747, #142922, #186487 ),
 ( #96421, #158107, #47963 ),
 ( #33774, #159086, #190444 ),
 ( #156118, #51919, #79276 ),
 ( #111605, #81241, #4404 ) ),
 .UNSPECIFIED., .F., .F., .T. ) 
 B_SPLINE_SURFACE_WITH_KNOTS ( ( 4, 2, 2, 2, 2, 2, 2, 2, 2, 2, 2, 2, 2, 2, 2, 2, 2, 2, 2, 2, 2, 4 ),
 ( 3, 3 ),
 ( 0.1334715276261017047, 0.1400397817209072804, 0.1416818452446086951, 0.1433239087683100821, 0.1466080358157128560, 0.1498921628631156300, 0.1531762899105184039, 0.1564604169579211779, 0.1597445440053239796, 0.1630286710527267813, 0.1646707345764281682, 0.1663127981001295552, 0.1679548616238309422, 0.1695969251475323292, 0.1712389886712337161, 0.1720600204330844096, 0.1728810521949351031, 0.1745231157186364901, 0.1761651792423378771, 0.1794493062897406788, 0.1827334333371434805, 0.1860175603845462544 ),
 ( 0.000000000000000000, 1.000000000000000000 ),
 .UNSPECIFIED. ) 
 GEOMETRIC_REPRESENTATION_ITEM ( )  RATIONAL_B_SPLINE_SURFACE ( (
 ( 1.000000000000000000, 0.7745966692414834043, 1.000000000000000000),
 ( 1.000000000000000000, 0.7873173169476442856, 1.000000000000000000),
 ( 1.000000000000000000, 0.8012080269091595985, 1.000000000000000000),
 ( 1.000000000000000000, 0.8197272276933328383, 1.000000000000000000),
 ( 1.000000000000000000, 0.8234885421913021863, 1.000000000000000000),
 ( 1.000000000000000000, 0.8311157573375610452, 1.000000000000000000),
 ( 1.000000000000000000, 0.8349728938257607869, 1.000000000000000000),
 ( 1.000000000000000000, 0.8465302108189354247, 1.000000000000000000),
 ( 1.000000000000000000, 0.8542644918356914197, 1.000000000000000000),
 ( 1.000000000000000000, 0.8696747091108276706, 1.000000000000000000),
 ( 1.000000000000000000, 0.8773507960691676599, 1.000000000000000000),
 ( 1.000000000000000000, 0.8925002889089016511, 1.000000000000000000),
 ( 1.000000000000000000, 0.8999891582781396338, 1.000000000000000000),
 ( 1.000000000000000000, 0.9145203485641226759, 1.000000000000000000),
 ( 1.000000000000000000, 0.9215166741119587002, 1.000000000000000000),
 ( 1.000000000000000000, 0.9348196634156782370, 1.000000000000000000),
 ( 1.000000000000000000, 0.9411264847296237912, 1.000000000000000000),
 ( 1.000000000000000000, 0.9528821887672441759, 1.000000000000000000),
 ( 1.000000000000000000, 0.9583320463343939499, 1.000000000000000000),
 ( 1.000000000000000000, 0.9657141226242618171, 1.000000000000000000),
 ( 1.000000000000000000, 0.9680424144921330187, 1.000000000000000000),
 ( 1.000000000000000000, 0.9724014971077669101, 1.000000000000000000),
 ( 1.000000000000000000, 0.9744334801158447412, 1.000000000000000000),
 ( 1.000000000000000000, 0.9781204877085358795, 1.000000000000000000),
 ( 1.000000000000000000, 0.9797809101335805959, 1.000000000000000000),
 ( 1.000000000000000000, 0.9826818083352881761, 1.000000000000000000),
 ( 1.000000000000000000, 0.9839230189806127402, 1.000000000000000000),
 ( 1.000000000000000000, 0.9859013487406023124, 1.000000000000000000),
 ( 1.000000000000000000, 0.9866146582094301731, 1.000000000000000000),
 ( 1.000000000000000000, 0.9872250220265939014, 1.000000000000000000),
 ( 1.000000000000000000, 0.9873522598263766437, 1.000000000000000000),
 ( 1.000000000000000000, 0.9874472609175324322, 1.000000000000000000),
 ( 1.000000000000000000, 0.9874138636738953867, 1.000000000000000000),
 ( 1.000000000000000000, 0.9870735186573816877, 1.000000000000000000),
 ( 1.000000000000000000, 0.9865315217161264583, 1.000000000000000000),
 ( 1.000000000000000000, 0.9848873008857174094, 1.000000000000000000),
 ( 1.000000000000000000, 0.9837743821442677117, 1.000000000000000000),
 ( 1.000000000000000000, 0.9797976954002749483, 1.000000000000000000),
 ( 1.000000000000000000, 0.9763000371664851684, 1.000000000000000000),
 ( 1.000000000000000000, 0.9680363503266700143, 1.000000000000000000),
 ( 1.000000000000000000, 0.9632464763793491258, 1.000000000000000000),
 ( 1.000000000000000000, 0.9526889542241591124, 1.000000000000000000),
 ( 1.000000000000000000, 0.9469283804590789000, 1.000000000000000000),
 ( 1.000000000000000000, 0.9407878411039238831, 1.000000000000000000) ) ) 
 REPRESENTATION_ITEM ( '' )  SURFACE ( )  );
#41494=B_SPLINE_CURVE_WITH_KNOTS ( 'NONE', 3,
 ( #76982, #107313, #182196, #183191, #92141, #32483, #154823, #155815, #43681, #15323, #167030, #75006, #121497, #28532, #152831, #45662, #168986, #106326, #90168, #123473, #136671, #198353, #168012, #29508, #30490, #153828 ),
 .UNSPECIFIED., .F., .F.,
 ( 4, 2, 2, 2, 2, 2, 2, 2, 2, 2, 2, 2, 4 ),
 ( 1.971416326362521810E-07, 0.0002960211146593206026, 0.0005918450876860049644, 0.0008876690607126895430, 0.001183493033739374230, 0.001775140979792742737, 0.002366788925846110593, 0.002662612898872792570, 0.002958436871899474113, 0.003254260844926156089, 0.003550084817952837632, 0.004141732764006201585, 0.004733380710059564671 ),
 .UNSPECIFIED. ) ;
#41521=VERTEX_POINT ( 'NONE', #164379 ) ;
#41549=CARTESIAN_POINT ( 'NONE',  ( 20.12987255291491095, 20.83652723102580495, -52.58065409862962269 ) ) ;
#41554=CARTESIAN_POINT ( 'NONE',  ( 11.74264578624799427, 36.14014761921585972, -4.599999999999999645 ) ) ;
#41570=CARTESIAN_POINT ( 'NONE',  ( 25.80819889657193045, -27.69677943096044714, -16.54815200935614428 ) ) ;
#41588=ORIENTED_EDGE ( 'NONE', *, *, #194310, .T. ) ;
#41679=VECTOR ( 'NONE', #181068, 1000.000000000000000 ) ;
#41686=CARTESIAN_POINT ( 'NONE',  ( 20.43538597629128262, -20.43538597629122222, -64.92279855667830191 ) ) ;
#41756=CARTESIAN_POINT ( 'NONE',  ( 22.80000000000002913, -8.654466842953076985E-14, -64.92279855667830191 ) ) ;
#41777=CARTESIAN_POINT ( 'NONE',  ( 0.000000000000000000, -105.0000000000000000, 12.00000000000000355 ) ) ;
#41790=DIRECTION ( 'NONE',  ( 1.000000000000000000, 0.000000000000000000, 0.000000000000000000 ) ) ;
#41808=ORIENTED_EDGE ( 'NONE', *, *, #145235, .F. ) ;
#41811=CARTESIAN_POINT ( 'NONE',  ( -30.74264578624800492, 22.33583958711400186, -0.1999999999999999001 ) ) ;
#41839=CARTESIAN_POINT ( 'NONE',  ( 6.310639553377889399, -38.36010752038117033, -23.94295717418827252 ) ) ;
#41842=ORIENTED_EDGE ( 'NONE', *, *, #19937, .F. ) ;
#41844=VERTEX_POINT ( 'NONE', #29830 ) ;
#41859=VECTOR ( 'NONE', #2927, 1000.000000000000000 ) ;
#41874=CARTESIAN_POINT ( 'NONE',  ( -11.40812507854754720, -35.11059874428192273, -4.224999997268813701 ) ) ;
#41891=EDGE_CURVE ( 'NONE', #144280, #57253, #64929, .T. ) ;
#41911=DIRECTION ( 'NONE',  ( -1.000000000000000000, 0.000000000000000000, 0.000000000000000000 ) ) ;
#41979=AXIS2_PLACEMENT_3D ( 'NONE', #144582, #21249, #80918 ) ;
#42040=DIRECTION ( 'NONE',  ( -1.000000000000000000, 0.000000000000000000, 0.000000000000000000 ) ) ;
#42050=CARTESIAN_POINT ( 'NONE',  ( -32.61617023573567309, -23.16041576125357082, -21.42686488341023932 ) ) ;
#42057=VERTEX_POINT ( 'NONE', #172307 ) ;
#42060=DIRECTION ( 'NONE',  ( -0.9526137857479314297, -0.3041824702427711746, 0.000000000000000000 ) ) ;
#42068=CARTESIAN_POINT ( 'NONE',  ( 11.26676076908655766, -37.89014424912599566, -31.17854569212329707 ) ) ;
#42100=EDGE_CURVE ( 'NONE', #70273, #130796, #105442, .T. ) ;
#42107=ORIENTED_EDGE ( 'NONE', *, *, #116672, .T. ) ;
#42121=DIRECTION ( 'NONE',  ( -0.000000000000000000, -0.000000000000000000, 1.000000000000000000 ) ) ;
#42134=ORIENTED_EDGE ( 'NONE', *, *, #152270, .F. ) ;
#42200=AXIS2_PLACEMENT_3D ( 'NONE', #80283, #141955, #62132 ) ;
#42256=B_SPLINE_CURVE_WITH_KNOTS ( 'NONE', 3,
 ( #28405, #91014, #14189, #150741, #57736, #90044, #102232, #103233, #164915, #137535, #13219, #42564, #181089, #199216, #119406, #58706 ),
 .UNSPECIFIED., .F., .F.,
 ( 4, 2, 2, 2, 2, 2, 2, 4 ),
 ( 0.001176332860010937233, 0.001620974858810565918, 0.002065616857610193952, 0.002954900855209450887, 0.003399542854009075452, 0.003844184852808700016, 0.004288826851608324581, 0.004733468850407949145 ),
 .UNSPECIFIED. ) ;
#42259=ADVANCED_FACE ( 'NONE', ( #92472 ), #15652, .F. ) ;
#42289=ORIENTED_EDGE ( 'NONE', *, *, #143629, .T. ) ;
#42295=CARTESIAN_POINT ( 'NONE',  ( 23.48529157249599919, 32.32473071737754111, -10.44999999453762385 ) ) ;
#42301=CARTESIAN_POINT ( 'NONE',  ( 4.803421339707764304, -3.978740937077453577, -62.48491958522772904 ) ) ;
#42324=LINE ( 'NONE', #58473, #165976 ) ;
#42344=CARTESIAN_POINT ( 'NONE',  ( -36.91746825000000598, 11.99521256947798520, -7.224999997268813701 ) ) ;
#42345=CYLINDRICAL_SURFACE ( 'NONE', #157214, 12.50000000000000000 ) ;
#42353=CARTESIAN_POINT ( 'NONE',  ( 28.98398574327581301, -24.58691951735649894, -17.12116358423670448 ) ) ;
#42359=VERTEX_POINT ( 'NONE', #156141 ) ;
#42365=CARTESIAN_POINT ( 'NONE',  ( -22.23580286100235526, -34.17069428431420874, -18.13567467416600820 ) ) ;
#42366=VERTEX_POINT ( 'NONE', #3444 ) ;
#42392=CARTESIAN_POINT ( 'NONE',  ( 6.292920404648722155, -0.7621229312825326119, -64.49503546857651770 ) ) ;
#42477=CARTESIAN_POINT ( 'NONE',  ( 0.000000000000000000, 0.000000000000000000, -54.21489346206828230 ) ) ;
#42498=CARTESIAN_POINT ( 'NONE',  ( -19.38985940809734032, -32.68077955211932561, -25.00000000000009592 ) ) ;
#42510=VERTEX_POINT ( 'NONE', #70117 ) ;
#42515=EDGE_CURVE ( 'NONE', #21583, #125361, #9454, .T. ) ;
#42534=VERTEX_POINT ( 'NONE', #55943 ) ;
#42536=CARTESIAN_POINT ( 'NONE',  ( 193.3062444957835453, -155.7167183371837496, -15.00000000000000178 ) ) ;
#42543=CARTESIAN_POINT ( 'NONE',  ( 21.84063423829474715, 22.96000461283902894, -49.40985016368630767 ) ) ;
#42545=CARTESIAN_POINT ( 'NONE',  ( -36.91746825000000598, 2.428612866367529932E-14, -11.12499999726881228 ) ) ;
#42548=CARTESIAN_POINT ( 'NONE',  ( -5.000000000000000000, 6.123233995736766282E-16, -15.00000000000000000 ) ) ;
#42564=CARTESIAN_POINT ( 'NONE',  ( -5.802100494052803370, -6.819150417750785564, -63.98534035886881099 ) ) ;
#42587=CARTESIAN_POINT ( 'NONE',  ( -6.434671708797603529, 6.434671708797564449, -63.95112321872120731 ) ) ;
#42618=FACE_OUTER_BOUND ( 'NONE', #125018, .T. ) ;
#42631=( BOUNDED_CURVE ( )  B_SPLINE_CURVE ( 2, ( #114314, #99147, #9163, #194187, #70830, #179020, #40488, #102160, #27336, #134509, #90943 ),
 .UNSPECIFIED., .F., .F. ) 
 B_SPLINE_CURVE_WITH_KNOTS ( ( 3, 2, 2, 2, 2, 3 ),
 ( 0.6000000000000000888, 0.6200000000000001066, 0.6400000000000001243, 0.6600000000000001421, 0.6800000000000001599, 0.7000000000000000666 ),
 .UNSPECIFIED. ) 
 CURVE ( )  GEOMETRIC_REPRESENTATION_ITEM ( )  RATIONAL_B_SPLINE_CURVE ( ( 0.9999999999999997780, 0.9510565162951537532, 1.000000000000000000, 0.9510565162951535312, 1.000000000000000000, 0.9510565162951535312, 1.000000000000000000, 0.9510565162951535312, 1.000000000000000000, 0.9510565162951533091, 1.000000000000000222 ) ) 
 REPRESENTATION_ITEM ( '' )  );
#42654=DIRECTION ( 'NONE',  ( -0.000000000000000000, -0.000000000000000000, 1.000000000000000000 ) ) ;
#42667=ADVANCED_FACE ( 'NONE', ( #12459 ), #25635, .F. ) ;
#42762=EDGE_CURVE ( 'NONE', #176889, #197513, #34935, .T. ) ;
#42785=CARTESIAN_POINT ( 'NONE',  ( -28.90000000000004476, 2.980639576201346218E-13, -49.67367017693150189 ) ) ;
#42790=EDGE_CURVE ( 'NONE', #84237, #42534, #2607, .T. ) ;
#42791=CARTESIAN_POINT ( 'NONE',  ( -1.250870343808723417, -21.94965239947791247, -55.99511580764671237 ) ) ;
#42809=CARTESIAN_POINT ( 'NONE',  ( 11.74264578624799427, 36.14014761921585972, -8.599999999999999645 ) ) ;
#42814=DIRECTION ( 'NONE',  ( 0.000000000000000000, 0.000000000000000000, 1.000000000000000000 ) ) ;
#42839=EDGE_LOOP ( 'NONE', ( #192307, #164191 ) ) ;
#42910=DIRECTION ( 'NONE',  ( 0.000000000000000000, 0.000000000000000000, 1.000000000000000000 ) ) ;
#42985=ORIENTED_EDGE ( 'NONE', *, *, #34928, .T. ) ;
#42989=EDGE_LOOP ( 'NONE', ( #109000, #132938, #121788, #48322, #24378 ) ) ;
#43025=EDGE_CURVE ( 'NONE', #43345, #156405, #9121, .T. ) ;
#43037=CARTESIAN_POINT ( 'NONE',  ( -29.86685920354755197, -21.69954338932560134, -8.424999997268812990 ) ) ;
#43054=CARTESIAN_POINT ( 'NONE',  ( 12.04662589228224689, -37.70593178236023846, -30.82293284779730769 ) ) ;
#43092=AXIS2_PLACEMENT_3D ( 'NONE', #165008, #88144, #38659 ) ;
#43192=( BOUNDED_CURVE ( )  B_SPLINE_CURVE ( 2, ( #68363, #192725, #130014, #54209, #7683, #100694, #193734, #159369, #191713, #86536, #53197, #101700, #67367, #8707, #131036, #20866, #56202, #113858, #69367, #177570, #9714, #82523, #162375, #133042, #40027, #97680, #38042, #23877, #71378, #178562, #70377, #144205, #174564, #85528, #132045, #148220, #147216, #36031, #114872, #55202, #52200, #116871, #160384, #99698, #175554, #83524, #37029, #98690, #21874, #137015, #168352, #12707, #25891, #153172, #76336, #11722, #58205, #106679, #10714, #57217, #182546, #44028, #121841, #87536, #138012, #90513, #150226, #119874, #167376, #28872, #60172, #135062, #149223, #164399, #120847, #183535, #197713, #196738, #43037, #73390, #105689, #59178, #181559, #104703, #29848, #91485, #72377, #199696, #74373, #75346, #166392, #152195, #118891, #180576, #13679, #198705, #134051, #136038, #14674, #45019, #117884 ),
 .UNSPECIFIED., .F., .T. ) 
 B_SPLINE_CURVE_WITH_KNOTS ( ( 3, 2, 2, 2, 2, 2, 2, 2, 2, 2, 2, 2, 2, 2, 2, 2, 2, 2, 2, 2, 2, 2, 2, 2, 2, 2, 2, 2, 2, 2, 2, 2, 2, 2, 2, 2, 2, 2, 2, 2, 2, 2, 2, 2, 2, 2, 2, 2, 2, 2, 3 ),
 ( 0.000000000000000000, 0.02000000000000000042, 0.04000000000000000083, 0.05999999999999999778, 0.08000000000000000167, 0.1000000000000000056, 0.1199999999999999956, 0.1400000000000000133, 0.1600000000000000033, 0.1799999999999999933, 0.2000000000000000111, 0.2200000000000000011, 0.2399999999999999911, 0.2600000000000000089, 0.2800000000000000266, 0.2999999999999999889, 0.3200000000000000067, 0.3400000000000000244, 0.3599999999999999867, 0.3800000000000000044, 0.4000000000000000222, 0.4199999999999999845, 0.4400000000000000022, 0.4600000000000000200, 0.4799999999999999822, 0.5000000000000000000, 0.5200000000000000178, 0.5400000000000000355, 0.5600000000000000533, 0.5799999999999999600, 0.5999999999999999778, 0.6199999999999999956, 0.6400000000000000133, 0.6600000000000000311, 0.6800000000000000488, 0.6999999999999999556, 0.7199999999999999734, 0.7399999999999999911, 0.7600000000000000089, 0.7800000000000000266, 0.8000000000000000444, 0.8199999999999999512, 0.8399999999999999689, 0.8599999999999999867, 0.8800000000000000044, 0.9000000000000000222, 0.9200000000000000400, 0.9399999999999999467, 0.9599999999999999645, 0.9799999999999999822, 1.000000000000000000 ),
 .UNSPECIFIED. ) 
 CURVE ( )  GEOMETRIC_REPRESENTATION_ITEM ( )  RATIONAL_B_SPLINE_CURVE ( ( 1.000000000000000000, 0.9510565162951535312, 1.000000000000000000, 0.9510565162951535312, 1.000000000000000000, 0.9510565162951535312, 1.000000000000000000, 0.9510565162951535312, 1.000000000000000000, 0.9510565162951535312, 1.000000000000000000, 0.9510565162951535312, 1.000000000000000000, 0.9510565162951535312, 1.000000000000000000, 0.9510565162951535312, 1.000000000000000000, 0.9510565162951535312, 1.000000000000000000, 0.9510565162951535312, 1.000000000000000000, 0.9510565162951535312, 1.000000000000000000, 0.9510565162951535312, 1.000000000000000000, 0.9510565162951535312, 1.000000000000000000, 0.9510565162951535312, 1.000000000000000000, 0.9510565162951535312, 1.000000000000000000, 0.9510565162951535312, 1.000000000000000000, 0.9510565162951535312, 1.000000000000000000, 0.9510565162951535312, 1.000000000000000000, 0.9510565162951535312, 1.000000000000000000, 0.9510565162951535312, 1.000000000000000000, 0.9510565162951535312, 1.000000000000000000, 0.9510565162951535312, 1.000000000000000000, 0.9510565162951535312, 1.000000000000000000, 0.9510565162951535312, 1.000000000000000000, 0.9510565162951535312, 1.000000000000000000, 0.9510565162951535312, 1.000000000000000000, 0.9510565162951535312, 1.000000000000000000, 0.9510565162951535312, 1.000000000000000000, 0.9510565162951535312, 1.000000000000000000, 0.9510565162951535312, 1.000000000000000000, 0.9510565162951535312, 1.000000000000000000, 0.9510565162951535312, 1.000000000000000000, 0.9510565162951535312, 1.000000000000000000, 0.9510565162951535312, 1.000000000000000000, 0.9510565162951535312, 1.000000000000000000, 0.9510565162951535312, 1.000000000000000000, 0.9510565162951535312, 1.000000000000000000, 0.9510565162951535312, 1.000000000000000000, 0.9510565162951535312, 1.000000000000000000, 0.9510565162951535312, 1.000000000000000000, 0.9510565162951535312, 1.000000000000000000, 0.9510565162951535312, 1.000000000000000000, 0.9510565162951535312, 1.000000000000000000, 0.9510565162951535312, 1.000000000000000000, 0.9510565162951535312, 1.000000000000000000, 0.9510565162951535312, 1.000000000000000000, 0.9510565162951535312, 1.000000000000000000, 0.9510565162951535312, 1.000000000000000000, 0.9510565162951535312, 1.000000000000000000, 0.9510565162951535312, 1.000000000000000000 ) ) 
 REPRESENTATION_ITEM ( '' )  );
#43230=AXIS2_PLACEMENT_3D ( 'NONE', #99950, #102960, #41299 ) ;
#43244=DIRECTION ( 'NONE',  ( -0.000000000000000000, 0.000000000000000000, 1.000000000000000000 ) ) ;
#43256=DIRECTION ( 'NONE',  ( 0.000000000000000000, 0.000000000000000000, 1.000000000000000000 ) ) ;
#43264=CARTESIAN_POINT ( 'NONE',  ( 10.19492084563873391, -9.320932348315787763, -60.40172357148235704 ) ) ;
#43271=ORIENTED_EDGE ( 'NONE', *, *, #170016, .F. ) ;
#43279=CARTESIAN_POINT ( 'NONE',  ( 38.00000000000000000, 12.34694845685046616, -10.64999999453762491 ) ) ;
#43292=VECTOR ( 'NONE', #23423, 1000.000000000000000 ) ;
#43304=CARTESIAN_POINT ( 'NONE',  ( -21.65131445265848598, 0.9841389949903269763, -58.61993113718295945 ) ) ;
#43313=CIRCLE ( 'NONE', #175652, 40.00000000000000711 ) ;
#43330=CARTESIAN_POINT ( 'NONE',  ( 29.86685920354754487, 21.69954338932564752, -5.924999997268813878 ) ) ;
#43331=CARTESIAN_POINT ( 'NONE',  ( -38.00000000000000711, 2.428612866367529932E-14, -8.000000000000000000 ) ) ;
#43345=VERTEX_POINT ( 'NONE', #92233 ) ;
#43351=CARTESIAN_POINT ( 'NONE',  ( -27.83073679762865638, -28.30972371523964881, -20.09501658340063557 ) ) ;
#43365=CARTESIAN_POINT ( 'NONE',  ( -0.6701480022146820703, -8.945614359730862830, -63.98123544873404711 ) ) ;
#43386=DIRECTION ( 'NONE',  ( -1.000000000000000000, 0.000000000000000000, 0.000000000000000000 ) ) ;
#43397=AXIS2_PLACEMENT_3D ( 'NONE', #176257, #175249, #146908 ) ;
#43402=ORIENTED_EDGE ( 'NONE', *, *, #6742, .F. ) ;
#43421=CIRCLE ( 'NONE', #75728, 21.30000000000002913 ) ;
#43460=EDGE_CURVE ( 'NONE', #85102, #116714, #74632, .T. ) ;
#43483=CARTESIAN_POINT ( 'NONE',  ( -6.837351365824967608, 5.758699013978442416, -61.93409818843132797 ) ) ;
#43487=CARTESIAN_POINT ( 'NONE',  ( -25.96435248595175693, -27.35529834266888116, -20.33897993952049887 ) ) ;
#43500=ORIENTED_EDGE ( 'NONE', *, *, #128552, .T. ) ;
#43506=CYLINDRICAL_SURFACE ( 'NONE', #18184, 1.500000000000001332 ) ;
#43532=CARTESIAN_POINT ( 'NONE',  ( 19.98428748653497422, 21.47640361312187096, -52.19293734151717956 ) ) ;
#43534=CARTESIAN_POINT ( 'NONE',  ( 4.999999999999999112, 11.45643923738960090, -15.00000000000000000 ) ) ;
#43552=CARTESIAN_POINT ( 'NONE',  ( 23.23284429171615884, -30.31406682163549959, -16.83429831496583873 ) ) ;
#43559=ADVANCED_FACE ( 'NONE', ( #188251 ), #145708, .F. ) ;
#43573=CIRCLE ( 'NONE', #140535, 21.30000000000002913 ) ;
#43577=CARTESIAN_POINT ( 'NONE',  ( -4.713425861958496554, 4.023676584314499038, -64.51712888360829368 ) ) ;
#43607=CARTESIAN_POINT ( 'NONE',  ( 0.000000000000000000, 0.000000000000000000, -25.00000000000000000 ) ) ;
#43611=ORIENTED_EDGE ( 'NONE', *, *, #162842, .F. ) ;
#43620=DIRECTION ( 'NONE',  ( -1.000000000000000000, 0.000000000000000000, 0.000000000000000000 ) ) ;
#43633=AXIS2_PLACEMENT_3D ( 'NONE', #136722, #134763, #103416 ) ;
#43645=CARTESIAN_POINT ( 'NONE',  ( 30.20036327792367814, -26.22857331006468584, -17.18026671435356434 ) ) ;
#43681=CARTESIAN_POINT ( 'NONE',  ( -8.725106586199771641, 0.9968436689773673143, -64.02420483255114902 ) ) ;
#43732=ORIENTED_EDGE ( 'NONE', *, *, #155029, .T. ) ;
#43738=ORIENTED_EDGE ( 'NONE', *, *, #124684, .F. ) ;
#43740=CARTESIAN_POINT ( 'NONE',  ( -38.00000000000000711, 2.428612866367529932E-14, -7.749999994537626336 ) ) ;
#43783=AXIS2_PLACEMENT_3D ( 'NONE', #17316, #139641, #3134 ) ;
#43795=CARTESIAN_POINT ( 'NONE',  ( 11.74264578624799427, 36.14014761921585972, -6.599999999999999645 ) ) ;
#43800=DIRECTION ( 'NONE',  ( 0.000000000000000000, 0.000000000000000000, 1.000000000000000000 ) ) ;
#43805=CARTESIAN_POINT ( 'NONE',  ( -193.3062444957834884, -155.7167183371838064, -23.00000000000000000 ) ) ;
#43880=VECTOR ( 'NONE', #159620, 1000.000000000000000 ) ;
#43907=B_SPLINE_CURVE_WITH_KNOTS ( 'NONE', 3,
 ( #185389, #157037, #18534, #3344, #65019, #139464, #94956, #122308, #2947, #137487 ),
 .UNSPECIFIED., .F., .F.,
 ( 4, 2, 2, 2, 4 ),
 ( 2.788259402197439630E-07, 0.0002944003759562778284, 0.0005885219259723359700, 0.0008826434759883940032, 0.001176765026004452036 ),
 .UNSPECIFIED. ) ;
#43928=CARTESIAN_POINT ( 'NONE',  ( -193.3062444957834884, -155.7167183371838064, 0.000000000000000000 ) ) ;
#43973=ORIENTED_EDGE ( 'NONE', *, *, #133150, .T. ) ;
#43976=ORIENTED_EDGE ( 'NONE', *, *, #7317, .F. ) ;
#43981=AXIS2_PLACEMENT_3D ( 'NONE', #51071, #101554, #86396 ) ;
#43986=CARTESIAN_POINT ( 'NONE',  ( -23.14280555631616210, -30.41650385747668750, -16.87365452859015136 ) ) ;
#43991=ORIENTED_EDGE ( 'NONE', *, *, #194548, .F. ) ;
#44000=B_SPLINE_CURVE_WITH_KNOTS ( 'NONE', 3,
 ( #94585, #106780, #4544, #172432, #114734, #7545 ),
 .UNSPECIFIED., .F., .F.,
 ( 4, 2, 4 ),
 ( 0.003693721832073882522, 0.004289092630022420076, 0.004884463427970957630 ),
 .UNSPECIFIED. ) ;
#44004=CARTESIAN_POINT ( 'NONE',  ( -18.36170132746697803, -35.61590944478785303, -18.35554273634631528 ) ) ;
#44014=CARTESIAN_POINT ( 'NONE',  ( -14.76558643118678305, -15.47416251488300887, -56.40920624782621928 ) ) ;
#44025=VERTEX_POINT ( 'NONE', #42548 ) ;
#44028=CARTESIAN_POINT ( 'NONE',  ( -36.91746825000000598, 11.99521256947798520, -6.724999997268813701 ) ) ;
#44038=EDGE_CURVE ( 'NONE', #117777, #172040, #166286, .T. ) ;
#44048=CARTESIAN_POINT ( 'NONE',  ( 8.817897698974592302, -38.37206457205375187, -32.07286502659245286 ) ) ;
#44105=CARTESIAN_POINT ( 'NONE',  ( 4.999999999999996447, 5.000000000000003553, -18.00000000000000000 ) ) ;
#44126=EDGE_CURVE ( 'NONE', #179372, #105638, #9152, .T. ) ;
#44268=EDGE_LOOP ( 'NONE', ( #199754, #69163, #135578, #66704 ) ) ;
#44272=LINE ( 'NONE', #57459, #27004 ) ;
#44276=CARTESIAN_POINT ( 'NONE',  ( 22.81625015709509441, 31.40387420917330275, -5.824999997268813345 ) ) ;
#44300=CARTESIAN_POINT ( 'NONE',  ( -24.06642195515787108, 0.8101246706336291403, -56.93999021579660536 ) ) ;
#44312=CARTESIAN_POINT ( 'NONE',  ( -11.80868324581538253, 11.80868324581533457, -65.00100000000003320 ) ) ;
#44315=DIRECTION ( 'NONE',  ( 0.000000000000000000, 0.000000000000000000, -1.000000000000000000 ) ) ;
#44326=CARTESIAN_POINT ( 'NONE',  ( -36.91746825000000598, 11.99521256947798520, -9.224999997268813701 ) ) ;
#44328=CARTESIAN_POINT ( 'NONE',  ( -11.80868324581538253, 11.80868324581533457, -61.34707691135562868 ) ) ;
#44330=CARTESIAN_POINT ( 'NONE',  ( 0.6703450422171775003, 8.945518415904238907, -63.98125415533367999 ) ) ;
#44341=ORIENTED_EDGE ( 'NONE', *, *, #136647, .F. ) ;
#44347=CARTESIAN_POINT ( 'NONE',  ( -21.89035704509619862, -33.26311937564968702, -20.38189100991792557 ) ) ;
#44348=VERTEX_POINT ( 'NONE', #144357 ) ;
#44363=CARTESIAN_POINT ( 'NONE',  ( 37.99999999999999289, 2.893978650043524126E-14, -10.74999999453762811 ) ) ;
#44375=CARTESIAN_POINT ( 'NONE',  ( 6.139823915386828368, -0.3964520562363907374, -64.52448473163055098 ) ) ;
#44393=EDGE_CURVE ( 'NONE', #3755, #42366, #188903, .T. ) ;
#44414=DIRECTION ( 'NONE',  ( 1.000000000000000000, 0.000000000000000000, 0.000000000000000000 ) ) ;
#44482=VECTOR ( 'NONE', #14171, 1000.000000000000000 ) ;
#44492=ORIENTED_EDGE ( 'NONE', *, *, #103099, .T. ) ;
#44498=PLANE ( 'NONE',  #127987 ) ;
#44545=CARTESIAN_POINT ( 'NONE',  ( 27.39934578958845179, -26.16170490841984630, -16.57183124570353172 ) ) ;
#44600=DIRECTION ( 'NONE',  ( 0.000000000000000000, 1.000000000000000000, 0.000000000000000000 ) ) ;
#44637=ORIENTED_EDGE ( 'NONE', *, *, #188177, .F. ) ;
#44667=DIRECTION ( 'NONE',  ( -9.445700745138859830E-17, 1.000000000000000000, 0.000000000000000000 ) ) ;
#44722=ORIENTED_EDGE ( 'NONE', *, *, #62577, .T. ) ;
#44728=ORIENTED_EDGE ( 'NONE', *, *, #17351, .T. ) ;
#44753=CARTESIAN_POINT ( 'NONE',  ( -38.00000000000000711, 12.34694845685046438, -5.849999994537627757 ) ) ;
#44766=CARTESIAN_POINT ( 'NONE',  ( 14.46985881644522465, -1.324169127979137883, -60.11284999819414310 ) ) ;
#44770=CARTESIAN_POINT ( 'NONE',  ( -20.41037832431298682, -34.40082058117823749, -25.00000000000009592 ) ) ;
#44782=ORIENTED_EDGE ( 'NONE', *, *, #193684, .F. ) ;
#44785=CARTESIAN_POINT ( 'NONE',  ( -6.020228577223754586E-15, 39.95556452105416412, -2.500000000000000444 ) ) ;
#44810=CARTESIAN_POINT ( 'NONE',  ( 11.22590306719470377, -43.10241010958339558, -21.31070173013108260 ) ) ;
#44832=EDGE_CURVE ( 'NONE', #71451, #99831, #188659, .T. ) ;
#44838=VERTEX_POINT ( 'NONE', #162525 ) ;
#44912=ORIENTED_EDGE ( 'NONE', *, *, #13873, .T. ) ;
#44928=CARTESIAN_POINT ( 'NONE',  ( 16.23105266556536463, 17.63037570847457047, -54.49189616393496749 ) ) ;
#44978=CARTESIAN_POINT ( 'NONE',  ( -10.08838716500075883, -37.25234734385823998, -23.84483522324640958 ) ) ;
#45009=CARTESIAN_POINT ( 'NONE',  ( 20.50626127892844863, -20.36451067365405976, -52.65483682830183909 ) ) ;
#45019=CARTESIAN_POINT ( 'NONE',  ( -36.91746825000000598, -11.99521256947794789, -10.52499999726881441 ) ) ;
#45021=AXIS2_PLACEMENT_3D ( 'NONE', #173787, #140441, #34268 ) ;
#45031=DIRECTION ( 'NONE',  ( -0.000000000000000000, -0.000000000000000000, 1.000000000000000000 ) ) ;
#45041=CARTESIAN_POINT ( 'NONE',  ( -9.248023074035630842, -11.04433579861080084, -62.31744588651325500 ) ) ;
#45095=CARTESIAN_POINT ( 'NONE',  ( 11.74264578624799427, 36.14014761921585972, -2.600000000000000533 ) ) ;
#45122=DIRECTION ( 'NONE',  ( 0.000000000000000000, -0.000000000000000000, -1.000000000000000000 ) ) ;
#45144=EDGE_CURVE ( 'NONE', #115376, #99310, #4595, .T. ) ;
#45156=ORIENTED_EDGE ( 'NONE', *, *, #6979, .F. ) ;
#45170=VECTOR ( 'NONE', #175951, 1000.000000000000000 ) ;
#45175=EDGE_CURVE ( 'NONE', #120193, #182074, #126097, .T. ) ;
#45232=CARTESIAN_POINT ( 'NONE',  ( 1.500000000000000888, 15.20000000000002061, -59.79525829764741474 ) ) ;
#45248=FACE_BOUND ( 'NONE', #109084, .T. ) ;
#45254=CARTESIAN_POINT ( 'NONE',  ( 0.2208081763724077662, 21.31244378140432971, -58.84882290019458395 ) ) ;
#45261=VERTEX_POINT ( 'NONE', #56353 ) ;
#45269=CARTESIAN_POINT ( 'NONE',  ( 3.556970738554033499E-15, -38.81732327939057825, -2.624999997268812724 ) ) ;
#45282=CARTESIAN_POINT ( 'NONE',  ( 4.070616889113809478, 4.625078002628068674, -62.49731305256334224 ) ) ;
#45288=ADVANCED_FACE ( 'NONE', ( #153083 ), #198618, .T. ) ;
#45328=CARTESIAN_POINT ( 'NONE',  ( 30.98370104197785224, -22.00508125442255647, -21.15278651796061382 ) ) ;
#45340=CARTESIAN_POINT ( 'NONE',  ( -37.91032098691104579, -19.19859865632797025, -20.09511994390769729 ) ) ;
#45362=LINE ( 'NONE', #27225, #140419 ) ;
#45388=VERTEX_POINT ( 'NONE', #60085 ) ;
#45461=CARTESIAN_POINT ( 'NONE',  ( -6.576301504920873953, 6.293041912674299354, -61.89430850415822505 ) ) ;
#45465=CARTESIAN_POINT ( 'NONE',  ( -20.53125566280828806, 20.33951628977422743, -49.67367017693150189 ) ) ;
#45482=DIRECTION ( 'NONE',  ( -0.000000000000000000, -0.000000000000000000, 1.000000000000000000 ) ) ;
#45483=FACE_BOUND ( 'NONE', #200173, .T. ) ;
#45512=CARTESIAN_POINT ( 'NONE',  ( 22.10131684062755042, -1.340157125434722429, -58.31342218742626216 ) ) ;
#45550=LINE ( 'NONE', #89070, #173238 ) ;
#45586=CARTESIAN_POINT ( 'NONE',  ( 15.06137443927351072, -15.06137443927345210, -56.46919128290398504 ) ) ;
#45626=DIRECTION ( 'NONE',  ( -0.000000000000000000, 0.000000000000000000, 1.000000000000000000 ) ) ;
#45662=CARTESIAN_POINT ( 'NONE',  ( -7.214655873249279594, 1.452908486251215381, -64.31726809345073548 ) ) ;
#45711=CARTESIAN_POINT ( 'NONE',  ( 20.43538597629129328, 20.43538597629121156, -52.65483682830182488 ) ) ;
#45716=VERTEX_POINT ( 'NONE', #170250 ) ;
#45718=CARTESIAN_POINT ( 'NONE',  ( -6.020228577223754586E-15, 39.95556452105416412, -8.249999994537626336 ) ) ;
#45728=CARTESIAN_POINT ( 'NONE',  ( 16.38029848613153661, -0.9460486868805465521, -61.48057501744755626 ) ) ;
#45750=CARTESIAN_POINT ( 'NONE',  ( 3.503282210674363295, -48.86437366581479580, -25.00000000000000000 ) ) ;
#45754=CARTESIAN_POINT ( 'NONE',  ( -0.1123844339349781840, -21.30000000000003268, -56.46919128290401346 ) ) ;
#45759=DIRECTION ( 'NONE',  ( -0.000000000000000000, -0.000000000000000000, 1.000000000000000000 ) ) ;
#45764=CARTESIAN_POINT ( 'NONE',  ( -15.69994562750274447, 14.67883866103742463, -58.73507448357034377 ) ) ;
#45773=CARTESIAN_POINT ( 'NONE',  ( 23.48529157249599919, 32.32473071737754111, -6.700000000000001066 ) ) ;
#45774=CIRCLE ( 'NONE', #68420, 59.99999999999998579 ) ;
#45799=CARTESIAN_POINT ( 'NONE',  ( 19.25015247713429289, -32.77362114220795064, -25.12817986193741859 ) ) ;
#45827=VERTEX_POINT ( 'NONE', #122743 ) ;
#45830=CARTESIAN_POINT ( 'NONE',  ( 1.464443979261886630, 14.82300492994660068, -62.12379213640164721 ) ) ;
#45831=VERTEX_POINT ( 'NONE', #107567 ) ;
#45883=DIRECTION ( 'NONE',  ( 1.000000000000000000, 0.000000000000000000, 0.000000000000000000 ) ) ;
#45905=DIRECTION ( 'NONE',  ( 1.000000000000000000, 0.000000000000000000, 0.000000000000000000 ) ) ;
#45912=CARTESIAN_POINT ( 'NONE',  ( 14.61887724323083937, 16.11132338694242350, -56.15647863711520671 ) ) ;
#45914=CARTESIAN_POINT ( 'NONE',  ( -11.74264578624799782, -36.14014761921581709, -11.34999999453762776 ) ) ;
#45962=CARTESIAN_POINT ( 'NONE',  ( -16.87022414723119113, -33.99382086345450915, -27.12615631800879967 ) ) ;
#45985=CARTESIAN_POINT ( 'NONE',  ( 23.48529157249600630, -32.32473071737748427, -9.300000000000000711 ) ) ;
#46012=DIRECTION ( 'NONE',  ( -0.000000000000000000, -0.000000000000000000, 1.000000000000000000 ) ) ;
#46020=CARTESIAN_POINT ( 'NONE',  ( 8.543935154430876366, -46.31530851241901559, -24.25021605108609535 ) ) ;
#46060=EDGE_CURVE ( 'NONE', #145210, #138331, #77238, .T. ) ;
#46142=DIRECTION ( 'NONE',  ( -0.000000000000000000, -0.000000000000000000, 1.000000000000000000 ) ) ;
#46152=ADVANCED_FACE ( 'NONE', ( #118034 ), #70525, .F. ) ;
#46233=FACE_BOUND ( 'NONE', #23007, .T. ) ;
#46239=CARTESIAN_POINT ( 'NONE',  ( -20.10180177043494254, -22.06666061677796975, -48.51647576933254413 ) ) ;
#46255=CARTESIAN_POINT ( 'NONE',  ( -36.91746825000000598, 2.428612866367529932E-14, -5.124999997268813168 ) ) ;
#46268=DIRECTION ( 'NONE',  ( -0.000000000000000000, -0.000000000000000000, 1.000000000000000000 ) ) ;
#46303=CARTESIAN_POINT ( 'NONE',  ( 11.40812507854755253, -35.11059874428192273, -10.52499999726881263 ) ) ;
#46306=CARTESIAN_POINT ( 'NONE',  ( 0.9201939147134639008, 8.788676749360311291, -64.01182165210214237 ) ) ;
#46314=CARTESIAN_POINT ( 'NONE',  ( -12.06727048284065340, 11.49022483853021903, -61.36479237366228290 ) ) ;
#46322=EDGE_LOOP ( 'NONE', ( #178316, #191055, #25603, #56540 ) ) ;
#46328=ORIENTED_EDGE ( 'NONE', *, *, #195370, .T. ) ;
#46452=CARTESIAN_POINT ( 'NONE',  ( -22.92000981050143338, 20.99774934350689648, -46.85949206705567605 ) ) ;
#46456=DIRECTION ( 'NONE',  ( 1.000000000000000000, 1.776356839400250465E-15, 0.000000000000000000 ) ) ;
#46465=VERTEX_POINT ( 'NONE', #110555 ) ;
#46487=ORIENTED_EDGE ( 'NONE', *, *, #37462, .F. ) ;
#46492=CARTESIAN_POINT ( 'NONE',  ( -7.122238460089373113, 1.425225664899916866, -62.29949481927938137 ) ) ;
#46503=CARTESIAN_POINT ( 'NONE',  ( 24.28797299941339816, -0.2180554607492743435, -56.78142080721293894 ) ) ;
#46561=CIRCLE ( 'NONE', #137351, 7.999999999999998224 ) ;
#46593=( GEOMETRIC_REPRESENTATION_CONTEXT ( 3 ) GLOBAL_UNCERTAINTY_ASSIGNED_CONTEXT ( ( #175317 ) ) GLOBAL_UNIT_ASSIGNED_CONTEXT ( ( #66915, #189290, #128579 ) ) REPRESENTATION_CONTEXT ( 'NONE', 'WORKASPACE' ) );
#46596=CARTESIAN_POINT ( 'NONE',  ( -16.70000000000002061, 1.759457951533292443E-13, -61.34707691135562868 ) ) ;
#46615=DIRECTION ( 'NONE',  ( -0.000000000000000000, -0.000000000000000000, 1.000000000000000000 ) ) ;
#46651=EDGE_CURVE ( 'NONE', #157648, #82035, #81934, .T. ) ;
#46659=LINE ( 'NONE', #141644, #156776 ) ;
#46676=AXIS2_PLACEMENT_3D ( 'NONE', #62740, #185106, #170929 ) ;
#46712=VERTEX_POINT ( 'NONE', #70161 ) ;
#46714=CARTESIAN_POINT ( 'NONE',  ( 37.99999999999999289, 2.893978650043524126E-14, -8.749999994537628112 ) ) ;
#46725=VECTOR ( 'NONE', #178142, 1000.000000000000000 ) ;
#46741=CARTESIAN_POINT ( 'NONE',  ( -12.49999999999997691, -89.99999999999997158, -15.00000000000000178 ) ) ;
#46752=CARTESIAN_POINT ( 'NONE',  ( -1.051486528467078463, -23.87412888849584647, -54.54543624665773649 ) ) ;
#46757=CARTESIAN_POINT ( 'NONE',  ( 17.55127066232087429, -16.58784780708363371, -56.88740615283250435 ) ) ;
#46762=CARTESIAN_POINT ( 'NONE',  ( -15.22409499613346640, 14.91565869316874959, -58.84910547483664800 ) ) ;
#46768=ORIENTED_EDGE ( 'NONE', *, *, #154789, .F. ) ;
#46771=CARTESIAN_POINT ( 'NONE',  ( 38.00000000000000711, -12.34694845685040754, -7.100000000000000533 ) ) ;
#46795=CARTESIAN_POINT ( 'NONE',  ( 16.63682861930254120, -37.51503513662888878, -19.06746308534681233 ) ) ;
#46826=ORIENTED_EDGE ( 'NONE', *, *, #149391, .F. ) ;
#46895=ADVANCED_FACE ( 'NONE', ( #22658 ), #40822, .T. ) ;
#46911=CARTESIAN_POINT ( 'NONE',  ( 17.18269478283314911, 17.18269478283310647, -54.21489346206828230 ) ) ;
#46913=DIRECTION ( 'NONE',  ( -0.000000000000000000, -0.000000000000000000, 1.000000000000000000 ) ) ;
#46950=ORIENTED_EDGE ( 'NONE', *, *, #6641, .T. ) ;
#46953=VECTOR ( 'NONE', #7393, 1000.000000000000000 ) ;
#46962=CARTESIAN_POINT ( 'NONE',  ( -18.60204571914025706, -35.35091242066509665, -18.26754506500681430 ) ) ;
#46988=CARTESIAN_POINT ( 'NONE',  ( 3.915140329348349990, 5.773271879485236013, -64.38756054665736883 ) ) ;
#47022=CARTESIAN_POINT ( 'NONE',  ( 22.02428569922084023, -33.37003842005633203, -23.53509012974128112 ) ) ;
#47043=ORIENTED_EDGE ( 'NONE', *, *, #8188, .T. ) ;
#47236=FACE_BOUND ( 'NONE', #72263, .T. ) ;
#47251=ORIENTED_EDGE ( 'NONE', *, *, #115833, .T. ) ;
#47259=CARTESIAN_POINT ( 'NONE',  ( -22.81625015709509441, -31.40387420917324590, -2.824999997268812901 ) ) ;
#47276=EDGE_CURVE ( 'NONE', #197536, #150928, #146999, .T. ) ;
#47298=EDGE_CURVE ( 'NONE', #104408, #140931, #185322, .T. ) ;
#47308=CARTESIAN_POINT ( 'NONE',  ( -28.81842663310010266, -24.98430004053108178, -11.52348593588107484 ) ) ;
#47320=CARTESIAN_POINT ( 'NONE',  ( 19.38985940809749309, -32.68077955211924035, -24.99999999999992895 ) ) ;
#47346=AXIS2_PLACEMENT_3D ( 'NONE', #29502, #47653, #13335 ) ;
#47456=FACE_OUTER_BOUND ( 'NONE', #157868, .T. ) ;
#47462=CARTESIAN_POINT ( 'NONE',  ( -24.06132300323553252, 0.8180345313833771170, -54.40060964255544462 ) ) ;
#47499=CARTESIAN_POINT ( 'NONE',  ( 20.43538597629129328, 20.43538597629121156, -64.92279855667830191 ) ) ;
#47532=EDGE_LOOP ( 'NONE', ( #56147, #187469, #49026, #38749, #75582 ) ) ;
#47533=EDGE_CURVE ( 'NONE', #56239, #183247, #7784, .T. ) ;
#47558=CARTESIAN_POINT ( 'NONE',  ( -22.72061570927963459, -33.65877872499205381, -17.91763856381928477 ) ) ;
#47564=CARTESIAN_POINT ( 'NONE',  ( -11.45643923738960446, -4.999999999999992895, -15.00000000000000000 ) ) ;
#47616=FACE_OUTER_BOUND ( 'NONE', #98820, .T. ) ;
#47633=EDGE_CURVE ( 'NONE', #177280, #143210, #13788, .T. ) ;
#47638=B_SPLINE_CURVE_WITH_KNOTS ( 'NONE', 3,
 ( #34471, #65790, #48657, #64809, #185168, #33479, #127459, #173989, #31489, #189165, #94139, #50637, #112299, #124485, #95137, #156826 ),
 .UNSPECIFIED., .F., .F.,
 ( 4, 2, 2, 2, 2, 2, 2, 4 ),
 ( 4.336808689942017736E-19, 0.005088736175617444152, 0.006360920219521812996, 0.007633104263426180106, 0.01017747235123490218, 0.01526620852685233766, 0.01781057661466104933, 0.02035494470246975926 ),
 .UNSPECIFIED. ) ;
#47641=VECTOR ( 'NONE', #21129, 1000.000000000000000 ) ;
#47644=EDGE_CURVE ( 'NONE', #22185, #126159, #43313, .T. ) ;
#47653=DIRECTION ( 'NONE',  ( -0.000000000000000000, 0.000000000000000000, 1.000000000000000000 ) ) ;
#47671=AXIS2_PLACEMENT_3D ( 'NONE', #33297, #45482, #14142 ) ;
#47695=FACE_OUTER_BOUND ( 'NONE', #145024, .T. ) ;
#47755=FACE_BOUND ( 'NONE', #143164, .T. ) ;
#47796=CARTESIAN_POINT ( 'NONE',  ( 8.779096689230840411, -37.67883572780987578, -23.98624440746760911 ) ) ;
#47800=ORIENTED_EDGE ( 'NONE', *, *, #71198, .F. ) ;
#47822=CYLINDRICAL_SURFACE ( 'NONE', #20775, 1.500000000000001332 ) ;
#47908=CARTESIAN_POINT ( 'NONE',  ( -28.47622644277399928, -25.16156846422451920, -16.68312038616162951 ) ) ;
#47910=CARTESIAN_POINT ( 'NONE',  ( 14.74842737557653116, 15.51017872335176762, -56.39952970130667609 ) ) ;
#47940=CIRCLE ( 'NONE', #131929, 216.0437394197456342 ) ;
#47952=VERTEX_POINT ( 'NONE', #14215 ) ;
#47963=CARTESIAN_POINT ( 'NONE',  ( -34.03190083852857128, -20.28298779506915750, -18.01673046680507184 ) ) ;
#48011=CARTESIAN_POINT ( 'NONE',  ( 22.81625015709509441, 31.40387420917330275, -5.324999997268812457 ) ) ;
#48020=CARTESIAN_POINT ( 'NONE',  ( 20.26331839697992265, -34.49854857074736714, -25.13492617046049560 ) ) ;
#48067=DIRECTION ( 'NONE',  ( 0.000000000000000000, 1.000000000000000000, 0.000000000000000000 ) ) ;
#48078=CARTESIAN_POINT ( 'NONE',  ( 2.500000000000000000, -105.0000000000000000, 7.000000000000003553 ) ) ;
#48228=DIRECTION ( 'NONE',  ( -1.000000000000000000, 0.000000000000000000, 0.000000000000000000 ) ) ;
#48229=CARTESIAN_POINT ( 'NONE',  ( 17.55241889863238569, -16.58432793727737575, -54.34081276845726904 ) ) ;
#48232=CARTESIAN_POINT ( 'NONE',  ( -0.1037895044722853544, -16.70000000000002061, -59.13370768023892055 ) ) ;
#48238=CARTESIAN_POINT ( 'NONE',  ( 20.43538597629128262, -20.43538597629122222, -49.67367017693150189 ) ) ;
#48254=CARTESIAN_POINT ( 'NONE',  ( -29.86685920354755197, -21.69954338932560134, -10.92499999726881299 ) ) ;
#48268=CARTESIAN_POINT ( 'NONE',  ( 4.313351365237948265, 4.313351365237946489, -62.50719930893269805 ) ) ;
#48291=CARTESIAN_POINT ( 'NONE',  ( -4.313351365237961588, 4.313351365237934942, -65.00100000000003320 ) ) ;
#48304=CARTESIAN_POINT ( 'NONE',  ( -36.91746825000001309, 11.99521256947798342, -7.224999997268814589 ) ) ;
#48305=CARTESIAN_POINT ( 'NONE',  ( 2.577820198429831642E-15, 9.100000000000001421, -63.95112321872120731 ) ) ;
#48307=VERTEX_POINT ( 'NONE', #127347 ) ;
#48314=CARTESIAN_POINT ( 'NONE',  ( 4.295634330582102756, -37.01983766409436072, -32.59999999999998721 ) ) ;
#48322=ORIENTED_EDGE ( 'NONE', *, *, #28066, .T. ) ;
#48374=ORIENTED_EDGE ( 'NONE', *, *, #186584, .F. ) ;
#48406=EDGE_CURVE ( 'NONE', #1611, #197947, #11297, .T. ) ;
#48453=CARTESIAN_POINT ( 'NONE',  ( 69.65682714487590488, -71.74905178543389184, -15.00000000000000178 ) ) ;
#48459=CARTESIAN_POINT ( 'NONE',  ( -21.36119649488922079, 0.4379334789938477690, -56.42482690868972384 ) ) ;
#48483=AXIS2_PLACEMENT_3D ( 'NONE', #81802, #7975, #69659 ) ;
#48495=CARTESIAN_POINT ( 'NONE',  ( -30.74264578624800492, 22.33583958711400186, -5.949999994537626513 ) ) ;
#48506=CARTESIAN_POINT ( 'NONE',  ( 21.30000000000002203, -0.1105695005019232124, -58.85720012050612127 ) ) ;
#48548=CARTESIAN_POINT ( 'NONE',  ( -1.467638476639070655, -30.74964850363294033, -47.27948696604328660 ) ) ;
#48561=VERTEX_POINT ( 'NONE', #178876 ) ;
#48581=EDGE_CURVE ( 'NONE', #74939, #166806, #88480, .T. ) ;
#48593=CARTESIAN_POINT ( 'NONE',  ( -13.90353822939980688, 0.7813480796680551954, -62.49831333862086780 ) ) ;
#48629=CARTESIAN_POINT ( 'NONE',  ( -3.874011537017815421, -5.374011537017722162, -62.41807096325323556 ) ) ;
#48657=CARTESIAN_POINT ( 'NONE',  ( -6.193113236902241248, -38.78391156914231175, -32.76858701579858035 ) ) ;
#48742=CYLINDRICAL_SURFACE ( 'NONE', #17757, 1.500000000000001332 ) ;
#48758=ORIENTED_EDGE ( 'NONE', *, *, #32194, .F. ) ;
#48761=CARTESIAN_POINT ( 'NONE',  ( 38.00000000000000711, -12.34694845685040754, -9.100000000000001421 ) ) ;
#48766=EDGE_CURVE ( 'NONE', #29006, #51296, #25997, .T. ) ;
#48777=EDGE_CURVE ( 'NONE', #76374, #111025, #193035, .T. ) ;
#48786=CARTESIAN_POINT ( 'NONE',  ( 23.57492084471138583, -29.96337447970307721, -16.79025860370820666 ) ) ;
#48790=ORIENTED_EDGE ( 'NONE', *, *, #62255, .T. ) ;
#48810=EDGE_CURVE ( 'NONE', #170287, #64113, #162687, .T. ) ;
#48888=DIRECTION ( 'NONE',  ( 1.000000000000000000, 0.000000000000000000, 0.000000000000000000 ) ) ;
#48896=CARTESIAN_POINT ( 'NONE',  ( 9.613975513199033429, 9.760750291312396243, -60.44446360152739572 ) ) ;
#48904=EDGE_CURVE ( 'NONE', #145335, #55466, #127416, .T. ) ;
#48938=ORIENTED_EDGE ( 'NONE', *, *, #18014, .F. ) ;
#48971=CARTESIAN_POINT ( 'NONE',  ( 21.11545612445405240, -20.04257545866360957, -49.42219586766479722 ) ) ;
#48974=CARTESIAN_POINT ( 'NONE',  ( 4.070821633784378335, 4.624734593510421377, -64.52277792523199196 ) ) ;
#48977=DIRECTION ( 'NONE',  ( -0.000000000000000000, -0.000000000000000000, 1.000000000000000000 ) ) ;
#48979=CARTESIAN_POINT ( 'NONE',  ( 22.89887992856522558, -20.94821244432957386, -50.23592918571483068 ) ) ;
#48988=DIRECTION ( 'NONE',  ( 1.000000000000000000, 0.000000000000000000, 0.000000000000000000 ) ) ;
#48997=CARTESIAN_POINT ( 'NONE',  ( -5.950531402560715689E-15, 38.81732327939063509, -5.124999997268813168 ) ) ;
#49003=EDGE_CURVE ( 'NONE', #110784, #143487, #75763, .T. ) ;
#49006=DIRECTION ( 'NONE',  ( 1.000000000000000000, 0.000000000000000000, 0.000000000000000000 ) ) ;
#49008=CARTESIAN_POINT ( 'NONE',  ( 16.25089620724480000, -36.76456463896338533, -23.32760966624454468 ) ) ;
#49026=ORIENTED_EDGE ( 'NONE', *, *, #181589, .T. ) ;
#49060=CARTESIAN_POINT ( 'NONE',  ( 36.91746824999999887, 11.99521256947799053, -8.024999997268814411 ) ) ;
#49064=DIRECTION ( 'NONE',  ( 1.000000000000000000, 0.000000000000000000, 0.000000000000000000 ) ) ;
#49087=CARTESIAN_POINT ( 'NONE',  ( 0.000000000000000000, -105.0000000000000000, 7.000000000000003553 ) ) ;
#49220=CARTESIAN_POINT ( 'NONE',  ( 1.500000000001822542, 22.62338797783493760, -55.49559142602143424 ) ) ;
#49223=CARTESIAN_POINT ( 'NONE',  ( 21.49604614807110536, -21.49604614807103786, -64.92279855667830191 ) ) ;
#49229=DIRECTION ( 'NONE',  ( -0.000000000000000000, 0.000000000000000000, 1.000000000000000000 ) ) ;
#49237=ORIENTED_EDGE ( 'NONE', *, *, #107092, .F. ) ;
#49242=CARTESIAN_POINT ( 'NONE',  ( -5.950531402560715689E-15, 38.81732327939063509, -7.624999997268814056 ) ) ;
#49290=CARTESIAN_POINT ( 'NONE',  ( -29.86685920354755552, 21.69954338932564397, -5.324999997268814234 ) ) ;
#49313=VERTEX_POINT ( 'NONE', #117181 ) ;
#49375=LINE ( 'NONE', #110048, #63938 ) ;
#49423=AXIS2_PLACEMENT_3D ( 'NONE', #110265, #186137, #66747 ) ;
#49441=CARTESIAN_POINT ( 'NONE',  ( 6.874011537017776341, -5.374011537017756801, -61.98469907122333922 ) ) ;
#49476=CARTESIAN_POINT ( 'NONE',  ( 30.74264578624799782, 22.33583958711400541, -2.549999994537626602 ) ) ;
#49487=CARTESIAN_POINT ( 'NONE',  ( 24.06642195515791371, -0.8101246706333994352, -56.93999021579657693 ) ) ;
#49490=CARTESIAN_POINT ( 'NONE',  ( -1.272595016298593507, -31.21487366219225734, -49.98150452412668443 ) ) ;
#49532=EDGE_CURVE ( 'NONE', #40299, #56239, #179963, .T. ) ;
#49560=DIRECTION ( 'NONE',  ( -1.000000000000000000, 0.000000000000000000, 0.000000000000000000 ) ) ;
#49564=AXIS2_PLACEMENT_3D ( 'NONE', #176177, #129633, #80159 ) ;
#49576=CARTESIAN_POINT ( 'NONE',  ( 15.20000000000001883, -5.133579287443888301E-14, -64.92279855667830191 ) ) ;
#49596=CARTESIAN_POINT ( 'NONE',  ( -3.573655867282028392E-15, 2.428612866367529932E-14, -25.00000000000000000 ) ) ;
#49599=CARTESIAN_POINT ( 'NONE',  ( -5.883457575057126299, -36.84471599068518799, -32.38015766500866732 ) ) ;
#49611=CARTESIAN_POINT ( 'NONE',  ( 8.673617379884035472E-16, -7.600000000000007638, -64.92279855667830191 ) ) ;
#49641=DIRECTION ( 'NONE',  ( 0.000000000000000000, 0.000000000000000000, 1.000000000000000000 ) ) ;
#49693=CARTESIAN_POINT ( 'NONE',  ( 0.000000000000000000, 0.000000000000000000, -64.92279855667830191 ) ) ;
#49728=CARTESIAN_POINT ( 'NONE',  ( 22.82566123211450915, -22.19887561992280567, -45.74155842934298022 ) ) ;
#49732=FACE_BOUND ( 'NONE', #136721, .T. ) ;
#49773=CARTESIAN_POINT ( 'NONE',  ( 34.03190083852023662, -20.28298779507398208, -18.01673046680643253 ) ) ;
#49777=ORIENTED_EDGE ( 'NONE', *, *, #28831, .F. ) ;
#49803=ORIENTED_EDGE ( 'NONE', *, *, #15852, .T. ) ;
#49816=AXIS2_PLACEMENT_3D ( 'NONE', #178310, #39773, #175299 ) ;
#49835=FACE_OUTER_BOUND ( 'NONE', #3595, .T. ) ;
#49871=VECTOR ( 'NONE', #19047, 1000.000000000000000 ) ;
#49884=CARTESIAN_POINT ( 'NONE',  ( 11.48863819084122184, 12.06828707866188921, -59.15275318406540350 ) ) ;
#49940=CARTESIAN_POINT ( 'NONE',  ( -30.04893132686769519, -22.76590847478283663, -19.45433810172459488 ) ) ;
#49944=EDGE_CURVE ( 'NONE', #76374, #22413, #199276, .T. ) ;
#49963=CARTESIAN_POINT ( 'NONE',  ( -31.81624771892549575, 0.5097844185668732875, -45.77220262091587699 ) ) ;
#49966=CARTESIAN_POINT ( 'NONE',  ( 4.242615737635166973, 4.384086992840732222, -64.53213882399994361 ) ) ;
#49971=CARTESIAN_POINT ( 'NONE',  ( 22.11731296686191328, -20.12440949879982455, -51.56823826216871254 ) ) ;
#49986=ORIENTED_EDGE ( 'NONE', *, *, #3940, .T. ) ;
#49988=CARTESIAN_POINT ( 'NONE',  ( -11.40812507854755609, 35.11059874428196537, -5.024999997268813523 ) ) ;
#49998=CARTESIAN_POINT ( 'NONE',  ( 17.75813068129455274, -35.78296932995310442, -27.23805928211041660 ) ) ;
#50009=AXIS2_PLACEMENT_3D ( 'NONE', #61288, #170466, #122958 ) ;
#50049=AXIS2_PLACEMENT_3D ( 'NONE', #30700, #16523, #152057 ) ;
#50053=CARTESIAN_POINT ( 'NONE',  ( 29.86685920354754487, 21.69954338932564752, -1.424999997268813212 ) ) ;
#50089=CARTESIAN_POINT ( 'NONE',  ( -38.00000000000000711, -12.34694845685042708, -1.899999999999999689 ) ) ;
#50132=CARTESIAN_POINT ( 'NONE',  ( 0.000000000000000000, -105.0000000000000000, -23.00000000000000000 ) ) ;
#50162=EDGE_CURVE ( 'NONE', #23346, #48561, #35246, .T. ) ;
#50244=CARTESIAN_POINT ( 'NONE',  ( -11.40812507854755609, 35.11059874428196537, -9.524999997268816188 ) ) ;
#50278=ADVANCED_FACE ( 'NONE', ( #173645 ), #35114, .F. ) ;
#50292=CARTESIAN_POINT ( 'NONE',  ( 29.86685920354754487, 21.69954338932564752, -1.924999997268813212 ) ) ;
#50299=CARTESIAN_POINT ( 'NONE',  ( -12.25159394783734434, 10.91551912637959276, -61.48002405683646288 ) ) ;
#50361=ORIENTED_EDGE ( 'NONE', *, *, #133623, .T. ) ;
#50374=CIRCLE ( 'NONE', #150556, 6.100000000000006750 ) ;
#50383=CARTESIAN_POINT ( 'NONE',  ( 0.000000000000000000, 0.000000000000000000, -15.00000000000000000 ) ) ;
#50401=CARTESIAN_POINT ( 'NONE',  ( 4.000000000000000888, -165.0000000000000000, 12.00000000000000355 ) ) ;
#50438=DIRECTION ( 'NONE',  ( 6.391086490440865492E-16, 1.000000000000000000, -0.000000000000000000 ) ) ;
#50460=CARTESIAN_POINT ( 'NONE',  ( 15.18304462349147599, -14.93970425505549038, -56.46919128290398504 ) ) ;
#50477=CARTESIAN_POINT ( 'NONE',  ( -30.74264578624800492, 22.33583958711400186, -3.949999994537626957 ) ) ;
#50487=DIRECTION ( 'NONE',  ( -0.000000000000000000, -0.000000000000000000, -1.000000000000000000 ) ) ;
#50489=CARTESIAN_POINT ( 'NONE',  ( -1.478515647795532795, -30.09553654342102291, -51.30846887466859840 ) ) ;
#50501=CARTESIAN_POINT ( 'NONE',  ( -20.03347751555784839, -21.15125157081075002, -49.39869787917044874 ) ) ;
#50533=CARTESIAN_POINT ( 'NONE',  ( -0.1356448107282722249, -31.90000000000003411, -45.64921306006599622 ) ) ;
#50545=CARTESIAN_POINT ( 'NONE',  ( -13.37225149056313356, -38.04021455642293859, -24.47500528307575962 ) ) ;
#50568=DIRECTION ( 'NONE',  ( 1.000000000000000000, 0.000000000000000000, 0.000000000000000000 ) ) ;
#50637=CARTESIAN_POINT ( 'NONE',  ( -17.36633513277073249, -35.95409897417807343, -27.53902325179330646 ) ) ;
#50644=AXIS2_PLACEMENT_3D ( 'NONE', #147656, #104140, #9144 ) ;
#50663=AXIS2_PLACEMENT_3D ( 'NONE', #154389, #169556, #187734 ) ;
#50694=VERTEX_POINT ( 'NONE', #74195 ) ;
#50704=AXIS2_PLACEMENT_3D ( 'NONE', #193026, #178867, #56506 ) ;
#50706=CARTESIAN_POINT ( 'NONE',  ( 15.93273212980866482, -1.322671946311529290, -61.66661032175887414 ) ) ;
#50723=DIRECTION ( 'NONE',  ( -0.000000000000000000, -0.000000000000000000, 1.000000000000000000 ) ) ;
#50738=CARTESIAN_POINT ( 'NONE',  ( -13.70000000000001528, 1.443387660838688656E-13, -60.44446360152740283 ) ) ;
#50787=TOROIDAL_SURFACE ( 'NONE', #70135, 69.99999999999998579, 10.00000000000000000 ) ;
#50812=AXIS2_PLACEMENT_3D ( 'NONE', #13201, #103214, #122339 ) ;
#50882=CARTESIAN_POINT ( 'NONE',  ( -20.17688442456149644, -20.77425831086903329, -52.59230516607028250 ) ) ;
#50929=CIRCLE ( 'NONE', #118802, 10.00000000000000000 ) ;
#50932=ORIENTED_EDGE ( 'NONE', *, *, #150147, .F. ) ;
#50951=CARTESIAN_POINT ( 'NONE',  ( -3.573655867282028392E-15, 2.428612866367529932E-14, -18.00000000000000000 ) ) ;
#50956=CARTESIAN_POINT ( 'NONE',  ( -29.14368513529649007, 0.8274645171316362680, -49.37167794572891211 ) ) ;
#50962=DIRECTION ( 'NONE',  ( 0.000000000000000000, 0.000000000000000000, 1.000000000000000000 ) ) ;
#50979=CARTESIAN_POINT ( 'NONE',  ( 29.86685920354754487, 21.69954338932564752, -1.424999997268813212 ) ) ;
#50989=CARTESIAN_POINT ( 'NONE',  ( 27.75718128995143630, -28.53842127824106356, -16.93139376985908129 ) ) ;
#51008=VERTEX_POINT ( 'NONE', #299 ) ;
#51039=CARTESIAN_POINT ( 'NONE',  ( 11.40812507854754365, 35.11059874428196537, -9.724999997268813701 ) ) ;
#51071=CARTESIAN_POINT ( 'NONE',  ( -30.40000000000003766, 3.080147572466333233E-13, -64.92279855667830191 ) ) ;
#51073=CARTESIAN_POINT ( 'NONE',  ( 28.90000000000004476, 0.000000000000000000, -52.65483682830183199 ) ) ;
#51155=ADVANCED_FACE ( 'NONE', ( #124645 ), #47822, .F. ) ;
#51184=DIRECTION ( 'NONE',  ( 1.000000000000000000, 0.000000000000000000, 0.000000000000000000 ) ) ;
#51186=CARTESIAN_POINT ( 'NONE',  ( 19.99074948409479902, 21.30378117525434334, -49.30207733784023105 ) ) ;
#51191=DIRECTION ( 'NONE',  ( 0.000000000000000000, 0.000000000000000000, 1.000000000000000000 ) ) ;
#51195=DIRECTION ( 'NONE',  ( -1.000000000000000000, 0.000000000000000000, 0.000000000000000000 ) ) ;
#51204=DIRECTION ( 'NONE',  ( 1.000000000000000000, 0.000000000000000000, 3.469446951953612217E-15 ) ) ;
#51210=CARTESIAN_POINT ( 'NONE',  ( 22.99604614807110181, -21.49604614807103786, -64.92279855667830191 ) ) ;
#51225=CARTESIAN_POINT ( 'NONE',  ( 36.91746824999999177, 2.880721459617395097E-14, -10.12499999726881583 ) ) ;
#51241=AXIS2_PLACEMENT_3D ( 'NONE', #190551, #48067, #80366 ) ;
#51273=CARTESIAN_POINT ( 'NONE',  ( 22.81625015709510151, -31.40387420917324590, -6.424999997268812102 ) ) ;
#51284=CARTESIAN_POINT ( 'NONE',  ( 14.75151636811257916, 15.50344475828853064, -58.79419791951498553 ) ) ;
#51296=VERTEX_POINT ( 'NONE', #34399 ) ;
#51423=CARTESIAN_POINT ( 'NONE',  ( -9.248023074035629065, -10.74802307403544077, -60.25555373585994090 ) ) ;
#51440=CARTESIAN_POINT ( 'NONE',  ( -29.02171288343480526, 0.6023940538451412197, -52.52077797743537246 ) ) ;
#51444=DIRECTION ( 'NONE',  ( -1.000000000000000000, -0.000000000000000000, -0.000000000000000000 ) ) ;
#51452=ORIENTED_EDGE ( 'NONE', *, *, #145235, .T. ) ;
#51455=FACE_OUTER_BOUND ( 'NONE', #171861, .T. ) ;
#51464=CIRCLE ( 'NONE', #148475, 38.00000000000000000 ) ;
#51472=CARTESIAN_POINT ( 'NONE',  ( 19.96964676835936459, -32.33678545050543107, -24.48363814647527548 ) ) ;
#51515=CARTESIAN_POINT ( 'NONE',  ( -1.481880339025519300, -30.11448378070094734, -48.12989299794422493 ) ) ;
#51527=CARTESIAN_POINT ( 'NONE',  ( -21.44681783660697860, -33.76292609719497761, -24.06782133911154631 ) ) ;
#51539=CARTESIAN_POINT ( 'NONE',  ( 6.434671708797603529, -6.434671708797564449, -63.95112321872120731 ) ) ;
#51550=CARTESIAN_POINT ( 'NONE',  ( 37.99999999999991473, -12.34694845685052833, -8.849999994537625980 ) ) ;
#51579=CARTESIAN_POINT ( 'NONE',  ( 0.000000000000000000, 0.000000000000000000, -49.67367017693150189 ) ) ;
#51582=CARTESIAN_POINT ( 'NONE',  ( -7.819668024151573249, -36.54656901728082374, -31.88218832179850182 ) ) ;
#51668=EDGE_CURVE ( 'NONE', #44025, #243, #11138, .T. ) ;
#51688=CARTESIAN_POINT ( 'NONE',  ( 0.4356378768753526032, 24.23951953793845249, -54.26206177644314010 ) ) ;
#51750=CARTESIAN_POINT ( 'NONE',  ( -30.74264578624800492, 22.33583958711400186, -9.949999994537627401 ) ) ;
#51753=CARTESIAN_POINT ( 'NONE',  ( 25.83444802367794679, -27.47999234037484939, -20.36589038153131881 ) ) ;
#51820=DIRECTION ( 'NONE',  ( -0.000000000000000000, -0.000000000000000000, 1.000000000000000000 ) ) ;
#51865=CARTESIAN_POINT ( 'NONE',  ( 9.278585747845305320, 10.38518860439147495, -60.35672204601533508 ) ) ;
#51909=ORIENTED_EDGE ( 'NONE', *, *, #90658, .F. ) ;
#51910=CARTESIAN_POINT ( 'NONE',  ( -5.000000000000000888, 4.999999999999999112, -18.00000000000000000 ) ) ;
#51917=ORIENTED_EDGE ( 'NONE', *, *, #42762, .F. ) ;
#51919=CARTESIAN_POINT ( 'NONE',  ( -33.17841651221153398, -18.64421535752885362, -21.40882326906567812 ) ) ;
#51936=DIRECTION ( 'NONE',  ( 0.000000000000000000, 1.000000000000000000, 0.000000000000000000 ) ) ;
#51944=CARTESIAN_POINT ( 'NONE',  ( 4.704672000039139768, 6.719938155502468646, -64.14994679864911120 ) ) ;
#51945=CARTESIAN_POINT ( 'NONE',  ( -38.00000000000004263, -12.34694845685037023, -7.649999994537626691 ) ) ;
#51948=DIRECTION ( 'NONE',  ( 1.000000000000000000, 0.000000000000000000, 0.000000000000000000 ) ) ;
#51967=CARTESIAN_POINT ( 'NONE',  ( -5.950531402560715689E-15, 38.81732327939063509, -1.124999997268812946 ) ) ;
#51978=CARTESIAN_POINT ( 'NONE',  ( 31.90410663231038768, -24.66877891592865879, -17.57859634139417082 ) ) ;
#52015=FACE_OUTER_BOUND ( 'NONE', #24120, .T. ) ;
#52024=CARTESIAN_POINT ( 'NONE',  ( -15.34294242576431522, -17.41135957075415774, -55.09099524710079976 ) ) ;
#52027=CARTESIAN_POINT ( 'NONE',  ( -29.86685920354755552, 21.69954338932564397, -9.324999997268813345 ) ) ;
#52107=CARTESIAN_POINT ( 'NONE',  ( 37.99999999999999289, 2.893978650043524126E-14, -3.000000000000000000 ) ) ;
#52114=EDGE_CURVE ( 'NONE', #106917, #45831, #137905, .T. ) ;
#52161=EDGE_LOOP ( 'NONE', ( #134378, #82222, #75294, #67690 ) ) ;
#52200=CARTESIAN_POINT ( 'NONE',  ( -36.91746825000000598, 2.428612866367529932E-14, -4.624999997268814056 ) ) ;
#52230=DIRECTION ( 'NONE',  ( -0.000000000000000000, -0.000000000000000000, 1.000000000000000000 ) ) ;
#52257=CARTESIAN_POINT ( 'NONE',  ( 31.90000000000003411, -0.1356448107283860505, -45.64921306006599622 ) ) ;
#52260=CARTESIAN_POINT ( 'NONE',  ( -22.81625015709510507, 31.40387420917330275, -3.424999997268813434 ) ) ;
#52261=CARTESIAN_POINT ( 'NONE',  ( -22.97983228106267362, 21.73741105231462711, -49.48322453030140622 ) ) ;
#52271=CARTESIAN_POINT ( 'NONE',  ( 14.79957802611874662, 15.40597107458649973, -58.81775317265829273 ) ) ;
#52283=EDGE_LOOP ( 'NONE', ( #192030, #90332, #25436, #165878, #150554, #6692 ) ) ;
#52391=ORIENTED_EDGE ( 'NONE', *, *, #31320, .T. ) ;
#52407=CARTESIAN_POINT ( 'NONE',  ( -9.164641033549692395, -36.31047332450869902, -31.46032839770261091 ) ) ;
#52426=CARTESIAN_POINT ( 'NONE',  ( 11.74264578624799427, 36.14014761921585972, -0.5999999999999999778 ) ) ;
#52429=CARTESIAN_POINT ( 'NONE',  ( -31.06299995236812350, 1.355922687059702980, -50.16575868250044579 ) ) ;
#52448=CARTESIAN_POINT ( 'NONE',  ( 38.00000000000000711, -12.34694845685040754, -2.849999994537626424 ) ) ;
#52462=CARTESIAN_POINT ( 'NONE',  ( 27.77250826529498440, -25.57832283906988025, -20.68473525701016413 ) ) ;
#52504=CARTESIAN_POINT ( 'NONE',  ( -0.6278704076484974417, -29.03295818733088041, -49.50940399778497891 ) ) ;
#52515=CARTESIAN_POINT ( 'NONE',  ( -20.26331839699024329, -34.49854857074117120, -25.13492617047004174 ) ) ;
#52527=LINE ( 'NONE', #37363, #2196 ) ;
#52535=EDGE_CURVE ( 'NONE', #17032, #40299, #90750, .T. ) ;
#52585=DIRECTION ( 'NONE',  ( 1.000000000000000000, 0.000000000000000000, 0.000000000000000000 ) ) ;
#52650=CARTESIAN_POINT ( 'NONE',  ( -16.02140599805581900, -17.62553472373751617, -57.13537817852984801 ) ) ;
#52672=CARTESIAN_POINT ( 'NONE',  ( 9.841528761215755594, -38.18405872352758479, -31.73089324721042104 ) ) ;
#52699=CYLINDRICAL_SURFACE ( 'NONE', #21807, 2.500000000000000000 ) ;
#52702=CARTESIAN_POINT ( 'NONE',  ( -37.45873412500000654, 2.428612866367529932E-14, -1.437499995903219974 ) ) ;
#52713=CARTESIAN_POINT ( 'NONE',  ( -13.90528855463212388, 0.7844626028951359187, -60.35633530387643475 ) ) ;
#52744=CARTESIAN_POINT ( 'NONE',  ( 31.47295357026365892, -21.29310327861803387, -24.13113353488660096 ) ) ;
#52747=ORIENTED_EDGE ( 'NONE', *, *, #7790, .T. ) ;
#52769=DIRECTION ( 'NONE',  ( -0.000000000000000000, -0.000000000000000000, 1.000000000000000000 ) ) ;
#52799=EDGE_CURVE ( 'NONE', #64113, #190965, #121194, .T. ) ;
#52812=CARTESIAN_POINT ( 'NONE',  ( -37.45873412500000654, 2.428612866367529932E-14, -10.31249999863440792 ) ) ;
#52908=CARTESIAN_POINT ( 'NONE',  ( -9.396967334131923977, -10.08899614358906405, -62.54888902377756210 ) ) ;
#52922=ORIENTED_EDGE ( 'NONE', *, *, #61218, .T. ) ;
#52933=CARTESIAN_POINT ( 'NONE',  ( 4.619345608252475976, 6.673977169394437858, -64.16796455867367399 ) ) ;
#52955=CARTESIAN_POINT ( 'NONE',  ( 36.91746824999999887, 11.99521256947799053, -7.524999997268814411 ) ) ;
#52978=VERTEX_POINT ( 'NONE', #138357 ) ;
#52986=EDGE_LOOP ( 'NONE', ( #82094, #96419, #64161, #189977 ) ) ;
#53018=CARTESIAN_POINT ( 'NONE',  ( 22.81625015709509441, 31.40387420917330275, -1.324999997268813123 ) ) ;
#53019=CARTESIAN_POINT ( 'NONE',  ( 37.99999999999999289, 2.893978650043524126E-14, -2.749999994537626780 ) ) ;
#53036=CIRCLE ( 'NONE', #43397, 4.000000000000000888 ) ;
#53086=ORIENTED_EDGE ( 'NONE', *, *, #160165, .F. ) ;
#53136=VERTEX_POINT ( 'NONE', #75682 ) ;
#53157=CIRCLE ( 'NONE', #166206, 38.00000000000002132 ) ;
#53168=CYLINDRICAL_SURFACE ( 'NONE', #134687, 31.90000000000003411 ) ;
#53193=ORIENTED_EDGE ( 'NONE', *, *, #67401, .T. ) ;
#53197=CARTESIAN_POINT ( 'NONE',  ( 36.91746824999999177, 2.880721459617395097E-14, -1.624999997268813390 ) ) ;
#53204=ORIENTED_EDGE ( 'NONE', *, *, #147752, .F. ) ;
#53207=CARTESIAN_POINT ( 'NONE',  ( 29.44683875480690816, -27.07775549506662927, -16.45954463943772339 ) ) ;
#53259=EDGE_CURVE ( 'NONE', #128045, #198744, #45362, .T. ) ;
#53269=CARTESIAN_POINT ( 'NONE',  ( 14.91565869316880288, 15.22409499613341133, -58.84910547483664089 ) ) ;
#53273=EDGE_LOOP ( 'NONE', ( #25713, #164884, #8216, #110465, #44728, #175257, #420, #147555, #134766, #57537, #74269, #76040 ) ) ;
#53348=AXIS2_PLACEMENT_3D ( 'NONE', #69022, #114516, #176217 ) ;
#53349=DIRECTION ( 'NONE',  ( 0.000000000000000000, 0.000000000000000000, -1.000000000000000000 ) ) ;
#53405=DIRECTION ( 'NONE',  ( 1.000000000000000000, 0.000000000000000000, 0.000000000000000000 ) ) ;
#53430=VECTOR ( 'NONE', #107558, 1000.000000000000000 ) ;
#53455=FACE_OUTER_BOUND ( 'NONE', #170347, .T. ) ;
#53461=CARTESIAN_POINT ( 'NONE',  ( -11.30153831258470731, -180.0000000000000000, -25.00000000000000000 ) ) ;
#53486=CARTESIAN_POINT ( 'NONE',  ( -17.18269478283316332, 17.18269478283309226, -54.21489346206828230 ) ) ;
#53518=CARTESIAN_POINT ( 'NONE',  ( -3.503282210674341979, -48.86437366581480291, -24.99999999999999289 ) ) ;
#53519=VERTEX_POINT ( 'NONE', #139971 ) ;
#53530=CARTESIAN_POINT ( 'NONE',  ( 9.550175731184127770, 9.839468975293851116, -62.57644703671204667 ) ) ;
#53556=B_SPLINE_CURVE_WITH_KNOTS ( 'NONE', 3,
 ( #76565, #138240, #19866, #148960, #127029, #188736, #25631, #21863, #132780, #144194, #80533, #194467, #34049, #55938 ),
 .UNSPECIFIED., .F., .F.,
 ( 4, 2, 2, 2, 2, 2, 4 ),
 ( 1.971390914159136004E-07, 0.0002964243498305583948, 0.0005926515605697007128, 0.0008888787713088428140, 0.001185105982047984698, 0.001777560403526266515, 0.002370014825004548333 ),
 .UNSPECIFIED. ) ;
#53593=DIRECTION ( 'NONE',  ( 1.000000000000000000, 0.000000000000000000, 0.000000000000000000 ) ) ;
#53619=CARTESIAN_POINT ( 'NONE',  ( -37.66961640367473052, -4.999999999999976019, -15.00000000000000000 ) ) ;
#53676=EDGE_LOOP ( 'NONE', ( #181094, #130830, #102292, #27686, #14492 ) ) ;
#53680=CYLINDRICAL_SURFACE ( 'NONE', #105355, 24.30000000000003268 ) ;
#53692=EDGE_CURVE ( 'NONE', #515, #85313, #130747, .T. ) ;
#53708=CARTESIAN_POINT ( 'NONE',  ( 21.49604614807110536, -21.49604614807103786, -64.92279855667830191 ) ) ;
#53718=CARTESIAN_POINT ( 'NONE',  ( -38.00000000000000711, -12.34694845685042708, -5.649999994537625803 ) ) ;
#53729=CIRCLE ( 'NONE', #79561, 13.70000000000001528 ) ;
#53736=B_SPLINE_CURVE_WITH_KNOTS ( 'NONE', 3,
 ( #40758, #70095, #146933, #101409, #71093, #23595, #195458, #26602, #85242, #178283, #147942, #9428, #162099, #11437, #132760, #116594 ),
 .UNSPECIFIED., .F., .F.,
 ( 4, 2, 2, 2, 2, 2, 2, 4 ),
 ( 0.003057157445971939082, 0.003802480048122062334, 0.004175141349197131549, 0.004547802650272200764, 0.004920463951347270846, 0.005293125252422339194, 0.005665786553497409277, 0.006038447854572478492 ),
 .UNSPECIFIED. ) ;
#53759=CARTESIAN_POINT ( 'NONE',  ( 31.56233167169124343, -22.40491105030149299, -17.28239568967847362 ) ) ;
#53785=EDGE_CURVE ( 'NONE', #196359, #126376, #65127, .T. ) ;
#53802=EDGE_CURVE ( 'NONE', #243, #44025, #127563, .T. ) ;
#53911=EDGE_LOOP ( 'NONE', ( #22303, #183775 ) ) ;
#53915=ORIENTED_EDGE ( 'NONE', *, *, #72679, .F. ) ;
#53957=CARTESIAN_POINT ( 'NONE',  ( 33.33394450212942672, -22.11087592608185659, -23.55754414195986257 ) ) ;
#53974=CARTESIAN_POINT ( 'NONE',  ( 36.91746825000000598, -11.99521256947793546, -7.724999997268812812 ) ) ;
#53997=EDGE_LOOP ( 'NONE', ( #11453, #11807, #159310, #178570 ) ) ;
#54004=ORIENTED_EDGE ( 'NONE', *, *, #181354, .F. ) ;
#54020=AXIS2_PLACEMENT_3D ( 'NONE', #49223, #189731, #66369 ) ;
#54032=DIRECTION ( 'NONE',  ( 0.07151044867601312471, 0.9974398506828144884, 0.000000000000000000 ) ) ;
#54035=CARTESIAN_POINT ( 'NONE',  ( 29.86685920354754487, 21.69954338932564752, -9.424999997268814766 ) ) ;
#54092=DIRECTION ( 'NONE',  ( 0.000000000000000000, 0.000000000000000000, -1.000000000000000000 ) ) ;
#54118=CIRCLE ( 'NONE', #150981, 38.00000000000000000 ) ;
#54160=AXIS2_PLACEMENT_3D ( 'NONE', #10933, #71596, #133262 ) ;
#54198=CARTESIAN_POINT ( 'NONE',  ( -26.37337922943865109, -29.71119707698751000, -20.32121347158689773 ) ) ;
#54209=CARTESIAN_POINT ( 'NONE',  ( -22.81625015709510507, 31.40387420917330275, -0.9249999972688132122 ) ) ;
#54220=CARTESIAN_POINT ( 'NONE',  ( 28.06518720328419647, -28.50306805876740412, -15.18214172726662881 ) ) ;
#54266=CARTESIAN_POINT ( 'NONE',  ( 31.20457203169702964, -1.278449583442190729, -46.64972497815392671 ) ) ;
#54356=CARTESIAN_POINT ( 'NONE',  ( -11.80868324581545714, -11.80868324581525997, -59.13370768023891344 ) ) ;
#54395=ADVANCED_FACE ( 'NONE', ( #189484 ), #95462, .F. ) ;
#54418=AXIS2_PLACEMENT_3D ( 'NONE', #39581, #162929, #38592 ) ;
#54435=CARTESIAN_POINT ( 'NONE',  ( -28.97745891950396313, 0.4911207797137864262, -52.56957762865166472 ) ) ;
#54454=CARTESIAN_POINT ( 'NONE',  ( 30.74264578624800137, -22.33583958711395212, -6.949999994537627401 ) ) ;
#54463=DIRECTION ( 'NONE',  ( -0.000000000000000000, -0.000000000000000000, 1.000000000000000000 ) ) ;
#54467=LINE ( 'NONE', #98951, #47641 ) ;
#54471=CARTESIAN_POINT ( 'NONE',  ( 4.647474457565486646E-15, -28.90000000000004476, -52.65483682830183199 ) ) ;
#54502=CARTESIAN_POINT ( 'NONE',  ( 22.81625015709509441, 31.40387420917330275, -1.824999997268813345 ) ) ;
#54503=CARTESIAN_POINT ( 'NONE',  ( -1.469699867061801779, -22.44763431097443274, -58.07555020237587939 ) ) ;
#54512=DIRECTION ( 'NONE',  ( -0.000000000000000000, -0.000000000000000000, -1.000000000000000000 ) ) ;
#54525=CARTESIAN_POINT ( 'NONE',  ( -10.44694540017202478, -45.05842955090937352, -23.63933302999038588 ) ) ;
#54539=CARTESIAN_POINT ( 'NONE',  ( 21.30000000000002203, -0.1123844339349802934, -56.46919128290399925 ) ) ;
#54562=EDGE_CURVE ( 'NONE', #53519, #21583, #35783, .T. ) ;
#54590=CARTESIAN_POINT ( 'NONE',  ( 5.374011537017778117, -5.374011537017756801, -64.92279855667830191 ) ) ;
#54650=CARTESIAN_POINT ( 'NONE',  ( 11.30153831258470731, -180.0000000000000000, -25.00000000000000000 ) ) ;
#54666=ORIENTED_EDGE ( 'NONE', *, *, #23760, .T. ) ;
#54673=CARTESIAN_POINT ( 'NONE',  ( 6.193113236902296315, -38.78391156914228333, -32.76858701579856614 ) ) ;
#54692=ORIENTED_EDGE ( 'NONE', *, *, #28742, .F. ) ;
#54701=CARTESIAN_POINT ( 'NONE',  ( 20.02676387111008438, 21.85243030949935061, -51.86007293692900078 ) ) ;
#54706=CARTESIAN_POINT ( 'NONE',  ( 37.99999999999999289, 12.34694845685046793, -4.899999999999999467 ) ) ;
#54712=DIRECTION ( 'NONE',  ( 0.000000000000000000, 0.000000000000000000, 1.000000000000000000 ) ) ;
#54726=ORIENTED_EDGE ( 'NONE', *, *, #24668, .F. ) ;
#54740=ORIENTED_EDGE ( 'NONE', *, *, #55706, .F. ) ;
#54821=CARTESIAN_POINT ( 'NONE',  ( 0.9268384597861692997, 6.404133089829842973, -64.47363563910111850 ) ) ;
#54903=B_SPLINE_CURVE_WITH_KNOTS ( 'NONE', 3,
 ( #29944, #86884, #107753, #10059, #71719, #14774, #41392, #194088, #199791, #122929, #55550, #178917, #77425, #62242 ),
 .UNSPECIFIED., .F., .F.,
 ( 4, 2, 2, 2, 2, 2, 4 ),
 ( 1.970604704964099883E-07, 0.0003055224468752419631, 0.0006108478332799875199, 0.001221498606089477766, 0.001832149378898968121, 0.002137474765303713949, 0.002442800151708459776 ),
 .UNSPECIFIED. ) ;
#54907=ORIENTED_EDGE ( 'NONE', *, *, #53692, .T. ) ;
#54913=CARTESIAN_POINT ( 'NONE',  ( -9.687362902255793884, -9.687362902255632235, -64.92279855667830191 ) ) ;
#54922=CARTESIAN_POINT ( 'NONE',  ( -69.65682714487590488, -71.74905178543390605, -25.00000000000000000 ) ) ;
#54938=ORIENTED_EDGE ( 'NONE', *, *, #34762, .F. ) ;
#54949=CARTESIAN_POINT ( 'NONE',  ( 28.47622644277404191, -25.16156846422445881, -16.68312038616162241 ) ) ;
#54951=CARTESIAN_POINT ( 'NONE',  ( 16.61636759701972466, -0.5040881997803988712, -59.17093420172795959 ) ) ;
#54967=ORIENTED_EDGE ( 'NONE', *, *, #17432, .T. ) ;
#54968=ADVANCED_FACE ( 'NONE', ( #100447 ), #10459, .T. ) ;
#54971=CARTESIAN_POINT ( 'NONE',  ( 11.40812507854754365, 35.11059874428196537, -7.224999997268813701 ) ) ;
#54976=CARTESIAN_POINT ( 'NONE',  ( 0.5042224564900709138, 16.61632169229824285, -59.17095462602203071 ) ) ;
#54980=CARTESIAN_POINT ( 'NONE',  ( 34.32499373855911529, -22.49325299167919567, -18.44817765300317802 ) ) ;
#55026=DIRECTION ( 'NONE',  ( -0.000000000000000000, -0.000000000000000000, 1.000000000000000000 ) ) ;
#55029=CARTESIAN_POINT ( 'NONE',  ( 3.556970738554033499E-15, -38.81732327939057825, -4.124999997268814056 ) ) ;
#55034=CARTESIAN_POINT ( 'NONE',  ( -11.80868324581545714, -11.80868324581525997, -59.13370768023891344 ) ) ;
#55067=EDGE_CURVE ( 'NONE', #55466, #171824, #141238, .T. ) ;
#55093=EDGE_CURVE ( 'NONE', #140931, #145198, #174904, .T. ) ;
#55149=CARTESIAN_POINT ( 'NONE',  ( 0.000000000000000000, -64.82615989628266107, -23.00000000000000000 ) ) ;
#55162=ORIENTED_EDGE ( 'NONE', *, *, #48777, .F. ) ;
#55191=DIRECTION ( 'NONE',  ( -0.000000000000000000, -0.000000000000000000, 1.000000000000000000 ) ) ;
#55202=CARTESIAN_POINT ( 'NONE',  ( -36.91746825000000598, -11.99521256947794789, -4.524999997268813523 ) ) ;
#55211=FACE_OUTER_BOUND ( 'NONE', #139325, .T. ) ;
#55213=CARTESIAN_POINT ( 'NONE',  ( -12.73749492396214578, -155.7167183371837496, -23.00000000000000000 ) ) ;
#55254=DIRECTION ( 'NONE',  ( -0.000000000000000000, -0.000000000000000000, 1.000000000000000000 ) ) ;
#55260=CARTESIAN_POINT ( 'NONE',  ( 28.90000000000004476, 0.000000000000000000, -49.67367017693150189 ) ) ;
#55284=ORIENTED_EDGE ( 'NONE', *, *, #156407, .T. ) ;
#55329=EDGE_CURVE ( 'NONE', #196237, #6179, #184580, .T. ) ;
#55405=DIRECTION ( 'NONE',  ( 1.000000000000000000, 0.000000000000000000, 0.000000000000000000 ) ) ;
#55411=CARTESIAN_POINT ( 'NONE',  ( -1.499966876285938833, -15.29519331188519615, -61.92990168432673670 ) ) ;
#55441=ORIENTED_EDGE ( 'NONE', *, *, #63444, .T. ) ;
#55444=DIRECTION ( 'NONE',  ( -1.000000000000000000, 0.000000000000000000, 0.000000000000000000 ) ) ;
#55448=CARTESIAN_POINT ( 'NONE',  ( 38.00000000000000000, 12.34694845685046616, -6.649999994537624914 ) ) ;
#55456=DIRECTION ( 'NONE',  ( 1.000000000000000000, 0.000000000000000000, 0.000000000000000000 ) ) ;
#55461=CARTESIAN_POINT ( 'NONE',  ( -11.94368209565404548, 9.822817408786974624, -59.71171441009364145 ) ) ;
#55466=VERTEX_POINT ( 'NONE', #123565 ) ;
#55485=CARTESIAN_POINT ( 'NONE',  ( -69.65682714487590488, -71.74905178543390605, -25.00000000000000000 ) ) ;
#55501=CARTESIAN_POINT ( 'NONE',  ( -36.91746825000000598, 2.428612866367529932E-14, -3.124999997268813168 ) ) ;
#55502=CARTESIAN_POINT ( 'NONE',  ( -0.4285070731208345807, -24.24152472029835792, -56.81472536503800796 ) ) ;
#55522=CARTESIAN_POINT ( 'NONE',  ( -26.94323156050993617, -28.89364864972289126, -18.52709669219113309 ) ) ;
#55523=ORIENTED_EDGE ( 'NONE', *, *, #26286, .F. ) ;
#55533=CARTESIAN_POINT ( 'NONE',  ( 11.49022483853025633, 12.06727048284061610, -61.36479237366228290 ) ) ;
#55534=ORIENTED_EDGE ( 'NONE', *, *, #44832, .T. ) ;
#55539=CARTESIAN_POINT ( 'NONE',  ( -1.313804288003784793, -8.349412516403770468, -64.09731636040746139 ) ) ;
#55550=CARTESIAN_POINT ( 'NONE',  ( 1.455685960264199608, 15.57403722060355022, -61.81495257977202584 ) ) ;
#55568=EDGE_CURVE ( 'NONE', #42510, #150779, #198615, .T. ) ;
#55633=CARTESIAN_POINT ( 'NONE',  ( -10.59477242850411649, -90.60836494048552936, -15.00000000000000178 ) ) ;
#55652=DIRECTION ( 'NONE',  ( 0.000000000000000000, 0.000000000000000000, 1.000000000000000000 ) ) ;
#55655=CARTESIAN_POINT ( 'NONE',  ( 0.1381572879930670350, 31.90000000000002700, -45.64921306006599622 ) ) ;
#55672=ORIENTED_EDGE ( 'NONE', *, *, #91752, .F. ) ;
#55706=EDGE_CURVE ( 'NONE', #28823, #146440, #104934, .T. ) ;
#55707=CARTESIAN_POINT ( 'NONE',  ( -10.41242334162750716, -12.21727042188736156, -59.44333992957475488 ) ) ;
#55741=ORIENTED_EDGE ( 'NONE', *, *, #60543, .T. ) ;
#55751=DIRECTION ( 'NONE',  ( 1.000000000000000000, 0.000000000000000000, 3.469446951953612217E-15 ) ) ;
#55779=AXIS2_PLACEMENT_3D ( 'NONE', #92099, #135661, #136629 ) ;
#55782=FACE_OUTER_BOUND ( 'NONE', #69865, .T. ) ;
#55783=ORIENTED_EDGE ( 'NONE', *, *, #148801, .F. ) ;
#55819=DIRECTION ( 'NONE',  ( 0.000000000000000000, 0.000000000000000000, 1.000000000000000000 ) ) ;
#55856=CARTESIAN_POINT ( 'NONE',  ( 3.766062262543149401E-15, -39.95556452105413570, -3.249999994537626780 ) ) ;
#55859=CARTESIAN_POINT ( 'NONE',  ( -28.66795886109348501, -27.90106222674905112, -15.73198891958529622 ) ) ;
#55918=DIRECTION ( 'NONE',  ( -1.000000000000000000, 0.000000000000000000, 0.000000000000000000 ) ) ;
#55924=CIRCLE ( 'NONE', #168913, 39.19183588453087452 ) ;
#55934=ORIENTED_EDGE ( 'NONE', *, *, #192965, .T. ) ;
#55938=CARTESIAN_POINT ( 'NONE',  ( 1.500000000004064082, 7.599999999999568878, -62.20201607440122871 ) ) ;
#55941=EDGE_CURVE ( 'NONE', #111780, #115644, #191971, .T. ) ;
#55943=CARTESIAN_POINT ( 'NONE',  ( -21.23184647844206552, -181.1785498424364675, -15.00000000000000178 ) ) ;
#55947=CARTESIAN_POINT ( 'NONE',  ( -38.00000000000000711, 2.428612866367529932E-14, -6.000000000000000000 ) ) ;
#55964=EDGE_CURVE ( 'NONE', #57253, #138331, #3711, .T. ) ;
#55968=CARTESIAN_POINT ( 'NONE',  ( 22.81625015709509441, 31.40387420917330275, -7.324999997268812457 ) ) ;
#55973=CARTESIAN_POINT ( 'NONE',  ( 0.7822855905564412016, 16.49570789208851807, -59.22457827466391223 ) ) ;
#55977=CARTESIAN_POINT ( 'NONE',  ( 29.45353567398453265, -26.40584612579220547, -18.78685418917150685 ) ) ;
#55993=CARTESIAN_POINT ( 'NONE',  ( 5.630366384172311278, -47.63986359793406677, -22.87684677291067814 ) ) ;
#55997=EDGE_LOOP ( 'NONE', ( #119825, #193707, #29237, #30215 ) ) ;
#56003=CARTESIAN_POINT ( 'NONE',  ( -30.20036327792369235, -26.22857331006468229, -17.18026671435357500 ) ) ;
#56026=CARTESIAN_POINT ( 'NONE',  ( 3.556970738554033499E-15, -38.81732327939057825, -8.124999997268814056 ) ) ;
#56030=CARTESIAN_POINT ( 'NONE',  ( 4.538945330120077948, -4.119035683228635669, -64.52788751195758721 ) ) ;
#56062=CARTESIAN_POINT ( 'NONE',  ( -19.97888994334923041, -34.65319547504298470, 0.000000000000000000 ) ) ;
#56086=DIRECTION ( 'NONE',  ( 1.000000000000000000, 0.000000000000000000, 0.000000000000000000 ) ) ;
#56119=ADVANCED_FACE ( 'NONE', ( #24140 ), #48742, .F. ) ;
#56147=ORIENTED_EDGE ( 'NONE', *, *, #197557, .T. ) ;
#56163=ORIENTED_EDGE ( 'NONE', *, *, #86821, .F. ) ;
#56176=CYLINDRICAL_SURFACE ( 'NONE', #2294, 28.90000000000004476 ) ;
#56186=CARTESIAN_POINT ( 'NONE',  ( -14.92381850146897371, -15.21399023779380677, -56.46147852626893382 ) ) ;
#56191=CARTESIAN_POINT ( 'NONE',  ( -21.61432565731197997, -33.65169730710061913, -23.91085783830776634 ) ) ;
#56202=CARTESIAN_POINT ( 'NONE',  ( -11.40812507854754720, -35.11059874428192273, -2.224999997268813701 ) ) ;
#56239=VERTEX_POINT ( 'NONE', #111396 ) ;
#56297=AXIS2_PLACEMENT_3D ( 'NONE', #177875, #98997, #40343 ) ;
#56353=CARTESIAN_POINT ( 'NONE',  ( -13.70000000000001528, 1.443387660838688656E-13, -60.44446360152740283 ) ) ;
#56391=CARTESIAN_POINT ( 'NONE',  ( -16.11132338694247679, 14.61887724323077897, -56.15647863711519960 ) ) ;
#56411=CARTESIAN_POINT ( 'NONE',  ( -20.00963169948588316, -33.79917020545752848, -17.75419178524651898 ) ) ;
#56417=CARTESIAN_POINT ( 'NONE',  ( -1.322814319812971595, -14.46726734353923050, -62.26916108939696670 ) ) ;
#56438=CARTESIAN_POINT ( 'NONE',  ( 12.14277428280450444, -10.17741597220468108, -59.53979320017422339 ) ) ;
#56440=AXIS2_PLACEMENT_3D ( 'NONE', #23183, #69680, #114164 ) ;
#56451=CARTESIAN_POINT ( 'NONE',  ( 21.61432565731214339, -33.65169730710053386, -23.91085783830763489 ) ) ;
#56455=CARTESIAN_POINT ( 'NONE',  ( 30.74264578624799782, 22.33583958711400541, -4.549999994537627046 ) ) ;
#56467=CARTESIAN_POINT ( 'NONE',  ( -12.06828707866192119, 11.48863819084119342, -59.15275318406537508 ) ) ;
#56493=DIRECTION ( 'NONE',  ( 1.000000000000000000, -1.776356839400250465E-15, 0.000000000000000000 ) ) ;
#56501=CIRCLE ( 'NONE', #114483, 214.0437394197456911 ) ;
#56505=CARTESIAN_POINT ( 'NONE',  ( 11.40812507854755253, -35.11059874428192273, -6.524999997268813523 ) ) ;
#56506=DIRECTION ( 'NONE',  ( 1.000000000000000000, 1.776356839400250465E-15, 0.000000000000000000 ) ) ;
#56529=CARTESIAN_POINT ( 'NONE',  ( -26.72240360496086709, -29.37940146934014507, -20.20861161915233595 ) ) ;
#56540=ORIENTED_EDGE ( 'NONE', *, *, #35894, .F. ) ;
#56545=CARTESIAN_POINT ( 'NONE',  ( -1.490470117976196107, -7.405238625847243128, -64.28041130758168720 ) ) ;
#56667=CARTESIAN_POINT ( 'NONE',  ( -31.34482716061811303, -21.47441072263947248, -23.96158720469884074 ) ) ;
#56685=ORIENTED_EDGE ( 'NONE', *, *, #136297, .F. ) ;
#56706=DIRECTION ( 'NONE',  ( 0.000000000000000000, 0.000000000000000000, 1.000000000000000000 ) ) ;
#56719=AXIS2_PLACEMENT_3D ( 'NONE', #162890, #54712, #190237 ) ;
#56738=CARTESIAN_POINT ( 'NONE',  ( 17.41079204577542683, -36.66972510653776851, -18.74440029985508716 ) ) ;
#56776=VERTEX_POINT ( 'NONE', #73640 ) ;
#56797=ORIENTED_EDGE ( 'NONE', *, *, #630, .T. ) ;
#56852=CARTESIAN_POINT ( 'NONE',  ( 2.973862142520690366, -93.04182470242774627, -25.00000000000000000 ) ) ;
#56916=EDGE_LOOP ( 'NONE', ( #191296, #145144, #181510, #9977, #174148 ) ) ;
#56919=VERTEX_POINT ( 'NONE', #149469 ) ;
#56921=ORIENTED_EDGE ( 'NONE', *, *, #182692, .F. ) ;
#56924=AXIS2_PLACEMENT_3D ( 'NONE', #126630, #33644, #34635 ) ;
#56970=CARTESIAN_POINT ( 'NONE',  ( -27.86273085795036408, -28.69962071417357663, 0.000000000000000000 ) ) ;
#56978=CARTESIAN_POINT ( 'NONE',  ( 11.40812507854755253, -35.11059874428192273, -10.02499999726881441 ) ) ;
#56983=CARTESIAN_POINT ( 'NONE',  ( 1.221313414957698099E-14, -31.90000000000003411, -49.13275782002545355 ) ) ;
#57003=ORIENTED_EDGE ( 'NONE', *, *, #137018, .T. ) ;
#57024=AXIS2_PLACEMENT_3D ( 'NONE', #149860, #26532, #104351 ) ;
#57034=EDGE_LOOP ( 'NONE', ( #158185, #184469 ) ) ;
#57039=CARTESIAN_POINT ( 'NONE',  ( -11.40812507854755609, 35.11059874428196537, -9.024999997268814411 ) ) ;
#57043=CARTESIAN_POINT ( 'NONE',  ( 6.090539141055496763, -4.048154665053746548, -64.32606980895295123 ) ) ;
#57068=CYLINDRICAL_SURFACE ( 'NONE', #65576, 40.00000000000000000 ) ;
#57100=CARTESIAN_POINT ( 'NONE',  ( -21.23184647844206197, -181.1785498424364675, -25.00000000000000000 ) ) ;
#57163=ORIENTED_EDGE ( 'NONE', *, *, #158775, .F. ) ;
#57168=CIRCLE ( 'NONE', #108813, 4.000000000000000888 ) ;
#57185=CIRCLE ( 'NONE', #50663, 21.30000000000002913 ) ;
#57214=ORIENTED_EDGE ( 'NONE', *, *, #29165, .F. ) ;
#57217=CARTESIAN_POINT ( 'NONE',  ( -36.91746825000000598, -11.99521256947794789, -6.524999997268811747 ) ) ;
#57219=CIRCLE ( 'NONE', #50704, 24.30000000000003268 ) ;
#57253=VERTEX_POINT ( 'NONE', #87784 ) ;
#57275=CARTESIAN_POINT ( 'NONE',  ( 29.34370184275720206, -1.069973119863033784, -49.12095057784394925 ) ) ;
#57286=CARTESIAN_POINT ( 'NONE',  ( 4.999999999999999112, 5.000000000000000888, -18.00000000000000000 ) ) ;
#57309=AXIS2_PLACEMENT_3D ( 'NONE', #145004, #23679, #6485 ) ;
#57363=EDGE_CURVE ( 'NONE', #126933, #112813, #72616, .T. ) ;
#57406=CARTESIAN_POINT ( 'NONE',  ( -17.56366054824412259, 15.66972982126927150, -54.83331888096112294 ) ) ;
#57448=DIRECTION ( 'NONE',  ( 0.000000000000000000, -0.000000000000000000, -1.000000000000000000 ) ) ;
#57455=ORIENTED_EDGE ( 'NONE', *, *, #145117, .T. ) ;
#57459=CARTESIAN_POINT ( 'NONE',  ( 15.06137443927350361, 15.06137443927346098, -64.92279855667830191 ) ) ;
#57464=CARTESIAN_POINT ( 'NONE',  ( 11.74264578624799427, 36.14014761921585972, -10.34999999453762598 ) ) ;
#57476=CARTESIAN_POINT ( 'NONE',  ( -11.74387995961032516, 9.622336364422256594, -59.83536316257175258 ) ) ;
#57480=CIRCLE ( 'NONE', #34783, 216.0437394197456342 ) ;
#57481=ADVANCED_FACE ( 'NONE', ( #153438 ), #30749, .F. ) ;
#57489=DIRECTION ( 'NONE',  ( -0.000000000000000000, -0.000000000000000000, -1.000000000000000000 ) ) ;
#57495=DIRECTION ( 'NONE',  ( 1.000000000000000000, 6.391086490440868450E-16, 0.000000000000000000 ) ) ;
#57504=LINE ( 'NONE', #73671, #112969 ) ;
#57515=CARTESIAN_POINT ( 'NONE',  ( 11.40812507854755253, -35.11059874428192273, -2.524999997268813523 ) ) ;
#57530=ORIENTED_EDGE ( 'NONE', *, *, #14301, .F. ) ;
#57536=CARTESIAN_POINT ( 'NONE',  ( -31.90410663231274668, -24.66877891592858774, -17.57859634138819871 ) ) ;
#57537=ORIENTED_EDGE ( 'NONE', *, *, #85994, .T. ) ;
#57550=CARTESIAN_POINT ( 'NONE',  ( 23.87412888849588555, -1.051486528467125758, -54.54543624665771517 ) ) ;
#57562=CARTESIAN_POINT ( 'NONE',  ( -2.500000000000000000, -165.0000000000000000, 7.000000000000003553 ) ) ;
#57563=CARTESIAN_POINT ( 'NONE',  ( 6.100000000000006750, -2.167155344068307965E-14, -64.53213882399991519 ) ) ;
#57571=CARTESIAN_POINT ( 'NONE',  ( 0.000000000000000000, 0.000000000000000000, -25.00000000000000000 ) ) ;
#57649=FACE_OUTER_BOUND ( 'NONE', #135011, .T. ) ;
#57684=VERTEX_POINT ( 'NONE', #131057 ) ;
#57691=CARTESIAN_POINT ( 'NONE',  ( -3.573655867282028392E-15, 2.428612866367529932E-14, 0.000000000000000000 ) ) ;
#57736=CARTESIAN_POINT ( 'NONE',  ( -4.044156916725154538, -6.083257512445876536, -64.32761231701863380 ) ) ;
#57754=DIRECTION ( 'NONE',  ( -0.000000000000000000, -0.000000000000000000, -1.000000000000000000 ) ) ;
#57770=ORIENTED_EDGE ( 'NONE', *, *, #146444, .F. ) ;
#57794=ORIENTED_EDGE ( 'NONE', *, *, #195656, .F. ) ;
#57828=CARTESIAN_POINT ( 'NONE',  ( -36.91746825000000598, 2.428612866367529932E-14, -0.8749999972688132788 ) ) ;
#57914=ORIENTED_EDGE ( 'NONE', *, *, #12763, .F. ) ;
#57919=ORIENTED_EDGE ( 'NONE', *, *, #40254, .T. ) ;
#57947=FACE_OUTER_BOUND ( 'NONE', #63952, .T. ) ;
#57960=DIRECTION ( 'NONE',  ( -0.000000000000000000, -0.000000000000000000, 1.000000000000000000 ) ) ;
#57962=FACE_OUTER_BOUND ( 'NONE', #163386, .T. ) ;
#57976=CARTESIAN_POINT ( 'NONE',  ( -6.020228577223754586E-15, 39.95556452105416412, -8.500000000000001776 ) ) ;
#57981=CARTESIAN_POINT ( 'NONE',  ( 1.359207933839712945, 15.84156095272284226, -59.51388212957616730 ) ) ;
#57986=VECTOR ( 'NONE', #58805, 1000.000000000000000 ) ;
#57992=EDGE_CURVE ( 'NONE', #127301, #182346, #161402, .T. ) ;
#58003=CARTESIAN_POINT ( 'NONE',  ( 6.907351198297244643, -38.20768336774872154, -23.99027881317354272 ) ) ;
#58007=ORIENTED_EDGE ( 'NONE', *, *, #57992, .T. ) ;
#58033=CARTESIAN_POINT ( 'NONE',  ( -36.91746825000001309, -11.99521256947794789, -8.524999997268812635 ) ) ;
#58071=DIRECTION ( 'NONE',  ( 1.000000000000000000, 0.000000000000000000, 0.000000000000000000 ) ) ;
#58079=FACE_OUTER_BOUND ( 'NONE', #168917, .T. ) ;
#58110=DIRECTION ( 'NONE',  ( -0.000000000000000000, -0.000000000000000000, -1.000000000000000000 ) ) ;
#58169=EDGE_LOOP ( 'NONE', ( #121316, #48790, #158463, #157871 ) ) ;
#58205=CARTESIAN_POINT ( 'NONE',  ( -11.40812507854754720, -35.11059874428192273, -6.224999997268812812 ) ) ;
#58211=VERTEX_POINT ( 'NONE', #19897 ) ;
#58224=CARTESIAN_POINT ( 'NONE',  ( -11.80868324581545714, -11.80868324581525997, -64.92279855667830191 ) ) ;
#58231=EDGE_CURVE ( 'NONE', #41521, #69935, #129046, .T. ) ;
#58388=CARTESIAN_POINT ( 'NONE',  ( -17.63037570847463442, 16.23105266556533621, -54.49189616393496749 ) ) ;
#58407=DIRECTION ( 'NONE',  ( 0.000000000000000000, 0.000000000000000000, 1.000000000000000000 ) ) ;
#58434=ORIENTED_EDGE ( 'NONE', *, *, #76859, .F. ) ;
#58442=CARTESIAN_POINT ( 'NONE',  ( -22.81625015709510507, 31.40387420917330275, -1.424999997268813212 ) ) ;
#58455=CARTESIAN_POINT ( 'NONE',  ( -10.38518860439150693, 9.278585747845273346, -60.35672204601534219 ) ) ;
#58467=CARTESIAN_POINT ( 'NONE',  ( -22.10131684062750423, 1.340157125434860985, -58.31342218742628347 ) ) ;
#58473=CARTESIAN_POINT ( 'NONE',  ( -37.45873412500000654, 2.428612866367529932E-14, -11.43749999590322020 ) ) ;
#58494=CARTESIAN_POINT ( 'NONE',  ( 11.40812507854754365, 35.11059874428196537, -7.724999997268813701 ) ) ;
#58510=ORIENTED_EDGE ( 'NONE', *, *, #22985, .F. ) ;
#58516=CARTESIAN_POINT ( 'NONE',  ( -29.45353567398637651, -26.40584612579511870, -18.78685418918301409 ) ) ;
#58527=ORIENTED_EDGE ( 'NONE', *, *, #139743, .T. ) ;
#58531=CARTESIAN_POINT ( 'NONE',  ( -1.197302953328902797, -6.691186640346296066, -64.41832325557876970 ) ) ;
#58543=CARTESIAN_POINT ( 'NONE',  ( 7.214655873249300910, -1.452908486251167419, -64.31726809345072127 ) ) ;
#58626=EDGE_CURVE ( 'NONE', #142912, #105638, #89551, .T. ) ;
#58641=CARTESIAN_POINT ( 'NONE',  ( -4.991179326919329640, 3.920341815485290482, -62.46637012391574473 ) ) ;
#58706=CARTESIAN_POINT ( 'NONE',  ( -6.434671708797631950, -6.434671708797536027, -63.95112321872120731 ) ) ;
#58763=TOROIDAL_SURFACE ( 'NONE', #171777, 69.99999999999998579, 10.00000000000000000 ) ;
#58796=CARTESIAN_POINT ( 'NONE',  ( 0.000000000000000000, 0.000000000000000000, -25.00000000000000000 ) ) ;
#58799=VERTEX_POINT ( 'NONE', #70398 ) ;
#58801=CARTESIAN_POINT ( 'NONE',  ( -5.000000000000003553, 37.66961640367474473, -18.00000000000000355 ) ) ;
#58805=DIRECTION ( 'NONE',  ( -0.000000000000000000, -0.000000000000000000, 1.000000000000000000 ) ) ;
#58841=CARTESIAN_POINT ( 'NONE',  ( 22.73749492396215288, -155.7167183371838064, -25.00000000000000000 ) ) ;
#58859=ADVANCED_FACE ( 'NONE', ( #104722 ), #181578, .F. ) ;
#58891=ORIENTED_EDGE ( 'NONE', *, *, #101613, .F. ) ;
#58932=CARTESIAN_POINT ( 'NONE',  ( 15.57302527691884109, -1.455916144794709322, -59.63194581529845095 ) ) ;
#58934=CYLINDRICAL_SURFACE ( 'NONE', #187032, 1.500000000000001332 ) ;
#58942=DIRECTION ( 'NONE',  ( -0.000000000000000000, -0.000000000000000000, 1.000000000000000000 ) ) ;
#58951=CARTESIAN_POINT ( 'NONE',  ( 30.74264578624800137, -22.33583958711395212, -3.200000000000000178 ) ) ;
#58981=ORIENTED_EDGE ( 'NONE', *, *, #30897, .F. ) ;
#58993=EDGE_CURVE ( 'NONE', #40993, #142912, #170492, .T. ) ;
#59008=CARTESIAN_POINT ( 'NONE',  ( -22.81625015709509441, -31.40387420917324590, -10.32499999726881157 ) ) ;
#59012=CARTESIAN_POINT ( 'NONE',  ( 6.218318179416534974, -4.125676326126586524, -64.29800624995039016 ) ) ;
#59065=CARTESIAN_POINT ( 'NONE',  ( 0.000000000000000000, 0.000000000000000000, -15.00000000000000000 ) ) ;
#59082=DIRECTION ( 'NONE',  ( -1.000000000000000000, 0.000000000000000000, 0.000000000000000000 ) ) ;
#59098=TOROIDAL_SURFACE ( 'NONE', #78418, 69.99999999999998579, 10.00000000000000000 ) ;
#59153=AXIS2_PLACEMENT_3D ( 'NONE', #62057, #92398, #121751 ) ;
#59178=CARTESIAN_POINT ( 'NONE',  ( -36.91746825000000598, 11.99521256947798520, -8.724999997268813701 ) ) ;
#59188=CYLINDRICAL_SURFACE ( 'NONE', #36523, 1.499999999999997780 ) ;
#59196=CARTESIAN_POINT ( 'NONE',  ( 8.400629636141365708, -38.44252190851328521, -32.19688134020121595 ) ) ;
#59254=CARTESIAN_POINT ( 'NONE',  ( 31.90000000000003411, -9.916512055951908821E-14, -45.64921306006598201 ) ) ;
#59332=CARTESIAN_POINT ( 'NONE',  ( -11.30153831258470731, -188.0000000000000000, -15.00000000000000178 ) ) ;
#59369=DIRECTION ( 'NONE',  ( -0.000000000000000000, -0.000000000000000000, 1.000000000000000000 ) ) ;
#59403=LINE ( 'NONE', #179802, #79842 ) ;
#59419=VERTEX_POINT ( 'NONE', #179352 ) ;
#59425=CARTESIAN_POINT ( 'NONE',  ( 3.556970738554033499E-15, -38.81732327939057825, -4.624999997268814056 ) ) ;
#59476=CARTESIAN_POINT ( 'NONE',  ( 3.556970738554034288E-15, -38.81732327939057114, -8.624999997268814056 ) ) ;
#59480=CARTESIAN_POINT ( 'NONE',  ( 1.203566692396469184, 8.516350909510459033, -64.06484607254931518 ) ) ;
#59497=CARTESIAN_POINT ( 'NONE',  ( -28.71286925542075963, -27.61909494970944579, -16.96471949292295989 ) ) ;
#59540=AXIS2_PLACEMENT_3D ( 'NONE', #155384, #58407, #181761 ) ;
#59584=CARTESIAN_POINT ( 'NONE',  ( 22.55670631985092811, 22.55670631985084640, -49.13275782002545355 ) ) ;
#59594=ORIENTED_EDGE ( 'NONE', *, *, #65973, .T. ) ;
#59626=CARTESIAN_POINT ( 'NONE',  ( -6.863180944108042247, 5.169469635059288137, -62.01598399707661002 ) ) ;
#59630=CARTESIAN_POINT ( 'NONE',  ( -21.51070015259078616, 19.98452092126590429, -49.12424573582180898 ) ) ;
#59648=CARTESIAN_POINT ( 'NONE',  ( -22.80000000000002913, 2.457562174807778276E-13, -64.92279855667830191 ) ) ;
#59660=EDGE_CURVE ( 'NONE', #51296, #182074, #148000, .T. ) ;
#59676=DIRECTION ( 'NONE',  ( 1.000000000000000000, 0.000000000000000000, 0.000000000000000000 ) ) ;
#59721=( BOUNDED_CURVE ( )  B_SPLINE_CURVE ( 2, ( #38213, #99869, #70547, #193906, #131209, #173402, #97510, #2545, #172398, #141059, #53019 ),
 .UNSPECIFIED., .F., .T. ) 
 B_SPLINE_CURVE_WITH_KNOTS ( ( 3, 2, 2, 2, 2, 3 ),
 ( 0.000000000000000000, 0.02000000000000000042, 0.04000000000000000083, 0.05999999999999999778, 0.08000000000000000167, 0.1000000000000000194 ),
 .UNSPECIFIED. ) 
 CURVE ( )  GEOMETRIC_REPRESENTATION_ITEM ( )  RATIONAL_B_SPLINE_CURVE ( ( 1.000000000000000000, 0.9510565162951535312, 1.000000000000000000, 0.9510565162951535312, 1.000000000000000000, 0.9510565162951535312, 1.000000000000000000, 0.9510565162951535312, 1.000000000000000000, 0.9510565162951535312, 1.000000000000000000 ) ) 
 REPRESENTATION_ITEM ( '' )  );
#59724=CARTESIAN_POINT ( 'NONE',  ( -6.824450432131288657, 4.979424220691202940, -64.09785073354593976 ) ) ;
#59760=ORIENTED_EDGE ( 'NONE', *, *, #7317, .T. ) ;
#59792=VERTEX_POINT ( 'NONE', #102485 ) ;
#59883=ORIENTED_EDGE ( 'NONE', *, *, #193684, .T. ) ;
#59916=CARTESIAN_POINT ( 'NONE',  ( 19.70810511599106363, -36.80807878390139365, -19.26229262562157984 ) ) ;
#59921=CARTESIAN_POINT ( 'NONE',  ( -3.883669081187027139, -5.177897575765684657, -64.47298040648024653 ) ) ;
#59923=DIRECTION ( 'NONE',  ( 1.000000000000000000, 0.000000000000000000, 0.000000000000000000 ) ) ;
#59929=CIRCLE ( 'NONE', #85764, 7.999999999999998224 ) ;
#59937=ORIENTED_EDGE ( 'NONE', *, *, #170098, .F. ) ;
#59940=CARTESIAN_POINT ( 'NONE',  ( -11.74264578624799782, -36.14014761921581709, -5.599999999999999645 ) ) ;
#59994=ORIENTED_EDGE ( 'NONE', *, *, #68507, .T. ) ;
#60012=DIRECTION ( 'NONE',  ( 0.000000000000000000, 0.000000000000000000, 1.000000000000000000 ) ) ;
#60028=TOROIDAL_SURFACE ( 'NONE', #37515, 206.0437394197456911, 8.000000000000000000 ) ;
#60072=CARTESIAN_POINT ( 'NONE',  ( 0.000000000000000000, 0.000000000000000000, -61.34707691135562868 ) ) ;
#60075=DIRECTION ( 'NONE',  ( 0.000000000000000000, 0.000000000000000000, -1.000000000000000000 ) ) ;
#60085=CARTESIAN_POINT ( 'NONE',  ( -10.59477242850411649, -90.60836494048552936, 0.000000000000000000 ) ) ;
#60133=CARTESIAN_POINT ( 'NONE',  ( -11.22590306719490627, -43.10241010958068841, -21.31070173013197433 ) ) ;
#60149=CARTESIAN_POINT ( 'NONE',  ( -4.790240017743690792, -48.14548474357629715, -22.95279619250844760 ) ) ;
#60172=CARTESIAN_POINT ( 'NONE',  ( 36.91746824999999177, 2.880721459617395097E-14, -7.624999997268813168 ) ) ;
#60223=CIRCLE ( 'NONE', #8561, 31.90000000000003411 ) ;
#60318=AXIS2_PLACEMENT_3D ( 'NONE', #42477, #181984, #40470 ) ;
#60319=EDGE_CURVE ( 'NONE', #190734, #35769, #27937, .T. ) ;
#60353=VERTEX_POINT ( 'NONE', #14447 ) ;
#60382=CARTESIAN_POINT ( 'NONE',  ( 0.7842620108279171331, 13.90517634892589882, -60.35638352309626953 ) ) ;
#60395=CARTESIAN_POINT ( 'NONE',  ( 17.18269478283316332, -17.18269478283309226, -54.21489346206828230 ) ) ;
#60404=CARTESIAN_POINT ( 'NONE',  ( 0.5310895872712830812, 21.39321968400172125, -58.79437919268159618 ) ) ;
#60419=CARTESIAN_POINT ( 'NONE',  ( -11.40812507854754720, -35.11059874428192273, -4.724999997268812812 ) ) ;
#60426=DIRECTION ( 'NONE',  ( 1.000000000000000000, 0.000000000000000000, 0.000000000000000000 ) ) ;
#60431=CARTESIAN_POINT ( 'NONE',  ( 4.457937930945874427, 6.565741541539653170, -62.16217994089669929 ) ) ;
#60466=CARTESIAN_POINT ( 'NONE',  ( 11.40812507854755253, -35.11059874428192273, -8.524999997268814411 ) ) ;
#60514=CARTESIAN_POINT ( 'NONE',  ( 6.100000000000011191, -0.2000799437544851234, -64.53213882399991519 ) ) ;
#60534=CARTESIAN_POINT ( 'NONE',  ( 1.452748147864696193, 7.214060343420894306, -64.31738320500510042 ) ) ;
#60536=ORIENTED_EDGE ( 'NONE', *, *, #121441, .T. ) ;
#60543=EDGE_CURVE ( 'NONE', #84237, #117432, #131226, .T. ) ;
#60551=DIRECTION ( 'NONE',  ( -0.000000000000000000, -0.000000000000000000, -1.000000000000000000 ) ) ;
#60615=CARTESIAN_POINT ( 'NONE',  ( -22.04836444019715458, 20.09153389842209236, -48.54295043639820051 ) ) ;
#60635=CARTESIAN_POINT ( 'NONE',  ( 2.285367203649865752E-16, -78.65850330665435308, -23.00000000000000000 ) ) ;
#60655=LINE ( 'NONE', #47499, #123791 ) ;
#60708=B_SPLINE_CURVE_WITH_KNOTS ( 'NONE', 3,
 ( #132307, #104961, #72642, #88792, #118145, #58455, #179835, #163651, #182806, #117132, #119148, #103968, #9973, #86795, #57476, #55461, #193999, #166647, #134317, #150485, #41305, #56467, #181814, #196989 ),
 .UNSPECIFIED., .F., .F.,
 ( 4, 2, 2, 2, 2, 2, 2, 2, 2, 2, 2, 4 ),
 ( 2.787091051190863422E-07, 0.0003070612385125897443, 0.0006138437679200604239, 0.001227408826735005253, 0.001534191356142474739, 0.001840973885549944010, 0.002147756414957413280, 0.002454538944364882333, 0.003068104003179821741, 0.003681669061994760281, 0.004295234120809699255, 0.004908799179624637361 ),
 .UNSPECIFIED. ) ;
#60715=CARTESIAN_POINT ( 'NONE',  ( -3.503282210674363295, -48.86437366581481001, -25.00000000000000000 ) ) ;
#60722=ORIENTED_EDGE ( 'NONE', *, *, #166964, .F. ) ;
#60776=SPHERICAL_SURFACE ( 'NONE', #110757, 40.00000000000002132 ) ;
#60868=ORIENTED_EDGE ( 'NONE', *, *, #20458, .T. ) ;
#60870=CARTESIAN_POINT ( 'NONE',  ( -2.500000000000000000, -105.0000000000000000, 7.000000000000003553 ) ) ;
#60879=CARTESIAN_POINT ( 'NONE',  ( 16.61713888009428075, -0.5018587474792359782, -61.38171595447354179 ) ) ;
#60885=EDGE_CURVE ( 'NONE', #138940, #93910, #11773, .T. ) ;
#60892=DIRECTION ( 'NONE',  ( -0.000000000000000000, -0.000000000000000000, 1.000000000000000000 ) ) ;
#60904=CARTESIAN_POINT ( 'NONE',  ( 10.06251177737616054, -45.32665049860680995, -23.77652626631510913 ) ) ;
#60908=CARTESIAN_POINT ( 'NONE',  ( -0.8285391498303467106, -21.53159096656797544, -56.30101842015763935 ) ) ;
#60912=DIRECTION ( 'NONE',  ( 0.000000000000000000, 0.000000000000000000, 1.000000000000000000 ) ) ;
#60918=DIRECTION ( 'NONE',  ( -0.000000000000000000, -0.000000000000000000, -1.000000000000000000 ) ) ;
#60928=CARTESIAN_POINT ( 'NONE',  ( -30.74264578624800492, -22.33583958711396278, -5.800000000000000711 ) ) ;
#60954=CARTESIAN_POINT ( 'NONE',  ( 14.77336750280265498, -39.52550427972109048, -19.86057791183392141 ) ) ;
#60985=CARTESIAN_POINT ( 'NONE',  ( 11.40812507854755253, -35.11059874428192273, -10.02499999726881441 ) ) ;
#61043=CARTESIAN_POINT ( 'NONE',  ( 0.000000000000000000, -105.0000000000000000, 12.00000000000000355 ) ) ;
#61069=CARTESIAN_POINT ( 'NONE',  ( -20.35785670957392668, -20.51291524300857816, -52.65483682830183199 ) ) ;
#61106=ORIENTED_EDGE ( 'NONE', *, *, #188107, .F. ) ;
#61119=CARTESIAN_POINT ( 'NONE',  ( -22.64239272338085485, -30.05593529206066705, -19.14955533181695202 ) ) ;
#61163=AXIS2_PLACEMENT_3D ( 'NONE', #78764, #145409, #53405 ) ;
#61180=CARTESIAN_POINT ( 'NONE',  ( 6.004573588225570191, -47.77740467397576651, -24.84605846612342006 ) ) ;
#61182=CARTESIAN_POINT ( 'NONE',  ( -11.15262245511042671, -12.20012380450693890, -61.42526006663408111 ) ) ;
#61218=EDGE_CURVE ( 'NONE', #70166, #102970, #53729, .T. ) ;
#61221=ORIENTED_EDGE ( 'NONE', *, *, #198190, .T. ) ;
#61224=CARTESIAN_POINT ( 'NONE',  ( 9.687362902255726382, 9.687362902255699737, -62.58071313852362039 ) ) ;
#61265=CARTESIAN_POINT ( 'NONE',  ( -19.24578484527059175, -180.9428398739492252, -15.00000000000000178 ) ) ;
#61278=AXIS2_PLACEMENT_3D ( 'NONE', #127028, #32061, #48228 ) ;
#61288=CARTESIAN_POINT ( 'NONE',  ( 0.000000000000000000, -165.0000000000000000, 7.000000000000003553 ) ) ;
#61320=ADVANCED_FACE ( 'NONE', ( #18437 ), #153893, .F. ) ;
#61390=FACE_BOUND ( 'NONE', #194765, .T. ) ;
#61396=DIRECTION ( 'NONE',  ( 1.000000000000000000, 0.000000000000000000, 0.000000000000000000 ) ) ;
#61404=ORIENTED_EDGE ( 'NONE', *, *, #55706, .T. ) ;
#61412=CARTESIAN_POINT ( 'NONE',  ( -11.74264578624799782, -36.14014761921581709, -11.34999999453762776 ) ) ;
#61417=AXIS2_PLACEMENT_3D ( 'NONE', #182537, #195734, #42040 ) ;
#61425=CARTESIAN_POINT ( 'NONE',  ( 11.95151397458945119, -11.66585251704126414, -59.13370768023892055 ) ) ;
#61463=CARTESIAN_POINT ( 'NONE',  ( -5.000000000000000000, 6.123233995736766282E-16, -18.00000000000000000 ) ) ;
#61464=CARTESIAN_POINT ( 'NONE',  ( 0.9733081508015164474, 23.94578629589191010, -57.02598899500504359 ) ) ;
#61546=CARTESIAN_POINT ( 'NONE',  ( 20.73749492396215288, -155.7167183371838064, -25.00000000000000000 ) ) ;
#61585=DIRECTION ( 'NONE',  ( -1.000000000000000000, 0.000000000000000000, 0.000000000000000000 ) ) ;
#61608=CARTESIAN_POINT ( 'NONE',  ( 1.500000000000003553, 30.40000000000004476, -47.75060438757614634 ) ) ;
#61679=ORIENTED_EDGE ( 'NONE', *, *, #103959, .T. ) ;
#61699=CARTESIAN_POINT ( 'NONE',  ( -4.313351365237961588, 4.313351365237934942, -64.53213882399992940 ) ) ;
#61778=DIRECTION ( 'NONE',  ( -0.000000000000000000, -0.000000000000000000, -1.000000000000000000 ) ) ;
#61855=ORIENTED_EDGE ( 'NONE', *, *, #115279, .F. ) ;
#61858=EDGE_LOOP ( 'NONE', ( #114048, #41177, #106715, #61106 ) ) ;
#61887=CARTESIAN_POINT ( 'NONE',  ( -6.938893903907228378E-15, -22.80000000000002913, -64.92279855667830191 ) ) ;
#61904=CARTESIAN_POINT ( 'NONE',  ( -16.10093921903352765, 14.61899031675401694, -58.57166825620330286 ) ) ;
#61914=CARTESIAN_POINT ( 'NONE',  ( 38.00000000000000000, 12.34694845685046616, -4.900000000000000355 ) ) ;
#61915=CIRCLE ( 'NONE', #7070, 16.70000000000002061 ) ;
#61920=CYLINDRICAL_SURFACE ( 'NONE', #176413, 31.90000000000003411 ) ;
#61939=ORIENTED_EDGE ( 'NONE', *, *, #76696, .F. ) ;
#61941=CARTESIAN_POINT ( 'NONE',  ( 16.00769354339547590, -38.20109431700117852, -19.33483434993953409 ) ) ;
#61969=ORIENTED_EDGE ( 'NONE', *, *, #133785, .F. ) ;
#61973=ORIENTED_EDGE ( 'NONE', *, *, #43460, .F. ) ;
#62020=CARTESIAN_POINT ( 'NONE',  ( 24.30000000000003268, 0.000000000000000000, -54.21489346206828230 ) ) ;
#62029=CARTESIAN_POINT ( 'NONE',  ( -14.62203461105063873, -16.12203461105573865, -58.56003730381080175 ) ) ;
#62030=CARTESIAN_POINT ( 'NONE',  ( 0.8851752879063210511, 31.61510582211850107, -49.48913787633048855 ) ) ;
#62057=CARTESIAN_POINT ( 'NONE',  ( 0.000000000000000000, 0.000000000000000000, -61.34707691135562868 ) ) ;
#62059=CARTESIAN_POINT ( 'NONE',  ( 22.55670631985092456, -22.55670631985084995, -64.92279855667830191 ) ) ;
#62085=EDGE_CURVE ( 'NONE', #145515, #4644, #60223, .T. ) ;
#62110=CARTESIAN_POINT ( 'NONE',  ( -8.963443992378397951, -45.12205215322087781, -22.08927284594089002 ) ) ;
#62132=DIRECTION ( 'NONE',  ( 1.000000000000000000, 0.000000000000000000, 0.000000000000000000 ) ) ;
#62168=CARTESIAN_POINT ( 'NONE',  ( 8.106210103299311243, -39.71824525391687644, -25.55638568641750297 ) ) ;
#62170=CARTESIAN_POINT ( 'NONE',  ( -10.01072506788280414, -12.06228617636993050, -61.80095975838368361 ) ) ;
#62224=CARTESIAN_POINT ( 'NONE',  ( -30.74264578624800492, 22.33583958711400186, -2.200000000000000178 ) ) ;
#62242=CARTESIAN_POINT ( 'NONE',  ( 1.500000000000005329, 15.20000000000001883, -61.96904110198155280 ) ) ;
#62249=DIRECTION ( 'NONE',  ( 0.000000000000000000, -1.000000000000000000, 0.000000000000000000 ) ) ;
#62255=EDGE_CURVE ( 'NONE', #185826, #149684, #45550, .T. ) ;
#62360=AXIS2_PLACEMENT_3D ( 'NONE', #131048, #9724, #193745 ) ;
#62385=CARTESIAN_POINT ( 'NONE',  ( -20.15954667362742825, -22.18921734867095452, -48.35113245326059683 ) ) ;
#62396=CIRCLE ( 'NONE', #43092, 38.00000000000000000 ) ;
#62401=CARTESIAN_POINT ( 'NONE',  ( -36.91746825000001309, 11.99521256947798342, -1.224999997268813035 ) ) ;
#62414=CARTESIAN_POINT ( 'NONE',  ( 4.884302457959432076, 6.795175062723209258, -62.06722337258344169 ) ) ;
#62448=CARTESIAN_POINT ( 'NONE',  ( -26.46959431505279881, -27.26463967846491698, -11.49588912907431393 ) ) ;
#62449=CARTESIAN_POINT ( 'NONE',  ( -5.950531402560715689E-15, 38.81732327939063509, -9.624999997268815832 ) ) ;
#62451=DIRECTION ( 'NONE',  ( 1.000000000000000000, 0.000000000000000000, 0.000000000000000000 ) ) ;
#62461=CARTESIAN_POINT ( 'NONE',  ( -12.24387616833797843, 10.52174046232662619, -61.59812483265029925 ) ) ;
#62470=ORIENTED_EDGE ( 'NONE', *, *, #142804, .F. ) ;
#62476=CARTESIAN_POINT ( 'NONE',  ( -34.32499373855440439, -22.49325299168063452, -18.44817765300819445 ) ) ;
#62499=ADVANCED_FACE ( 'NONE', ( #18204 ), #66706, .F. ) ;
#62535=AXIS2_PLACEMENT_3D ( 'NONE', #12539, #180406, #193562 ) ;
#62577=EDGE_CURVE ( 'NONE', #58799, #11425, #15054, .T. ) ;
#62598=CARTESIAN_POINT ( 'NONE',  ( -193.3062444957834884, -155.7167183371838064, -25.00000000000000000 ) ) ;
#62604=CARTESIAN_POINT ( 'NONE',  ( -23.87412888849583936, 1.051486528467328041, -54.54543624665774360 ) ) ;
#62638=ORIENTED_EDGE ( 'NONE', *, *, #135320, .F. ) ;
#62642=CARTESIAN_POINT ( 'NONE',  ( -6.404810000729013630, 0.9277198534073001213, -62.44539631020982284 ) ) ;
#62698=CARTESIAN_POINT ( 'NONE',  ( -4.908066780550751851, -48.27782543269305648, -24.94981842180952825 ) ) ;
#62703=DIRECTION ( 'NONE',  ( 1.000000000000000000, 0.000000000000000000, 0.000000000000000000 ) ) ;
#62705=VECTOR ( 'NONE', #34208, 1000.000000000000000 ) ;
#62740=CARTESIAN_POINT ( 'NONE',  ( 0.000000000000000000, 0.000000000000000000, -59.13370768023891344 ) ) ;
#62803=DIRECTION ( 'NONE',  ( 0.000000000000000000, 0.000000000000000000, -1.000000000000000000 ) ) ;
#62820=CIRCLE ( 'NONE', #175852, 38.00000000000000000 ) ;
#62849=EDGE_CURVE ( 'NONE', #173655, #193677, #82860, .T. ) ;
#62858=DIRECTION ( 'NONE',  ( 0.000000000000000000, 1.000000000000000000, 0.000000000000000000 ) ) ;
#62869=VECTOR ( 'NONE', #175537, 1000.000000000000000 ) ;
#62892=DIRECTION ( 'NONE',  ( 0.000000000000000000, 0.000000000000000000, 1.000000000000000000 ) ) ;
#62905=CARTESIAN_POINT ( 'NONE',  ( -17.18269478283316332, 17.18269478283309226, -56.77278709839600879 ) ) ;
#62925=DIRECTION ( 'NONE',  ( -0.000000000000000000, -0.000000000000000000, -1.000000000000000000 ) ) ;
#62939=CARTESIAN_POINT ( 'NONE',  ( 20.37447694478314730, -32.07477979233135557, -24.11443027216501278 ) ) ;
#62964=AXIS2_PLACEMENT_3D ( 'NONE', #49087, #112726, #173429 ) ;
#62967=VERTEX_POINT ( 'NONE', #129327 ) ;
#63000=VECTOR ( 'NONE', #51444, 1000.000000000000000 ) ;
#63008=DIRECTION ( 'NONE',  ( 0.000000000000000000, 0.000000000000000000, -1.000000000000000000 ) ) ;
#63011=CARTESIAN_POINT ( 'NONE',  ( 8.516083024820106928, -1.203758653825250269, -62.01440738234568073 ) ) ;
#63055=CARTESIAN_POINT ( 'NONE',  ( 9.687362902255724606, 9.687362902255701513, -60.44446360152740993 ) ) ;
#63098=ORIENTED_EDGE ( 'NONE', *, *, #95584, .F. ) ;
#63110=CARTESIAN_POINT ( 'NONE',  ( -19.25015247713983868, -32.77362114220466083, -25.12817986194701803 ) ) ;
#63132=CARTESIAN_POINT ( 'NONE',  ( 20.43538597629128262, -20.43538597629122222, -49.67367017693150189 ) ) ;
#63135=CARTESIAN_POINT ( 'NONE',  ( 4.175862767829956468, 6.297097159419585033, -64.28037419727766633 ) ) ;
#63140=CARTESIAN_POINT ( 'NONE',  ( 22.99604614807110181, -21.49604614807104142, -49.67998909148434450 ) ) ;
#63159=CARTESIAN_POINT ( 'NONE',  ( -36.91746825000000598, 2.428612866367529932E-14, -4.624999997268814056 ) ) ;
#63169=CARTESIAN_POINT ( 'NONE',  ( 26.41049836824324260, -29.67629096701676161, -20.30943395415963693 ) ) ;
#63188=EDGE_LOOP ( 'NONE', ( #25422, #9251, #31653, #170640 ) ) ;
#63203=VECTOR ( 'NONE', #14890, 1000.000000000000000 ) ;
#63228=CARTESIAN_POINT ( 'NONE',  ( -23.48529157249600985, 32.32473071737754111, -2.299999999999998934 ) ) ;
#63287=VERTEX_POINT ( 'NONE', #98990 ) ;
#63306=EDGE_CURVE ( 'NONE', #133509, #191474, #57219, .T. ) ;
#63320=B_SPLINE_CURVE_WITH_KNOTS ( 'NONE', 3,
 ( #158459, #84592, #53269, #52271, #51284, #114947, #162448, #7759, #69442, #177642, #39110, #146272, #100766, #85604, #175629, #19948, #132115, #82595, #8780, #143275, #144277, #113929, #40099, #27962 ),
 .UNSPECIFIED., .F., .F.,
 ( 4, 2, 2, 2, 2, 2, 2, 2, 2, 2, 2, 4 ),
 ( 2.784816138770050137E-07, 0.0003261688173017064543, 0.0006520591529895358339, 0.0009779494886773747002, 0.001303839824365213458, 0.001955620495740909189, 0.002607401167116605353, 0.003259181838492301083, 0.003910962509867992910, 0.004562743181243684304, 0.004888633516931526098, 0.005214523852619367891 ),
 .UNSPECIFIED. ) ;
#63335=B_SPLINE_CURVE_WITH_KNOTS ( 'NONE', 3,
 ( #159851, #116347, #177047, #67842, #114335, #194210, #133516, #8170, #147699, #52672, #146675, #193200, #115357, #54673, #178036, #162852 ),
 .UNSPECIFIED., .F., .F.,
 ( 4, 2, 2, 2, 2, 2, 2, 4 ),
 ( 0.02152764489805616965, 0.02408704820948082137, 0.02664645152090547309, 0.03176525814375479040, 0.03432466145517944905, 0.03560436311089177491, 0.03688406476660410077, 0.04200287138945340421 ),
 .UNSPECIFIED. ) ;
#63394=CARTESIAN_POINT ( 'NONE',  ( -22.48049813892993143, -22.63291450077185019, -45.64921306006597490 ) ) ;
#63411=CARTESIAN_POINT ( 'NONE',  ( -11.40812507854754720, -35.11059874428192273, -8.724999997268813701 ) ) ;
#63444=EDGE_CURVE ( 'NONE', #188934, #102970, #149511, .T. ) ;
#63462=CARTESIAN_POINT ( 'NONE',  ( 11.40812507854755253, -35.11059874428192273, -6.524999997268813523 ) ) ;
#63463=CARTESIAN_POINT ( 'NONE',  ( 1.227931366032057224E-14, 24.30000000000003268, -56.77278709839600879 ) ) ;
#63471=CARTESIAN_POINT ( 'NONE',  ( 13.29753078558972668, -35.33598341332321269, -29.59763579011271517 ) ) ;
#63478=ORIENTED_EDGE ( 'NONE', *, *, #15614, .F. ) ;
#63485=EDGE_LOOP ( 'NONE', ( #181791, #118149, #177869, #29107 ) ) ;
#63532=ORIENTED_EDGE ( 'NONE', *, *, #55093, .T. ) ;
#63591=CARTESIAN_POINT ( 'NONE',  ( 1.197484662147158874, 6.691433960895806443, -62.38716993895737062 ) ) ;
#63617=ADVANCED_FACE ( 'NONE', ( #26185 ), #118184, .F. ) ;
#63665=CARTESIAN_POINT ( 'NONE',  ( 23.94686256013573100, -0.9720251121415568463, -57.02522261278120652 ) ) ;
#63682=CIRCLE ( 'NONE', #86347, 9.100000000000001421 ) ;
#63707=CARTESIAN_POINT ( 'NONE',  ( -0.6194686979411263561, -31.77050690183225257, -45.83912112027729080 ) ) ;
#63738=EDGE_CURVE ( 'NONE', #42359, #93735, #27984, .T. ) ;
#63751=CARTESIAN_POINT ( 'NONE',  ( -0.6707077324887361636, -8.945340038113741343, -61.92615459704094860 ) ) ;
#63816=FACE_OUTER_BOUND ( 'NONE', #142298, .T. ) ;
#63823=CIRCLE ( 'NONE', #2474, 8.000000000000001776 ) ;
#63865=ORIENTED_EDGE ( 'NONE', *, *, #146334, .T. ) ;
#63905=CARTESIAN_POINT ( 'NONE',  ( -3.573655867282028392E-15, 2.428612866367529932E-14, -15.00000000000000000 ) ) ;
#63909=DIRECTION ( 'NONE',  ( -0.000000000000000000, -0.000000000000000000, -1.000000000000000000 ) ) ;
#63914=DIRECTION ( 'NONE',  ( 1.000000000000000000, 0.000000000000000000, 0.000000000000000000 ) ) ;
#63921=EDGE_LOOP ( 'NONE', ( #44492, #190801, #79691, #108555 ) ) ;
#63938=VECTOR ( 'NONE', #65527, 1000.000000000000000 ) ;
#63948=CARTESIAN_POINT ( 'NONE',  ( 21.74014569711068390, -31.09693755439586837, -22.87366378656934174 ) ) ;
#63952=EDGE_LOOP ( 'NONE', ( #147004, #155418, #131303, #166628, #27126, #61404 ) ) ;
#64059=CARTESIAN_POINT ( 'NONE',  ( 9.622336364422297450, 11.74387995961029141, -59.83536316257176679 ) ) ;
#64061=CARTESIAN_POINT ( 'NONE',  ( 14.67621740152110377, 15.70878279763964258, -56.33456566391306808 ) ) ;
#64113=VERTEX_POINT ( 'NONE', #157218 ) ;
#64115=CARTESIAN_POINT ( 'NONE',  ( -24.94166821950383195, -28.00113106727059176, -18.51304999530125173 ) ) ;
#64155=CARTESIAN_POINT ( 'NONE',  ( 0.000000000000000000, -165.0000000000000000, -23.00000000000000000 ) ) ;
#64161=ORIENTED_EDGE ( 'NONE', *, *, #24639, .T. ) ;
#64164=CARTESIAN_POINT ( 'NONE',  ( -29.86685920354755197, -21.69954338932560134, -6.424999997268812990 ) ) ;
#64174=CARTESIAN_POINT ( 'NONE',  ( 27.53771902582990450, -28.32105632907330062, -18.50180672658675363 ) ) ;
#64192=ORIENTED_EDGE ( 'NONE', *, *, #37197, .F. ) ;
#64210=ADVANCED_FACE ( 'NONE', ( #186586 ), #42345, .T. ) ;
#64219=VERTEX_POINT ( 'NONE', #43331 ) ;
#64226=CARTESIAN_POINT ( 'NONE',  ( -5.950531402560715689E-15, 38.81732327939063509, -9.624999997268815832 ) ) ;
#64234=DIRECTION ( 'NONE',  ( 6.391086490440868450E-16, -1.000000000000000000, 0.000000000000000000 ) ) ;
#64339=ORIENTED_EDGE ( 'NONE', *, *, #15073, .F. ) ;
#64367=CARTESIAN_POINT ( 'NONE',  ( 38.00000000000000000, -12.34694845685040754, -5.099999999999999645 ) ) ;
#64385=CARTESIAN_POINT ( 'NONE',  ( 1.500000000000020872, 22.80000000000002913, -55.36297086913598520 ) ) ;
#64394=CYLINDRICAL_SURFACE ( 'NONE', #146876, 6.100000000000006750 ) ;
#64404=FACE_OUTER_BOUND ( 'NONE', #125769, .T. ) ;
#64419=CARTESIAN_POINT ( 'NONE',  ( 6.125853549498594397, 6.687054376293244395, -61.90253133708614541 ) ) ;
#64442=DIRECTION ( 'NONE',  ( -0.000000000000000000, -0.000000000000000000, 1.000000000000000000 ) ) ;
#64456=CARTESIAN_POINT ( 'NONE',  ( -36.91746825000000598, 2.428612866367529932E-14, -5.124999997268813168 ) ) ;
#64458=CARTESIAN_POINT ( 'NONE',  ( -22.97168310438084760, 21.16989542479035080, -49.98402367076293018 ) ) ;
#64467=CARTESIAN_POINT ( 'NONE',  ( -10.00917710959074824, 9.438666190699219527, -62.55979675456845257 ) ) ;
#64480=CARTESIAN_POINT ( 'NONE',  ( -38.00000000000000711, 2.428612866367529932E-14, -11.74999999453762634 ) ) ;
#64481=ORIENTED_EDGE ( 'NONE', *, *, #121810, .T. ) ;
#64604=VECTOR ( 'NONE', #183526, 1000.000000000000000 ) ;
#64610=DIRECTION ( 'NONE',  ( -0.000000000000000000, -0.000000000000000000, 1.000000000000000000 ) ) ;
#64646=CARTESIAN_POINT ( 'NONE',  ( 32.12256032297300834, -23.75458735917137787, -22.83990191704117478 ) ) ;
#64659=CARTESIAN_POINT ( 'NONE',  ( -1.097581692000294984, -31.42649584489976533, -49.72218688481378734 ) ) ;
#64679=ORIENTED_EDGE ( 'NONE', *, *, #115279, .T. ) ;
#64735=CARTESIAN_POINT ( 'NONE',  ( 11.74264578624800315, -36.14014761921581709, -9.149999994537626691 ) ) ;
#64745=FACE_OUTER_BOUND ( 'NONE', #147587, .T. ) ;
#64769=CARTESIAN_POINT ( 'NONE',  ( -16.49801837613219035, -34.15639402546915449, -27.41207208920364025 ) ) ;
#64776=ADVANCED_FACE ( 'NONE', ( #52015 ), #114684, .F. ) ;
#64809=CARTESIAN_POINT ( 'NONE',  ( -8.231229499106921921, -38.47007264976929974, -32.24440875978790189 ) ) ;
#64868=CARTESIAN_POINT ( 'NONE',  ( 13.70000000000001528, -0.2066332630087097111, -62.58071313852360618 ) ) ;
#64870=EDGE_CURVE ( 'NONE', #11421, #159131, #96514, .T. ) ;
#64890=DIRECTION ( 'NONE',  ( -0.000000000000000000, -0.000000000000000000, 1.000000000000000000 ) ) ;
#64891=CARTESIAN_POINT ( 'NONE',  ( -69.65682714487590488, -71.74905178543390605, 0.000000000000000000 ) ) ;
#64902=FACE_OUTER_BOUND ( 'NONE', #184144, .T. ) ;
#64908=ORIENTED_EDGE ( 'NONE', *, *, #35894, .T. ) ;
#64929=B_SPLINE_CURVE_WITH_KNOTS ( 'NONE', 3,
 ( #63132, #171321, #188484, #91467, #137994, #16644, #48971, #153155, #14656, #2456, #79299, #76316, #1454, #106661, #77311, #184505, #17639, #124811, #457, #107640, #95456, #31814 ),
 .UNSPECIFIED., .F., .F.,
 ( 4, 2, 2, 2, 2, 2, 2, 2, 2, 2, 4 ),
 ( 2.775519118949223281E-07, 0.0003140540122564098344, 0.0006278304726009247688, 0.0009416069329454397575, 0.001255383393289954746, 0.001882936313978984724, 0.002510489234668014484, 0.003138042155357044245, 0.003765595076046074439, 0.004393147996735103332, 0.005020700917424133526 ),
 .UNSPECIFIED. ) ;
#64935=CARTESIAN_POINT ( 'NONE',  ( 19.65168359646968099, -34.19331532915641958, -17.88087567707446013 ) ) ;
#64960=EDGE_LOOP ( 'NONE', ( #75055, #126741, #67893, #123820 ) ) ;
#65019=CARTESIAN_POINT ( 'NONE',  ( -4.024989859040965179, -4.710833808339871531, -62.49156203976952639 ) ) ;
#65046=CARTESIAN_POINT ( 'NONE',  ( 0.000000000000000000, 0.000000000000000000, -64.92279855667830191 ) ) ;
#65082=ORIENTED_EDGE ( 'NONE', *, *, #87886, .T. ) ;
#65098=CARTESIAN_POINT ( 'NONE',  ( -29.30938409335406547, -24.40035533028687453, -16.80062434859987874 ) ) ;
#65127=LINE ( 'NONE', #3450, #146927 ) ;
#65146=CARTESIAN_POINT ( 'NONE',  ( -36.91746825000001309, 11.99521256947798342, -0.7249999972688133676 ) ) ;
#65156=CARTESIAN_POINT ( 'NONE',  ( 24.59647911868938763, -31.70815657101694995, -17.34206816074872037 ) ) ;
#65195=CARTESIAN_POINT ( 'NONE',  ( 0.000000000000000000, 0.000000000000000000, -64.92279855667830191 ) ) ;
#65207=CARTESIAN_POINT ( 'NONE',  ( 22.81625015709509441, 31.40387420917330275, -3.324999997268812901 ) ) ;
#65242=CARTESIAN_POINT ( 'NONE',  ( 37.99999999999999289, 2.893978650043524126E-14, -1.000000000000000000 ) ) ;
#65264=DIRECTION ( 'NONE',  ( 1.000000000000000000, 0.000000000000000000, 0.000000000000000000 ) ) ;
#65273=ORIENTED_EDGE ( 'NONE', *, *, #88864, .F. ) ;
#65351=CARTESIAN_POINT ( 'NONE',  ( -23.48529157249599919, -32.32473071737749848, -5.700000000000000178 ) ) ;
#65365=ADVANCED_FACE ( 'NONE', ( #81336 ), #127850, .F. ) ;
#65392=CARTESIAN_POINT ( 'NONE',  ( 11.40812507854754365, 35.11059874428196537, -7.724999997268813701 ) ) ;
#65426=DIRECTION ( 'NONE',  ( 0.000000000000000000, 0.000000000000000000, 1.000000000000000000 ) ) ;
#65436=LINE ( 'NONE', #127097, #138282 ) ;
#65439=CARTESIAN_POINT ( 'NONE',  ( 36.91746824999999177, 2.880721459617395097E-14, -4.124999997268813168 ) ) ;
#65447=CARTESIAN_POINT ( 'NONE',  ( 8.204442743001546745, -36.48291145135366520, -31.77125895174628312 ) ) ;
#65509=ORIENTED_EDGE ( 'NONE', *, *, #78263, .F. ) ;
#65527=DIRECTION ( 'NONE',  ( -0.000000000000000000, -0.000000000000000000, 1.000000000000000000 ) ) ;
#65576=AXIS2_PLACEMENT_3D ( 'NONE', #10566, #189848, #72230 ) ;
#65595=CARTESIAN_POINT ( 'NONE',  ( -22.10945809693575370, 1.344113590474837361, -55.87741762761909570 ) ) ;
#65608=CARTESIAN_POINT ( 'NONE',  ( 37.99999999999999289, 2.893978650043524126E-14, -1.000000000000000000 ) ) ;
#65627=CARTESIAN_POINT ( 'NONE',  ( 30.74264578624799782, 22.33583958711400541, -6.549999994537627046 ) ) ;
#65640=CARTESIAN_POINT ( 'NONE',  ( 24.30000000000003268, -0.1103568551765998634, -56.77278709839600168 ) ) ;
#65642=CARTESIAN_POINT ( 'NONE',  ( -1.502453648625268645, -30.26186088262145901, -51.11561252063850702 ) ) ;
#65695=CARTESIAN_POINT ( 'NONE',  ( -15.53529872673524004, -37.10890965030864663, -23.64498726423861186 ) ) ;
#65696=ORIENTED_EDGE ( 'NONE', *, *, #98431, .F. ) ;
#65727=CARTESIAN_POINT ( 'NONE',  ( -16.09882439466100124, 1.216645939406925780, -61.59766612755959869 ) ) ;
#65790=CARTESIAN_POINT ( 'NONE',  ( -4.521720347981119659, -38.96825017273092584, -33.00000000000000711 ) ) ;
#65844=FACE_OUTER_BOUND ( 'NONE', #135665, .T. ) ;
#65853=CARTESIAN_POINT ( 'NONE',  ( 15.38891197842629133, -1.491051326732930171, -61.89130710690760395 ) ) ;
#65871=DIRECTION ( 'NONE',  ( 1.000000000000000000, 0.000000000000000000, 0.000000000000000000 ) ) ;
#65882=CARTESIAN_POINT ( 'NONE',  ( 17.57848473335091555, -16.49314274028410310, -56.92152151716637576 ) ) ;
#65887=CARTESIAN_POINT ( 'NONE',  ( -15.57302527691882688, 1.455916144794820566, -59.63194581529847937 ) ) ;
#65893=ORIENTED_EDGE ( 'NONE', *, *, #28831, .T. ) ;
#65903=VECTOR ( 'NONE', #151948, 1000.000000000000000 ) ;
#65922=CARTESIAN_POINT ( 'NONE',  ( 25.08997344983162137, -28.19247641866554233, -20.54396225645222884 ) ) ;
#65948=ORIENTED_EDGE ( 'NONE', *, *, #136692, .F. ) ;
#65950=FACE_OUTER_BOUND ( 'NONE', #52283, .T. ) ;
#65965=AXIS2_PLACEMENT_3D ( 'NONE', #128016, #51191, #131014 ) ;
#65973=EDGE_CURVE ( 'NONE', #182543, #126159, #131372, .T. ) ;
#65985=DIRECTION ( 'NONE',  ( -1.000000000000000000, 6.391086490440866478E-16, 0.000000000000000000 ) ) ;
#65991=CARTESIAN_POINT ( 'NONE',  ( 6.854124442542001816, -1.305043071815303435, -62.35408385982738366 ) ) ;
#66074=ORIENTED_EDGE ( 'NONE', *, *, #64870, .F. ) ;
#66107=DIRECTION ( 'NONE',  ( -1.000000000000000000, -1.953992523340275511E-14, 0.000000000000000000 ) ) ;
#66112=EDGE_CURVE ( 'NONE', #86619, #66459, #35092, .T. ) ;
#66138=CARTESIAN_POINT ( 'NONE',  ( -36.91746825000000598, 2.428612866367529932E-14, -2.624999997268813168 ) ) ;
#66148=CARTESIAN_POINT ( 'NONE',  ( 24.90102501248377109, -31.06609936492516866, -21.12314233236756778 ) ) ;
#66159=AXIS2_PLACEMENT_3D ( 'NONE', #187947, #15101, #61585 ) ;
#66168=VERTEX_POINT ( 'NONE', #51539 ) ;
#66175=DIRECTION ( 'NONE',  ( 1.000000000000000000, 0.000000000000000000, 0.000000000000000000 ) ) ;
#66200=CARTESIAN_POINT ( 'NONE',  ( -11.40812507854755609, 35.11059874428196537, -9.524999997268816188 ) ) ;
#66202=CIRCLE ( 'NONE', #192226, 9.100000000000001421 ) ;
#66238=CARTESIAN_POINT ( 'NONE',  ( 29.02171288343477329, -0.6023940538448767645, -52.52077797743539378 ) ) ;
#66349=CARTESIAN_POINT ( 'NONE',  ( 20.24680444626657305, 22.34286686445877734, -48.12863666802713425 ) ) ;
#66351=CIRCLE ( 'NONE', #4999, 13.70000000000001528 ) ;
#66355=FACE_OUTER_BOUND ( 'NONE', #37582, .T. ) ;
#66362=EDGE_CURVE ( 'NONE', #166806, #45388, #52527, .T. ) ;
#66366=CARTESIAN_POINT ( 'NONE',  ( 1.469609370623580213, 22.44847579118772529, -55.62606073046919875 ) ) ;
#66369=DIRECTION ( 'NONE',  ( 1.000000000000000000, 0.000000000000000000, 0.000000000000000000 ) ) ;
#66389=CARTESIAN_POINT ( 'NONE',  ( -36.91746825000001309, -11.99521256947794789, -9.024999997268812635 ) ) ;
#66436=CARTESIAN_POINT ( 'NONE',  ( -22.81625015709510507, 31.40387420917330275, -1.424999997268813212 ) ) ;
#66437=CARTESIAN_POINT ( 'NONE',  ( -21.26972126690566611, 19.99598863510428970, -52.34638024103106346 ) ) ;
#66459=VERTEX_POINT ( 'NONE', #195061 ) ;
#66471=ORIENTED_EDGE ( 'NONE', *, *, #175399, .T. ) ;
#66563=LINE ( 'NONE', #23064, #108167 ) ;
#66603=CARTESIAN_POINT ( 'NONE',  ( -29.12650189376887511, 0.8004727011106961276, -52.40478149256038876 ) ) ;
#66616=ORIENTED_EDGE ( 'NONE', *, *, #97418, .T. ) ;
#66619=CARTESIAN_POINT ( 'NONE',  ( 28.30127546286013285, -27.84967942650701644, -20.15398247455537373 ) ) ;
#66621=CARTESIAN_POINT ( 'NONE',  ( -30.74264578624800492, -22.33583958711396278, -3.549999994537626602 ) ) ;
#66635=CARTESIAN_POINT ( 'NONE',  ( 24.75282386541786650, -28.51018972888594050, -20.68147073028488947 ) ) ;
#66648=CARTESIAN_POINT ( 'NONE',  ( -20.00287982954261423, -21.32739072855598650, -49.27013238145816842 ) ) ;
#66651=AXIS2_PLACEMENT_3D ( 'NONE', #136665, #185158, #92134 ) ;
#66672=CARTESIAN_POINT ( 'NONE',  ( -22.81625015709510507, 31.40387420917330275, -1.424999997268813212 ) ) ;
#66680=CARTESIAN_POINT ( 'NONE',  ( -1.495846735942510941, -30.59399807301415208, -47.49088840515941712 ) ) ;
#66686=CARTESIAN_POINT ( 'NONE',  ( -3.503282210674334873, -48.86437366581479580, -35.00000000000000000 ) ) ;
#66691=CARTESIAN_POINT ( 'NONE',  ( -18.08554851550293208, -38.44972689945520017, -20.08432885666762502 ) ) ;
#66703=CARTESIAN_POINT ( 'NONE',  ( 9.279464826303303937, 10.38198520235567024, -62.49863477660405664 ) ) ;
#66704=ORIENTED_EDGE ( 'NONE', *, *, #192980, .F. ) ;
#66706=CONICAL_SURFACE ( 'NONE', #179762, 2.500000000000000000, 1.029744258676656976 ) ;
#66720=CARTESIAN_POINT ( 'NONE',  ( 37.99999999999999289, 2.893978650043524126E-14, -1.000000000000000000 ) ) ;
#66747=DIRECTION ( 'NONE',  ( -1.000000000000000000, 0.000000000000000000, 0.000000000000000000 ) ) ;
#66759=CARTESIAN_POINT ( 'NONE',  ( -11.45643923738959735, 5.000000000000007105, -15.00000000000000000 ) ) ;
#66820=CARTESIAN_POINT ( 'NONE',  ( -15.73785899003303790, -17.57910283142216201, -57.30050143854533218 ) ) ;
#66842=DIRECTION ( 'NONE',  ( 1.000000000000000000, 0.000000000000000000, 0.000000000000000000 ) ) ;
#66852=CARTESIAN_POINT ( 'NONE',  ( 0.9809564218223714160, 23.93924616269290340, -54.49512787944463099 ) ) ;
#66869=DIRECTION ( 'NONE',  ( 1.000000000000000000, 0.000000000000000000, 0.000000000000000000 ) ) ;
#66873=DIRECTION ( 'NONE',  ( 1.000000000000000000, 0.000000000000000000, 0.000000000000000000 ) ) ;
#66896=CARTESIAN_POINT ( 'NONE',  ( 11.74264578624800315, -36.14014761921581709, -9.400000000000000355 ) ) ;
#66915=( LENGTH_UNIT ( ) NAMED_UNIT ( * ) SI_UNIT ( .MILLI., .METRE. ) );
#66919=CARTESIAN_POINT ( 'NONE',  ( 26.43919995774724185, -26.89423752947832114, -20.34026575423448691 ) ) ;
#66964=AXIS2_PLACEMENT_3D ( 'NONE', #17397, #127545, #123557 ) ;
#67086=ORIENTED_EDGE ( 'NONE', *, *, #102940, .T. ) ;
#67088=CARTESIAN_POINT ( 'NONE',  ( -29.33118895280791349, -23.95254016166466116, -21.73655181065874942 ) ) ;
#67105=DIRECTION ( 'NONE',  ( 1.000000000000000000, 0.000000000000000000, 0.000000000000000000 ) ) ;
#67111=CARTESIAN_POINT ( 'NONE',  ( -29.64248797448946249, 1.297617798568585501, -48.74145669546046378 ) ) ;
#67120=CARTESIAN_POINT ( 'NONE',  ( 33.72732726872323639, -21.50529672980692908, -24.82116981130025124 ) ) ;
#67137=CARTESIAN_POINT ( 'NONE',  ( -36.91746825000000598, 2.428612866367529932E-14, -0.6249999972688132788 ) ) ;
#67147=CARTESIAN_POINT ( 'NONE',  ( 17.67029085834301227, -36.01944455193423522, -22.64778610421477723 ) ) ;
#67166=ORIENTED_EDGE ( 'NONE', *, *, #136461, .T. ) ;
#67185=DIRECTION ( 'NONE',  ( 0.000000000000000000, 0.000000000000000000, 1.000000000000000000 ) ) ;
#67196=CARTESIAN_POINT ( 'NONE',  ( 22.81625015709509441, 31.40387420917330275, -7.824999997268813345 ) ) ;
#67228=CARTESIAN_POINT ( 'NONE',  ( -15.06137443927351072, 15.06137443927345210, -56.46919128290398504 ) ) ;
#67230=CARTESIAN_POINT ( 'NONE',  ( -23.48529157249599919, -32.32473071737749848, -1.699999999999999956 ) ) ;
#67261=ORIENTED_EDGE ( 'NONE', *, *, #79473, .F. ) ;
#67338=CARTESIAN_POINT ( 'NONE',  ( 37.99999999999999289, 2.893978650043524126E-14, -5.000000000000000000 ) ) ;
#67339=B_SPLINE_CURVE_WITH_KNOTS ( 'NONE', 3,
 ( #15908, #172572, #125071, #77566, #93727, #713, #108901, #60404, #91720, #45254, #187759, #155409 ),
 .UNSPECIFIED., .F., .F.,
 ( 4, 2, 2, 2, 2, 4 ),
 ( 0.002611479512216078464, 0.003262097472420399501, 0.003912715432624720539, 0.004563333392829041144, 0.004888642372931204481, 0.005213951353033367819 ),
 .UNSPECIFIED. ) ;
#67341=CARTESIAN_POINT ( 'NONE',  ( 20.70663425419854420, 22.78165926218171222, -47.27781451939568313 ) ) ;
#67355=DIRECTION ( 'NONE',  ( 1.000000000000000000, 0.000000000000000000, 0.000000000000000000 ) ) ;
#67365=CARTESIAN_POINT ( 'NONE',  ( 22.55670631985092456, -22.55670631985084995, -49.13275782002545355 ) ) ;
#67367=CARTESIAN_POINT ( 'NONE',  ( 29.86685920354754842, -21.69954338932559068, -1.824999997268813345 ) ) ;
#67381=CARTESIAN_POINT ( 'NONE',  ( 11.40812507854755253, -35.11059874428192273, -10.52499999726881263 ) ) ;
#67401=EDGE_CURVE ( 'NONE', #28211, #173655, #191943, .T. ) ;
#67429=CARTESIAN_POINT ( 'NONE',  ( -29.86685920354755197, -21.69954338932560134, -4.924999997268813878 ) ) ;
#67483=VECTOR ( 'NONE', #148723, 1000.000000000000000 ) ;
#67516=CARTESIAN_POINT ( 'NONE',  ( -5.000000000000000888, 4.999999999999999112, -15.00000000000000000 ) ) ;
#67598=CARTESIAN_POINT ( 'NONE',  ( 17.59990181671015819, -15.82965471272139091, -54.72698953881466366 ) ) ;
#67622=CIRCLE ( 'NONE', #32137, 214.0437394197456911 ) ;
#67633=EDGE_CURVE ( 'NONE', #166185, #30659, #148266, .T. ) ;
#67646=EDGE_CURVE ( 'NONE', #17032, #120193, #116105, .T. ) ;
#67652=DIRECTION ( 'NONE',  ( 3.469446951953612217E-15, 0.000000000000000000, -1.000000000000000000 ) ) ;
#67663=ORIENTED_EDGE ( 'NONE', *, *, #186227, .T. ) ;
#67676=CARTESIAN_POINT ( 'NONE',  ( -1.376802789500885194, -29.79829367730026846, -48.54110828511537079 ) ) ;
#67689=CARTESIAN_POINT ( 'NONE',  ( -8.106210103297929237, -39.71824525391685512, -25.55638568641365893 ) ) ;
#67690=ORIENTED_EDGE ( 'NONE', *, *, #174924, .F. ) ;
#67712=CARTESIAN_POINT ( 'NONE',  ( 27.83212366386711523, -25.89052209088936607, -16.12745387078193815 ) ) ;
#67755=CARTESIAN_POINT ( 'NONE',  ( -5.361383004202544100, -6.881117414448073788, -61.98550895074578193 ) ) ;
#67796=AXIS2_PLACEMENT_3D ( 'NONE', #128420, #191111, #52585 ) ;
#67801=ORIENTED_EDGE ( 'NONE', *, *, #171282, .T. ) ;
#67822=CARTESIAN_POINT ( 'NONE',  ( -3.573655867282028392E-15, 2.428612866367529932E-14, -25.00000000000000000 ) ) ;
#67839=ORIENTED_EDGE ( 'NONE', *, *, #89447, .F. ) ;
#67842=CARTESIAN_POINT ( 'NONE',  ( 18.00321789565200703, -35.67122027912853355, -27.04300662093937291 ) ) ;
#67870=FACE_OUTER_BOUND ( 'NONE', #164723, .T. ) ;
#67893=ORIENTED_EDGE ( 'NONE', *, *, #67633, .F. ) ;
#67905=ORIENTED_EDGE ( 'NONE', *, *, #71198, .T. ) ;
#67915=SURFACE_STYLE_USAGE ( .BOTH. , #6236 ) ;
#67916=CARTESIAN_POINT ( 'NONE',  ( -38.00000000000000711, 2.428612866367529932E-14, -9.749999994537626336 ) ) ;
#67919=CARTESIAN_POINT ( 'NONE',  ( 25.38628342471155364, -27.91043139587388566, -20.44818103819207167 ) ) ;
#67946=LINE ( 'NONE', #178145, #136566 ) ;
#68000=EDGE_CURVE ( 'NONE', #53519, #101425, #83047, .T. ) ;
#68023=CARTESIAN_POINT ( 'NONE',  ( -29.44685852473304166, -27.07773368778541112, -16.45956342659044580 ) ) ;
#68072=CARTESIAN_POINT ( 'NONE',  ( -23.48529157249599919, -32.32473071737749848, -3.699999999999999734 ) ) ;
#68082=CARTESIAN_POINT ( 'NONE',  ( -26.28653040952168141, -27.04268878403664900, -20.33571853020666609 ) ) ;
#68107=CARTESIAN_POINT ( 'NONE',  ( 22.73749492396215288, -155.7167183371838064, -15.00000000000000178 ) ) ;
#68129=CARTESIAN_POINT ( 'NONE',  ( 30.74264578624799782, 22.33583958711400541, -0.7999999999999999334 ) ) ;
#68190=CARTESIAN_POINT ( 'NONE',  ( 29.86685920354754842, -21.69954338932559068, -8.324999997268813345 ) ) ;
#68198=DIRECTION ( 'NONE',  ( 1.000000000000000000, 0.000000000000000000, 0.000000000000000000 ) ) ;
#68244=EDGE_CURVE ( 'NONE', #190550, #116695, #63682, .T. ) ;
#68319=EDGE_CURVE ( 'NONE', #194525, #115704, #59403, .T. ) ;
#68337=FACE_OUTER_BOUND ( 'NONE', #63921, .T. ) ;
#68342=DIRECTION ( 'NONE',  ( 0.000000000000000000, 0.000000000000000000, 1.000000000000000000 ) ) ;
#68351=CARTESIAN_POINT ( 'NONE',  ( -32.99455490591380169, -22.60464286593628458, -23.90693389968298277 ) ) ;
#68361=CARTESIAN_POINT ( 'NONE',  ( 17.18269478283316332, -17.18269478283309226, -64.92279855667830191 ) ) ;
#68363=CARTESIAN_POINT ( 'NONE',  ( -36.91746825000000598, 2.428612866367529932E-14, -0.6249999972688132788 ) ) ;
#68420=AXIS2_PLACEMENT_3D ( 'NONE', #166962, #120434, #106258 ) ;
#68507=EDGE_CURVE ( 'NONE', #4269, #24637, #89754, .T. ) ;
#68589=CARTESIAN_POINT ( 'NONE',  ( -11.74264578624800670, 36.14014761921585972, -0.3999999999999999112 ) ) ;
#68592=CARTESIAN_POINT ( 'NONE',  ( -31.67901979315909600, 0.7913989229881625009, -49.40962234820035093 ) ) ;
#68606=CARTESIAN_POINT ( 'NONE',  ( 0.000000000000000000, 0.000000000000000000, -61.34707691135562868 ) ) ;
#68608=CARTESIAN_POINT ( 'NONE',  ( 0.000000000000000000, 0.000000000000000000, -65.00100000000003320 ) ) ;
#68620=CARTESIAN_POINT ( 'NONE',  ( 22.99604614807110892, -21.65681935926113866, -46.12383121077565562 ) ) ;
#68623=CARTESIAN_POINT ( 'NONE',  ( -9.687362902255733488, 9.687362902255692632, -62.58071313852362039 ) ) ;
#68627=CARTESIAN_POINT ( 'NONE',  ( 26.58214507596527199, -26.75488679838896289, -20.35119661315284390 ) ) ;
#68662=CARTESIAN_POINT ( 'NONE',  ( -1.245073757422965999, -21.94104750614015487, -58.42286556281734988 ) ) ;
#68671=CARTESIAN_POINT ( 'NONE',  ( -0.1353689087803485180, -28.90000000000005187, -49.67367017693150899 ) ) ;
#68677=ORIENTED_EDGE ( 'NONE', *, *, #28409, .T. ) ;
#68683=CARTESIAN_POINT ( 'NONE',  ( -14.09403216839727158, -37.74807521950489075, -24.22002746647715554 ) ) ;
#68695=CARTESIAN_POINT ( 'NONE',  ( 9.244353370540800086, 10.58303160951403221, -62.45107349144919340 ) ) ;
#68710=CARTESIAN_POINT ( 'NONE',  ( 69.65682714487590488, -71.74905178543389184, -15.00000000000000178 ) ) ;
#68748=AXIS2_PLACEMENT_3D ( 'NONE', #156783, #126428, #18276 ) ;
#68827=B_SPLINE_CURVE_WITH_KNOTS ( 'NONE', 3,
 ( #82712, #147409, #8896, #70564, #193924, #37222, #40216, #148405, #56391, #10897, #89720, #117057, #71560, #57406, #25077, #58388, #28080, #88722, #178752, #120055 ),
 .UNSPECIFIED., .F., .F.,
 ( 4, 2, 2, 2, 2, 2, 2, 2, 2, 4 ),
 ( 2.784207231363245562E-07, 0.0003311547508960723256, 0.0006620310810690082683, 0.0009929074112419442651, 0.001323783741414880262, 0.002647289062106632923, 0.003309041722452508820, 0.003970794382798385584, 0.004632547043144262348, 0.005294299703490139113 ),
 .UNSPECIFIED. ) ;
#68840=ORIENTED_EDGE ( 'NONE', *, *, #110986, .T. ) ;
#68843=CARTESIAN_POINT ( 'NONE',  ( 193.3062444957835453, -155.7167183371837496, -15.00000000000000178 ) ) ;
#68880=CARTESIAN_POINT ( 'NONE',  ( 23.48529157249600630, -32.32473071737748427, -5.049999994537627046 ) ) ;
#68898=AXIS2_PLACEMENT_3D ( 'NONE', #31934, #15772, #76440 ) ;
#68908=ORIENTED_EDGE ( 'NONE', *, *, #163998, .T. ) ;
#68917=SHAPE_REPRESENTATION_RELATIONSHIP ( 'NONE' , 'NONE' ,  #92179, #100331 ) ;
#68921=CARTESIAN_POINT ( 'NONE',  ( 24.48191864109216098, -29.02791343561681003, -16.65471697699033982 ) ) ;
#68948=EDGE_LOOP ( 'NONE', ( #43973, #42107, #58434, #7114 ) ) ;
#68989=DIRECTION ( 'NONE',  ( -1.000000000000000000, 1.065814103640150121E-14, 0.000000000000000000 ) ) ;
#69022=CARTESIAN_POINT ( 'NONE',  ( 69.65682714487590488, -71.74905178543389184, -15.00000000000000178 ) ) ;
#69099=VERTEX_POINT ( 'NONE', #138243 ) ;
#69101=CIRCLE ( 'NONE', #94941, 59.99999999999998579 ) ;
#69107=CARTESIAN_POINT ( 'NONE',  ( -30.27664185797782537, 1.503321482105818507, -47.91583118997741053 ) ) ;
#69132=CARTESIAN_POINT ( 'NONE',  ( 23.48529157249599919, 32.32473071737754111, -0.6999999999999998446 ) ) ;
#69149=EDGE_CURVE ( 'NONE', #14377, #70166, #36716, .T. ) ;
#69163=ORIENTED_EDGE ( 'NONE', *, *, #140897, .T. ) ;
#69170=DIRECTION ( 'NONE',  ( -0.000000000000000000, 0.000000000000000000, 1.000000000000000000 ) ) ;
#69194=CARTESIAN_POINT ( 'NONE',  ( -11.40812507854755609, 35.11059874428196537, -5.024999997268813523 ) ) ;
#69231=CARTESIAN_POINT ( 'NONE',  ( 31.88380457335793849, -0.2515199893712269930, -49.15318026754363245 ) ) ;
#69328=ORIENTED_EDGE ( 'NONE', *, *, #4868, .F. ) ;
#69341=CARTESIAN_POINT ( 'NONE',  ( 22.55670631985092811, 22.55670631985084640, -45.64921306006598201 ) ) ;
#69367=CARTESIAN_POINT ( 'NONE',  ( -29.86685920354755197, -21.69954338932560134, -2.424999997268813434 ) ) ;
#69376=DIRECTION ( 'NONE',  ( 1.000000000000000000, 0.000000000000000000, 0.000000000000000000 ) ) ;
#69417=DIRECTION ( 'NONE',  ( -0.000000000000000000, -0.000000000000000000, 1.000000000000000000 ) ) ;
#69428=CARTESIAN_POINT ( 'NONE',  ( 29.14368513529645099, -0.8274645171313743663, -49.37167794572895474 ) ) ;
#69442=CARTESIAN_POINT ( 'NONE',  ( 14.61899031675406846, 16.10093921903347081, -58.57166825620328154 ) ) ;
#69455=ORIENTED_EDGE ( 'NONE', *, *, #149391, .T. ) ;
#69481=VECTOR ( 'NONE', #153273, 1000.000000000000000 ) ;
#69503=VERTEX_POINT ( 'NONE', #75569 ) ;
#69519=DIRECTION ( 'NONE',  ( 1.000000000000000000, 0.000000000000000000, 0.000000000000000000 ) ) ;
#69579=CARTESIAN_POINT ( 'NONE',  ( 69.65682714487590488, -71.74905178543389184, 0.000000000000000000 ) ) ;
#69583=CARTESIAN_POINT ( 'NONE',  ( 11.82759615478249593, -9.696917953820088698, -61.96080966668566248 ) ) ;
#69601=CARTESIAN_POINT ( 'NONE',  ( -29.18776880969891607, 0.8894290736110457285, -52.33677266386640525 ) ) ;
#69621=CARTESIAN_POINT ( 'NONE',  ( 38.00000000000000711, -12.34694845685040754, -4.849999994537625092 ) ) ;
#69637=ORIENTED_EDGE ( 'NONE', *, *, #133011, .F. ) ;
#69655=CARTESIAN_POINT ( 'NONE',  ( 0.000000000000000000, 0.000000000000000000, -25.00000000000000000 ) ) ;
#69657=ADVANCED_FACE ( 'NONE', ( #47236, #153408, #33060, #94715, #137245, #93721, #141220, #170574, #32065, #45248, #168575, #76568, #199927, #61390, #46233, #173568, #37021, #126056 ), #175546, .T. ) ;
#69659=DIRECTION ( 'NONE',  ( -1.000000000000000000, 0.000000000000000000, 0.000000000000000000 ) ) ;
#69670=CARTESIAN_POINT ( 'NONE',  ( 22.81625015709510151, -31.40387420917324590, -6.424999997268811214 ) ) ;
#69680=DIRECTION ( 'NONE',  ( -0.000000000000000000, -0.000000000000000000, -1.000000000000000000 ) ) ;
#69686=LINE ( 'NONE', #162692, #176945 ) ;
#69692=CARTESIAN_POINT ( 'NONE',  ( -6.767138868727710310, -40.03474714072286389, -25.59093536067524610 ) ) ;
#69702=DIRECTION ( 'NONE',  ( 1.000000000000000000, 0.000000000000000000, 0.000000000000000000 ) ) ;
#69703=EDGE_LOOP ( 'NONE', ( #56921, #199659, #181360, #98385 ) ) ;
#69720=DIRECTION ( 'NONE',  ( -1.000000000000000000, 0.000000000000000000, 0.000000000000000000 ) ) ;
#69806=ADVANCED_FACE ( 'NONE', ( #112865 ), #34052, .F. ) ;
#69826=CARTESIAN_POINT ( 'NONE',  ( -21.64789649210654687, -31.17538106138195175, -22.95353217465975249 ) ) ;
#69865=EDGE_LOOP ( 'NONE', ( #143208, #75584, #99403, #99520 ) ) ;
#69876=CARTESIAN_POINT ( 'NONE',  ( 0.000000000000000000, 0.000000000000000000, -64.92279855667830191 ) ) ;
#69879=CARTESIAN_POINT ( 'NONE',  ( -6.020228577223754586E-15, 39.95556452105416412, -4.500000000000000888 ) ) ;
#69894=CARTESIAN_POINT ( 'NONE',  ( -16.64782025964801093, 0.4052355915355428384, -59.15693706287431297 ) ) ;
#69926=FILL_AREA_STYLE_COLOUR ( '', #182283 ) ;
#69927=CARTESIAN_POINT ( 'NONE',  ( 11.74264578624799427, 36.14014761921585972, -10.34999999453762598 ) ) ;
#69935=VERTEX_POINT ( 'NONE', #127032 ) ;
#69994=DIRECTION ( 'NONE',  ( 0.000000000000000000, 0.000000000000000000, 1.000000000000000000 ) ) ;
#70095=CARTESIAN_POINT ( 'NONE',  ( 1.499999999999961586, 30.23919084766313858, -51.14197153238884397 ) ) ;
#70107=DIRECTION ( 'NONE',  ( 0.000000000000000000, 0.000000000000000000, 1.000000000000000000 ) ) ;
#70117=CARTESIAN_POINT ( 'NONE',  ( -38.00000000000000711, 2.893978650043524126E-14, -15.00000000000000000 ) ) ;
#70121=CARTESIAN_POINT ( 'NONE',  ( 4.313351365237948265, 4.313351365237946489, -62.50719930893269805 ) ) ;
#70123=CARTESIAN_POINT ( 'NONE',  ( 16.70000000000002416, -0.1037895044722859789, -59.13370768023892055 ) ) ;
#70127=CARTESIAN_POINT ( 'NONE',  ( 11.30153831258471797, -180.0000000000000000, -14.99999999999999822 ) ) ;
#70133=CARTESIAN_POINT ( 'NONE',  ( 6.938893903907228378E-15, 22.80000000000002913, -65.00100000000003320 ) ) ;
#70135=AXIS2_PLACEMENT_3D ( 'NONE', #118619, #114595, #176292 ) ;
#70142=CARTESIAN_POINT ( 'NONE',  ( 22.81625015709509441, 31.40387420917330275, -9.324999997268813345 ) ) ;
#70145=VECTOR ( 'NONE', #137229, 1000.000000000000000 ) ;
#70152=CARTESIAN_POINT ( 'NONE',  ( 30.57338251523173156, -25.88377959333006118, -17.25078043576312936 ) ) ;
#70161=CARTESIAN_POINT ( 'NONE',  ( -6.434671708797631950, -6.434671708797536027, -61.89430850415821794 ) ) ;
#70166=VERTEX_POINT ( 'NONE', #18890 ) ;
#70168=EDGE_CURVE ( 'NONE', #137721, #74853, #80536, .T. ) ;
#70174=VERTEX_POINT ( 'NONE', #97672 ) ;
#70205=CARTESIAN_POINT ( 'NONE',  ( 36.91746824999999177, 2.880721459617395097E-14, -3.624999997268813168 ) ) ;
#70210=CARTESIAN_POINT ( 'NONE',  ( 6.542287240554228056, -4.421942842314275701, -64.21309694765785991 ) ) ;
#70235=FACE_OUTER_BOUND ( 'NONE', #35973, .T. ) ;
#70245=CYLINDRICAL_SURFACE ( 'NONE', #28986, 2.500000000000000000 ) ;
#70273=VERTEX_POINT ( 'NONE', #81509 ) ;
#70315=AXIS2_PLACEMENT_3D ( 'NONE', #176829, #4947, #189994 ) ;
#70377=CARTESIAN_POINT ( 'NONE',  ( 36.91746824999999177, 2.880721459617395097E-14, -3.624999997268813168 ) ) ;
#70386=CYLINDRICAL_SURFACE ( 'NONE', #143133, 2.500000000000000000 ) ;
#70398=CARTESIAN_POINT ( 'NONE',  ( 1.508955259217861487E-14, -71.74905152827281540, -24.99410988490251029 ) ) ;
#70435=CARTESIAN_POINT ( 'NONE',  ( 29.20736712825158321, -0.9155518048963849909, -49.29216761470111408 ) ) ;
#70461=ORIENTED_EDGE ( 'NONE', *, *, #192965, .F. ) ;
#70525=CYLINDRICAL_SURFACE ( 'NONE', #75622, 38.00000000000000000 ) ;
#70547=CARTESIAN_POINT ( 'NONE',  ( -30.74264578624800492, 22.33583958711400186, -1.949999994537626735 ) ) ;
#70564=CARTESIAN_POINT ( 'NONE',  ( -15.41147372653650116, 14.79648886421073506, -56.42550976940268015 ) ) ;
#70582=CARTESIAN_POINT ( 'NONE',  ( -2.662494480112494788, -37.13692398601925504, -32.59999999999999432 ) ) ;
#70589=CARTESIAN_POINT ( 'NONE',  ( -0.7792920370541464026, -16.49741402511618915, -61.43171317168469869 ) ) ;
#70611=CARTESIAN_POINT ( 'NONE',  ( 11.62258226397313798, -9.495678640448794283, -59.91195431507608049 ) ) ;
#70618=ORIENTED_EDGE ( 'NONE', *, *, #137192, .T. ) ;
#70624=CARTESIAN_POINT ( 'NONE',  ( 27.00987238947314850, -29.10436634937579115, -20.14159902729967300 ) ) ;
#70627=CARTESIAN_POINT ( 'NONE',  ( 23.48529157249599919, 32.32473071737754111, -4.449999994537627401 ) ) ;
#70641=CARTESIAN_POINT ( 'NONE',  ( 6.434671708797586653, 6.434671708797580436, -63.95112321872120731 ) ) ;
#70664=FACE_OUTER_BOUND ( 'NONE', #77511, .T. ) ;
#70679=CARTESIAN_POINT ( 'NONE',  ( -11.40812507854754720, -35.11059874428192273, -6.724999997268813701 ) ) ;
#70700=CARTESIAN_POINT ( 'NONE',  ( -24.59647911869062042, -31.70815657101477925, -17.34206816075075253 ) ) ;
#70701=VERTEX_POINT ( 'NONE', #2350 ) ;
#70710=CARTESIAN_POINT ( 'NONE',  ( 9.408549014593489801, 11.42987701755554752, -62.15975709196300869 ) ) ;
#70715=CARTESIAN_POINT ( 'NONE',  ( 0.000000000000000000, 0.000000000000000000, -62.58071313852362039 ) ) ;
#70721=EDGE_CURVE ( 'NONE', #12139, #114764, #180063, .T. ) ;
#70736=CARTESIAN_POINT ( 'NONE',  ( -1.197744245042869471, -6.691772886347793659, -62.38710104649958055 ) ) ;
#70768=DIRECTION ( 'NONE',  ( 0.000000000000000000, 0.000000000000000000, 1.000000000000000000 ) ) ;
#70830=CARTESIAN_POINT ( 'NONE',  ( -11.74264578624800670, 36.14014761921585972, -6.400000000000000355 ) ) ;
#70849=ORIENTED_EDGE ( 'NONE', *, *, #200059, .T. ) ;
#70861=AXIS2_PLACEMENT_3D ( 'NONE', #159828, #86988, #21323 ) ;
#70879=LINE ( 'NONE', #73883, #67483 ) ;
#70898=DIRECTION ( 'NONE',  ( -1.000000000000000000, -6.938893903907222461E-16, -0.000000000000000000 ) ) ;
#70905=ORIENTED_EDGE ( 'NONE', *, *, #58993, .F. ) ;
#70928=CARTESIAN_POINT ( 'NONE',  ( -23.48529157249600985, 32.32473071737754111, -10.04999999453762705 ) ) ;
#70959=ORIENTED_EDGE ( 'NONE', *, *, #72533, .F. ) ;
#70961=AXIS2_PLACEMENT_3D ( 'NONE', #98554, #160248, #117745 ) ;
#70995=ORIENTED_EDGE ( 'NONE', *, *, #140816, .T. ) ;
#70996=CARTESIAN_POINT ( 'NONE',  ( 21.30000000000002913, 0.000000000000000000, -56.46919128290398504 ) ) ;
#71036=DIRECTION ( 'NONE',  ( 1.000000000000000000, 0.000000000000000000, 0.000000000000000000 ) ) ;
#71084=VERTEX_POINT ( 'NONE', #156035 ) ;
#71093=CARTESIAN_POINT ( 'NONE',  ( 1.358751706670194404, 29.75846941761153985, -51.69462059227841877 ) ) ;
#71105=AXIS2_PLACEMENT_3D ( 'NONE', #173564, #5679, #67355 ) ;
#71118=DIRECTION ( 'NONE',  ( 1.000000000000000000, 0.000000000000000000, 0.000000000000000000 ) ) ;
#71122=CARTESIAN_POINT ( 'NONE',  ( 23.48529157249600630, -32.32473071737748427, -7.049999994537626158 ) ) ;
#71126=CARTESIAN_POINT ( 'NONE',  ( 32.61313261257514284, -23.16473864289021378, -21.41836715626212495 ) ) ;
#71136=CIRCLE ( 'NONE', #109943, 12.00000000000000000 ) ;
#71140=ORIENTED_EDGE ( 'NONE', *, *, #2746, .F. ) ;
#71143=CARTESIAN_POINT ( 'NONE',  ( -11.74264578624800670, 36.14014761921585972, -2.400000000000000355 ) ) ;
#71160=DIRECTION ( 'NONE',  ( -1.000000000000000000, 0.000000000000000000, 0.000000000000000000 ) ) ;
#71168=EDGE_LOOP ( 'NONE', ( #75864, #52922, #178029, #6159, #24356 ) ) ;
#71170=CARTESIAN_POINT ( 'NONE',  ( -9.248023074035629065, -10.74802307403544077, -60.25555373585994090 ) ) ;
#71198=EDGE_CURVE ( 'NONE', #193343, #40990, #43907, .T. ) ;
#71204=CARTESIAN_POINT ( 'NONE',  ( -22.81625015709509441, -31.40387420917324590, -4.324999997268812457 ) ) ;
#71238=CARTESIAN_POINT ( 'NONE',  ( 0.000000000000000000, -105.0000000000000000, 12.00000000000000355 ) ) ;
#71243=DIRECTION ( 'NONE',  ( 1.000000000000000000, 0.000000000000000000, 0.000000000000000000 ) ) ;
#71273=ORIENTED_EDGE ( 'NONE', *, *, #55067, .T. ) ;
#71291=ADVANCED_FACE ( 'NONE', ( #183999 ), #15143, .F. ) ;
#71358=CARTESIAN_POINT ( 'NONE',  ( -14.98843538525856722, -15.13431349328839914, -58.85720012050613548 ) ) ;
#71367=CARTESIAN_POINT ( 'NONE',  ( -27.81822689058051878, -28.32190533958856449, -20.09416750255129713 ) ) ;
#71378=CARTESIAN_POINT ( 'NONE',  ( 29.86685920354754487, 21.69954338932564752, -3.424999997268813434 ) ) ;
#71435=CARTESIAN_POINT ( 'NONE',  ( 0.000000000000000000, 0.000000000000000000, -62.50719930893269805 ) ) ;
#71451=VERTEX_POINT ( 'NONE', #76805 ) ;
#71476=PLANE ( 'NONE',  #146739 ) ;
#71560=CARTESIAN_POINT ( 'NONE',  ( -17.41439684931615517, 15.33930553228139004, -55.09142748592167038 ) ) ;
#71577=CARTESIAN_POINT ( 'NONE',  ( -8.779096689238560458, -37.67883572780603174, -23.98624440746952757 ) ) ;
#71583=CARTESIAN_POINT ( 'NONE',  ( -1.322671946311490432, -15.93273212980864173, -61.66661032175889545 ) ) ;
#71596=DIRECTION ( 'NONE',  ( -0.000000000000000000, -0.000000000000000000, 1.000000000000000000 ) ) ;
#71599=DIRECTION ( 'NONE',  ( -0.000000000000000000, -0.000000000000000000, 1.000000000000000000 ) ) ;
#71604=CARTESIAN_POINT ( 'NONE',  ( 9.687362902255731711, -9.687362902255694408, -60.44446360152740993 ) ) ;
#71616=CARTESIAN_POINT ( 'NONE',  ( 22.78725946537545965, -32.81619059092827939, -22.84582334174698559 ) ) ;
#71620=CARTESIAN_POINT ( 'NONE',  ( 11.74264578624799427, 36.14014761921585972, -8.349999994537625980 ) ) ;
#71659=CARTESIAN_POINT ( 'NONE',  ( 0.000000000000000000, 0.000000000000000000, -64.53213882399991519 ) ) ;
#71670=CARTESIAN_POINT ( 'NONE',  ( -11.40812507854755609, 35.11059874428196537, -5.524999997268813523 ) ) ;
#71693=CARTESIAN_POINT ( 'NONE',  ( -24.90102501248286160, -31.06609936492528945, -21.12314233236282845 ) ) ;
#71694=ORIENTED_EDGE ( 'NONE', *, *, #188107, .T. ) ;
#71719=CARTESIAN_POINT ( 'NONE',  ( 0.5019701148545779867, 16.61710099588754019, -61.38173178550033526 ) ) ;
#71826=CARTESIAN_POINT ( 'NONE',  ( -26.58214507596518672, -26.75488679838906947, -20.35119661315286521 ) ) ;
#71847=DIRECTION ( 'NONE',  ( -0.000000000000000000, -0.000000000000000000, -1.000000000000000000 ) ) ;
#71862=ORIENTED_EDGE ( 'NONE', *, *, #196878, .F. ) ;
#71873=FACE_OUTER_BOUND ( 'NONE', #155655, .T. ) ;
#71892=CARTESIAN_POINT ( 'NONE',  ( 8.945614359730875265, -0.6701480022146872884, -63.98123544873406132 ) ) ;
#71928=VERTEX_POINT ( 'NONE', #154645 ) ;
#71952=ORIENTED_EDGE ( 'NONE', *, *, #51668, .T. ) ;
#71987=CARTESIAN_POINT ( 'NONE',  ( 0.7618971401916020403, 6.292798783326192691, -64.49505886858686665 ) ) ;
#72008=DIRECTION ( 'NONE',  ( 1.000000000000000000, 0.000000000000000000, 0.000000000000000000 ) ) ;
#72025=CARTESIAN_POINT ( 'NONE',  ( -11.74264578624799782, -36.14014761921581709, -3.349999994537626868 ) ) ;
#72080=CARTESIAN_POINT ( 'NONE',  ( 30.74264578624800137, -22.33583958711395212, -3.200000000000000178 ) ) ;
#72114=B_SPLINE_CURVE_WITH_KNOTS ( 'NONE', 3,
 ( #129290, #175822, #160644, #18169, #83786, #189015, #145465, #2980, #64659, #49490, #172841, #34320, #95983, #65642, #50489, #178831, #134321, #181818, #102971, #164656, #84784, #40300, #146463, #7955, #72647, #24150, #23139, #54471 ),
 .UNSPECIFIED., .F., .F.,
 ( 4, 2, 2, 2, 2, 2, 2, 2, 2, 2, 2, 2, 2, 4 ),
 ( 1.961533960389205320E-07, 0.0003775868847195711629, 0.0007549776160431033488, 0.001132368347366635806, 0.001509759078690167938, 0.002264540541337212252, 0.003019322003984256566, 0.003774103466631300880, 0.004151494197954830843, 0.004528884929278359506, 0.004906275660601889903, 0.005283666391925419432, 0.005661057123248948962, 0.006038447854572478492 ),
 .UNSPECIFIED. ) ;
#72117=FACE_OUTER_BOUND ( 'NONE', #131810, .T. ) ;
#72122=CARTESIAN_POINT ( 'NONE',  ( 0.000000000000000000, 0.000000000000000000, -65.00100000000003320 ) ) ;
#72130=FACE_OUTER_BOUND ( 'NONE', #169521, .T. ) ;
#72138=CARTESIAN_POINT ( 'NONE',  ( 22.81625015709510151, -31.40387420917324590, -7.924999997268812990 ) ) ;
#72154=AXIS2_PLACEMENT_3D ( 'NONE', #68606, #23118, #176812 ) ;
#72166=CARTESIAN_POINT ( 'NONE',  ( 6.020883695542538661, -38.43099163646597560, -23.90977630326271353 ) ) ;
#72173=EDGE_CURVE ( 'NONE', #94189, #27850, #132602, .T. ) ;
#72201=CARTESIAN_POINT ( 'NONE',  ( 36.91746825000000598, -11.99521256947793546, -7.724999997268812812 ) ) ;
#72230=DIRECTION ( 'NONE',  ( 1.000000000000000000, 0.000000000000000000, 0.000000000000000000 ) ) ;
#72263=EDGE_LOOP ( 'NONE', ( #118839, #79880, #155116, #150361 ) ) ;
#72352=CARTESIAN_POINT ( 'NONE',  ( -28.47622644277399928, -25.16156846422451920, -16.68312038616162951 ) ) ;
#72377=CARTESIAN_POINT ( 'NONE',  ( 11.40812507854754365, 35.11059874428196537, -9.224999997268813701 ) ) ;
#72384=ORIENTED_EDGE ( 'NONE', *, *, #38861, .F. ) ;
#72388=CARTESIAN_POINT ( 'NONE',  ( -3.573655867282028392E-15, 2.428612866367529932E-14, -25.00000000000000000 ) ) ;
#72434=AXIS2_PLACEMENT_3D ( 'NONE', #91069, #44600, #149791 ) ;
#72437=CARTESIAN_POINT ( 'NONE',  ( 30.74964850363291546, -1.467638476639183009, -47.27948696604331502 ) ) ;
#72457=ORIENTED_EDGE ( 'NONE', *, *, #151524, .F. ) ;
#72464=EDGE_CURVE ( 'NONE', #84310, #85102, #125174, .T. ) ;
#72465=ORIENTED_EDGE ( 'NONE', *, *, #79617, .F. ) ;
#72514=EDGE_LOOP ( 'NONE', ( #22064, #148295, #113623, #178558, #92196, #113988, #197660, #162618, #97000 ) ) ;
#72533=EDGE_CURVE ( 'NONE', #197947, #144280, #176850, .T. ) ;
#72558=VECTOR ( 'NONE', #134446, 1000.000000000000000 ) ;
#72594=CARTESIAN_POINT ( 'NONE',  ( 0.4098915413868572943, 13.74273402794541177, -60.42614997978301972 ) ) ;
#72616=CIRCLE ( 'NONE', #117929, 214.0437394197456911 ) ;
#72621=ORIENTED_EDGE ( 'NONE', *, *, #75628, .T. ) ;
#72630=CARTESIAN_POINT ( 'NONE',  ( -11.74264578624799782, -36.14014761921581709, -9.349999994537627757 ) ) ;
#72642=CARTESIAN_POINT ( 'NONE',  ( -9.840250911107732534, 9.549542882988092174, -60.43989527633940639 ) ) ;
#72647=CARTESIAN_POINT ( 'NONE',  ( -0.4911207797134861108, -28.97745891950397024, -52.56957762865166472 ) ) ;
#72654=CARTESIAN_POINT ( 'NONE',  ( 11.30153831258470021, -180.0000000000000000, -15.00000000000000178 ) ) ;
#72676=AXIS2_PLACEMENT_3D ( 'NONE', #26234, #24233, #179925 ) ;
#72679=EDGE_CURVE ( 'NONE', #93860, #112813, #63823, .T. ) ;
#72681=CARTESIAN_POINT ( 'NONE',  ( -5.950531402560715689E-15, 38.81732327939063509, -1.624999997268813390 ) ) ;
#72696=CARTESIAN_POINT ( 'NONE',  ( -9.100000000000001421, 9.789526074884739315E-14, -63.95112321872120731 ) ) ;
#72704=CARTESIAN_POINT ( 'NONE',  ( -30.36026264928165119, -25.76863830326744775, -21.12575414590727618 ) ) ;
#72720=CARTESIAN_POINT ( 'NONE',  ( -0.9199430937698453992, -8.788868155854853370, -64.01178436185549003 ) ) ;
#72734=CARTESIAN_POINT ( 'NONE',  ( 8.725106586199796510, -0.9968436689772890436, -64.02420483255117745 ) ) ;
#72776=CARTESIAN_POINT ( 'NONE',  ( 2.500000000000000000, -165.0000000000000000, 12.00000000000000355 ) ) ;
#72845=EDGE_CURVE ( 'NONE', #30659, #104408, #104446, .T. ) ;
#72864=DIRECTION ( 'NONE',  ( 1.000000000000000000, 0.000000000000000000, 0.000000000000000000 ) ) ;
#72872=AXIS2_PLACEMENT_3D ( 'NONE', #97033, #3054, #7017 ) ;
#72890=CARTESIAN_POINT ( 'NONE',  ( 20.23564678862950927, 22.32700255269481104, -51.30755147637196956 ) ) ;
#72895=CARTESIAN_POINT ( 'NONE',  ( -9.574135874901902099, -11.69267847920397685, -59.86604769085835187 ) ) ;
#72911=CARTESIAN_POINT ( 'NONE',  ( 4.158454644149660595, -48.51789971941278168, -23.00000000000000000 ) ) ;
#73041=CARTESIAN_POINT ( 'NONE',  ( 9.656827144875922642, -71.74905178543389184, -15.00000000000000178 ) ) ;
#73047=CARTESIAN_POINT ( 'NONE',  ( -5.000000000000000000, 6.123233995736766282E-16, -18.00000000000000000 ) ) ;
#73052=CIRCLE ( 'NONE', #89051, 69.99999999999997158 ) ;
#73091=VERTEX_POINT ( 'NONE', #14903 ) ;
#73095=ORIENTED_EDGE ( 'NONE', *, *, #137670, .F. ) ;
#73153=EDGE_CURVE ( 'NONE', #116695, #41844, #53556, .T. ) ;
#73154=ORIENTED_EDGE ( 'NONE', *, *, #156319, .T. ) ;
#73157=CARTESIAN_POINT ( 'NONE',  ( 38.00000000000000000, 12.34694845685046616, -2.900000000000000355 ) ) ;
#73184=CARTESIAN_POINT ( 'NONE',  ( 7.980598154334715311, -36.52039581308737581, -31.83703727319202414 ) ) ;
#73194=CARTESIAN_POINT ( 'NONE',  ( -6.918342302711550929, -47.27039221922506584, -24.65254351866712668 ) ) ;
#73215=CARTESIAN_POINT ( 'NONE',  ( 3.556970738554033499E-15, -38.81732327939057825, -6.124999997268812280 ) ) ;
#73248=DIRECTION ( 'NONE',  ( -0.000000000000000000, -0.000000000000000000, -1.000000000000000000 ) ) ;
#73257=EDGE_CURVE ( 'NONE', #149684, #185073, #181441, .T. ) ;
#73293=CYLINDRICAL_SURFACE ( 'NONE', #143915, 61.99999999999998579 ) ;
#73335=ORIENTED_EDGE ( 'NONE', *, *, #84390, .F. ) ;
#73365=FACE_OUTER_BOUND ( 'NONE', #104942, .T. ) ;
#73390=CARTESIAN_POINT ( 'NONE',  ( -36.91746825000000598, -11.99521256947794789, -8.524999997268812635 ) ) ;
#73400=CARTESIAN_POINT ( 'NONE',  ( 28.26755983467668898, -28.30239183792592428, -15.36609880857821153 ) ) ;
#73410=CARTESIAN_POINT ( 'NONE',  ( -21.49604614807126524, -21.49604614807088154, -64.92279855667830191 ) ) ;
#73447=DIRECTION ( 'NONE',  ( -0.000000000000000000, -0.000000000000000000, 1.000000000000000000 ) ) ;
#73471=VERTEX_POINT ( 'NONE', #151935 ) ;
#73481=AXIS2_PLACEMENT_3D ( 'NONE', #185246, #60892, #134791 ) ;
#73495=EDGE_CURVE ( 'NONE', #127301, #42534, #141326, .T. ) ;
#73526=SURFACE_STYLE_USAGE ( .BOTH. , #180711 ) ;
#73609=CARTESIAN_POINT ( 'NONE',  ( 0.000000000000000000, 0.000000000000000000, -25.00000000000000000 ) ) ;
#73619=AXIS2_PLACEMENT_3D ( 'NONE', #198496, #75141, #151015 ) ;
#73632=CARTESIAN_POINT ( 'NONE',  ( 23.48529157249599919, 32.32473071737754111, -6.449999994537626513 ) ) ;
#73640=CARTESIAN_POINT ( 'NONE',  ( -14.62203461105304036, -16.12203461105356794, -56.14925526931841659 ) ) ;
#73671=CARTESIAN_POINT ( 'NONE',  ( 11.80868324581538253, -11.80868324581533457, -64.92279855667830191 ) ) ;
#73679=ORIENTED_EDGE ( 'NONE', *, *, #91683, .F. ) ;
#73683=CARTESIAN_POINT ( 'NONE',  ( -11.40812507854755609, 35.11059874428196537, -7.524999997268813523 ) ) ;
#73700=ORIENTED_EDGE ( 'NONE', *, *, #11846, .F. ) ;
#73706=CARTESIAN_POINT ( 'NONE',  ( -24.05628303387027600, -31.51879896407069737, -19.31700871830652844 ) ) ;
#73732=CARTESIAN_POINT ( 'NONE',  ( 8.516692751257743055, -1.203296689329369729, -64.06477955746662190 ) ) ;
#73835=CARTESIAN_POINT ( 'NONE',  ( -6.824288631998610022, 4.978841623633250890, -62.04929096494494445 ) ) ;
#73852=ORIENTED_EDGE ( 'NONE', *, *, #119482, .T. ) ;
#73883=CARTESIAN_POINT ( 'NONE',  ( -38.00000000000000711, 2.893978650043524126E-14, -25.00000000000000000 ) ) ;
#73898=DIRECTION ( 'NONE',  ( -0.000000000000000000, -0.000000000000000000, 1.000000000000000000 ) ) ;
#73903=CARTESIAN_POINT ( 'NONE',  ( 9.979912183652610125, -44.24332767168409930, -21.75883150241362429 ) ) ;
#73921=DIRECTION ( 'NONE',  ( -0.000000000000000000, -0.000000000000000000, 1.000000000000000000 ) ) ;
#73927=CARTESIAN_POINT ( 'NONE',  ( -5.183909576824695442, 3.882848763669461967, -64.47227361656568689 ) ) ;
#73963=ORIENTED_EDGE ( 'NONE', *, *, #44832, .F. ) ;
#73995=EDGE_LOOP ( 'NONE', ( #46826, #144997, #194438, #189 ) ) ;
#74016=DIRECTION ( 'NONE',  ( -0.000000000000000000, -0.000000000000000000, 1.000000000000000000 ) ) ;
#74084=ORIENTED_EDGE ( 'NONE', *, *, #26286, .T. ) ;
#74124=CARTESIAN_POINT ( 'NONE',  ( -0.5379555815578647149, -24.20415418211123892, -54.28961862586980658 ) ) ;
#74139=ORIENTED_EDGE ( 'NONE', *, *, #172113, .F. ) ;
#74142=CARTESIAN_POINT ( 'NONE',  ( -38.00000000000001421, 12.34694845685046438, -4.100000000000000533 ) ) ;
#74168=ORIENTED_EDGE ( 'NONE', *, *, #90391, .F. ) ;
#74187=VECTOR ( 'NONE', #20314, 1000.000000000000000 ) ;
#74195=CARTESIAN_POINT ( 'NONE',  ( -4.313351365237961588, 4.313351365237934054, -62.50719930893269805 ) ) ;
#74196=ORIENTED_EDGE ( 'NONE', *, *, #115703, .T. ) ;
#74269=ORIENTED_EDGE ( 'NONE', *, *, #119223, .T. ) ;
#74303=ADVANCED_FACE ( 'NONE', ( #171076 ), #112381, .F. ) ;
#74355=CARTESIAN_POINT ( 'NONE',  ( -14.81363604427072644, -15.38158542220645408, -58.82267548686223080 ) ) ;
#74363=CARTESIAN_POINT ( 'NONE',  ( 1.500000000004810818, 7.599999999999482725, -64.24270632869257724 ) ) ;
#74373=CARTESIAN_POINT ( 'NONE',  ( 29.86685920354754487, 21.69954338932564752, -9.424999997268814766 ) ) ;
#74430=DIRECTION ( 'NONE',  ( 0.000000000000000000, 0.000000000000000000, 1.000000000000000000 ) ) ;
#74445=EDGE_CURVE ( 'NONE', #117961, #182543, #154157, .T. ) ;
#74517=EDGE_CURVE ( 'NONE', #185763, #30659, #157899, .T. ) ;
#74597=CARTESIAN_POINT ( 'NONE',  ( 11.09567578556706025, -9.260623346590088900, -60.14574966503957398 ) ) ;
#74609=ADVANCED_FACE ( 'NONE', ( #191225, #84028 ), #174073, .F. ) ;
#74610=DIRECTION ( 'NONE',  ( -0.000000000000000000, -0.000000000000000000, 1.000000000000000000 ) ) ;
#74614=CARTESIAN_POINT ( 'NONE',  ( 29.86685920354754487, 21.69954338932564752, -1.924999997268813212 ) ) ;
#74627=DIRECTION ( 'NONE',  ( 1.908195823574487804E-15, 0.000000000000000000, -1.000000000000000000 ) ) ;
#74632=B_SPLINE_CURVE_WITH_KNOTS ( 'NONE', 3,
 ( #45750, #33562, #17401, #153918, #79058, #95224, #168096, #60904, #29594, #156910, #2220, #223, #18407, #136759, #59916, #183279, #169075, #122579, #184268, #107402, #144708, #142717, #96214, #174077, #84030, #100205 ),
 .UNSPECIFIED., .F., .F.,
 ( 4, 2, 2, 2, 2, 2, 2, 2, 2, 2, 2, 2, 4 ),
 ( 8.673617379884035472E-19, 0.002268141957793348533, 0.004536283915586696198, 0.006804425873380042997, 0.009072567831173390662, 0.01360885174676007212, 0.01814513566234675704, 0.02268141957793343502, 0.02721770349352011995, 0.02948584545131345894, 0.03175398740910680140, 0.03402212936690014039, 0.03629027132469347938 ),
 .UNSPECIFIED. ) ;
#74662=ORIENTED_EDGE ( 'NONE', *, *, #53692, .F. ) ;
#74665=CARTESIAN_POINT ( 'NONE',  ( -36.91746825000000598, -11.99521256947794789, -11.02499999726881263 ) ) ;
#74669=CARTESIAN_POINT ( 'NONE',  ( 1.500000000000345945, 22.97976134357531564, -57.70670369762110141 ) ) ;
#74674=CARTESIAN_POINT ( 'NONE',  ( 31.88558403383513706, -20.67508902814666882, -24.22575984094845936 ) ) ;
#74687=CARTESIAN_POINT ( 'NONE',  ( -25.95926362436877710, -29.82107321766972774, -18.67624575278512822 ) ) ;
#74707=ADVANCED_FACE ( 'NONE', ( #193229 ), #97189, .F. ) ;
#74774=LINE ( 'NONE', #136436, #186190 ) ;
#74818=CARTESIAN_POINT ( 'NONE',  ( 1.499999999999986677, 30.24381343224601437, -47.95930528970760776 ) ) ;
#74822=ADVANCED_FACE ( 'NONE', ( #67870 ), #52699, .F. ) ;
#74853=VERTEX_POINT ( 'NONE', #42545 ) ;
#74855=CARTESIAN_POINT ( 'NONE',  ( -7.989781499195968806, 1.461410587780254788, -62.12232043736380405 ) ) ;
#74887=VERTEX_POINT ( 'NONE', #137517 ) ;
#74939=VERTEX_POINT ( 'NONE', #182051 ) ;
#74970=VERTEX_POINT ( 'NONE', #43534 ) ;
#75000=CARTESIAN_POINT ( 'NONE',  ( -6.020228577223754586E-15, 39.95556452105416412, -4.249999994537626336 ) ) ;
#75006=CARTESIAN_POINT ( 'NONE',  ( -7.990187535671161356, 1.461319442807373692, -64.16708268805474802 ) ) ;
#75055=ORIENTED_EDGE ( 'NONE', *, *, #16747, .T. ) ;
#75058=EDGE_LOOP ( 'NONE', ( #177831, #121549, #75297, #198654 ) ) ;
#75085=( BOUNDED_CURVE ( )  B_SPLINE_CURVE ( 2, ( #170633, #110935, #173623, #156455, #78604, #16950, #123119, #79607, #93779, #92778, #95766 ),
 .UNSPECIFIED., .F., .T. ) 
 B_SPLINE_CURVE_WITH_KNOTS ( ( 3, 2, 2, 2, 2, 3 ),
 ( 0.8000000000000000444, 0.8199999999999999512, 0.8399999999999999689, 0.8599999999999999867, 0.8800000000000000044, 0.9000000000000000222 ),
 .UNSPECIFIED. ) 
 CURVE ( )  GEOMETRIC_REPRESENTATION_ITEM ( )  RATIONAL_B_SPLINE_CURVE ( ( 1.000000000000000000, 0.9510565162951535312, 1.000000000000000000, 0.9510565162951535312, 1.000000000000000000, 0.9510565162951535312, 1.000000000000000000, 0.9510565162951535312, 1.000000000000000000, 0.9510565162951535312, 1.000000000000000000 ) ) 
 REPRESENTATION_ITEM ( '' )  );
#75086=CARTESIAN_POINT ( 'NONE',  ( 0.000000000000000000, 0.000000000000000000, -60.44446360152740283 ) ) ;
#75097=CARTESIAN_POINT ( 'NONE',  ( -3.874011537017815421, -5.374011537017721274, -64.44758591613756948 ) ) ;
#75099=FACE_OUTER_BOUND ( 'NONE', #16606, .T. ) ;
#75115=CARTESIAN_POINT ( 'NONE',  ( 30.74264578624799782, 22.33583958711400541, -2.799999999999999822 ) ) ;
#75141=DIRECTION ( 'NONE',  ( 0.000000000000000000, -1.000000000000000000, 0.000000000000000000 ) ) ;
#75168=VERTEX_POINT ( 'NONE', #105199 ) ;
#75225=AXIS2_PLACEMENT_3D ( 'NONE', #133052, #162386, #42060 ) ;
#75249=CARTESIAN_POINT ( 'NONE',  ( 0.000000000000000000, 0.000000000000000000, -56.77278709839600879 ) ) ;
#75257=CARTESIAN_POINT ( 'NONE',  ( 15.06137443927350361, 15.06137443927346098, -56.46919128290398504 ) ) ;
#75267=AXIS2_PLACEMENT_3D ( 'NONE', #33435, #188125, #98051 ) ;
#75294=ORIENTED_EDGE ( 'NONE', *, *, #139940, .T. ) ;
#75297=ORIENTED_EDGE ( 'NONE', *, *, #45175, .F. ) ;
#75306=CARTESIAN_POINT ( 'NONE',  ( -24.21728366753307071, -29.00647930567809851, -20.95994360448459659 ) ) ;
#75346=CARTESIAN_POINT ( 'NONE',  ( 36.91746824999999177, 11.99521256947799230, -9.524999997268812635 ) ) ;
#75364=CARTESIAN_POINT ( 'NONE',  ( 14.29384609392659833, -37.08231061483255075, -29.62140346006600922 ) ) ;
#75398=ADVANCED_FACE ( 'NONE', ( #71873 ), #151708, .F. ) ;
#75504=B_SPLINE_CURVE_WITH_KNOTS ( 'NONE', 3,
 ( #161242, #127898, #69231, #82382, #22736, #142078, #19740, #130898, #36885, #95578, #173437, #98551, #160245, #84384, #143066, #146061, #175417, #3564, #21734, #81381, #113721, #192588, #83387, #66238, #144070, #145064, #189600, #51073 ),
 .UNSPECIFIED., .F., .F.,
 ( 4, 2, 2, 2, 2, 2, 2, 2, 2, 2, 2, 2, 2, 4 ),
 ( 1.961533959443023196E-07, 0.0003775868847194836678, 0.0007549776160430232263, 0.001132368347366562514, 0.001509759078690102235, 0.002264540541337181027, 0.003019322003984260035, 0.003774103466631338610, 0.004151494197954877681, 0.004528884929278417619, 0.004906275660601956690, 0.005283666391925495760, 0.005661057123249034831, 0.006038447854572573902 ),
 .UNSPECIFIED. ) ;
#75552=CARTESIAN_POINT ( 'NONE',  ( -8.388830574159379737E-16, -13.70000000000001528, -62.58071313852362039 ) ) ;
#75569=CARTESIAN_POINT ( 'NONE',  ( -20.43538597629128262, 20.43538597629122222, -49.67367017693150189 ) ) ;
#75575=CARTESIAN_POINT ( 'NONE',  ( -20.29787683430801692, -22.40769709776935059, -48.02032541638636332 ) ) ;
#75582=ORIENTED_EDGE ( 'NONE', *, *, #26705, .T. ) ;
#75584=ORIENTED_EDGE ( 'NONE', *, *, #165816, .T. ) ;
#75590=CARTESIAN_POINT ( 'NONE',  ( -5.950531402560715689E-15, 38.81732327939063509, -1.624999997268813612 ) ) ;
#75613=CARTESIAN_POINT ( 'NONE',  ( 4.000000000000000888, -105.0000000000000000, 12.00000000000000355 ) ) ;
#75622=AXIS2_PLACEMENT_3D ( 'NONE', #179725, #167287, #28784 ) ;
#75628=EDGE_CURVE ( 'NONE', #39588, #92192, #167865, .T. ) ;
#75640=CARTESIAN_POINT ( 'NONE',  ( -11.40812507854755609, 35.11059874428196537, -9.524999997268816188 ) ) ;
#75648=CARTESIAN_POINT ( 'NONE',  ( 29.94898851760540026, -23.39111959325554935, -18.65171477573349179 ) ) ;
#75682=CARTESIAN_POINT ( 'NONE',  ( -16.70000000000002061, 1.759457951533292443E-13, -61.34707691135562868 ) ) ;
#75693=DIRECTION ( 'NONE',  ( -0.8660254037844391517, 0.000000000000000000, 0.4999999999999989453 ) ) ;
#75709=ORIENTED_EDGE ( 'NONE', *, *, #49944, .T. ) ;
#75728=AXIS2_PLACEMENT_3D ( 'NONE', #30345, #153681, #77827 ) ;
#75763=CIRCLE ( 'NONE', #82080, 12.50000000000000000 ) ;
#75791=CARTESIAN_POINT ( 'NONE',  ( 1.475613392205543661, 30.08492190595072557, -48.16867494856833787 ) ) ;
#75829=CARTESIAN_POINT ( 'NONE',  ( -8.898623008803063783, 0.7571601631682653988, -61.93576936796790022 ) ) ;
#75853=FACE_OUTER_BOUND ( 'NONE', #63188, .T. ) ;
#75859=CARTESIAN_POINT ( 'NONE',  ( 9.100000000000004974, -0.1000365528946606797, -63.95112321872119310 ) ) ;
#75864=ORIENTED_EDGE ( 'NONE', *, *, #69149, .T. ) ;
#75884=DIRECTION ( 'NONE',  ( 1.000000000000000000, 0.000000000000000000, 0.000000000000000000 ) ) ;
#75897=( BOUNDED_CURVE ( )  B_SPLINE_CURVE ( 2, ( #62448, #47308, #170644, #155470, #93790 ),
 .UNSPECIFIED., .F., .F. ) 
 B_SPLINE_CURVE_WITH_KNOTS ( ( 3, 2, 3 ),
 ( 0.9744993486534860860, 0.9799999999999999822, 1.000000000000000000 ),
 .UNSPECIFIED. ) 
 CURVE ( )  GEOMETRIC_REPRESENTATION_ITEM ( )  RATIONAL_B_SPLINE_CURVE ( ( 0.9804823514139775487, 0.9865389480227928498, 1.000000000000000000, 0.9510565162951535312, 1.000000000000000000 ) ) 
 REPRESENTATION_ITEM ( '' )  );
#75944=AXIS2_PLACEMENT_3D ( 'NONE', #126521, #62858, #173047 ) ;
#75951=CARTESIAN_POINT ( 'NONE',  ( 22.83054850305942907, -22.20849125555281489, -49.19912570997622936 ) ) ;
#75962=EDGE_CURVE ( 'NONE', #99310, #57684, #2693, .T. ) ;
#75967=CARTESIAN_POINT ( 'NONE',  ( 24.30000000000003268, 0.000000000000000000, -56.77278709839600879 ) ) ;
#76002=AXIS2_PLACEMENT_3D ( 'NONE', #13037, #188593, #182880 ) ;
#76040=ORIENTED_EDGE ( 'NONE', *, *, #115218, .T. ) ;
#76043=VERTEX_POINT ( 'NONE', #95981 ) ;
#76045=ORIENTED_EDGE ( 'NONE', *, *, #63738, .F. ) ;
#76047=CARTESIAN_POINT ( 'NONE',  ( -23.48529157249600985, 32.32473071737754111, -8.049999994537627046 ) ) ;
#76070=DIRECTION ( 'NONE',  ( -1.000000000000000000, 0.000000000000000000, 0.000000000000000000 ) ) ;
#76088=AXIS2_PLACEMENT_3D ( 'NONE', #43928, #105590, #153073 ) ;
#76091=CARTESIAN_POINT ( 'NONE',  ( -15.13939621930183854, 14.98335265924511717, -58.85720012050611416 ) ) ;
#76100=CARTESIAN_POINT ( 'NONE',  ( 11.74264578624799427, 36.14014761921585972, -2.600000000000000533 ) ) ;
#76105=DIRECTION ( 'NONE',  ( -0.000000000000000000, -0.000000000000000000, 1.000000000000000000 ) ) ;
#76125=CARTESIAN_POINT ( 'NONE',  ( 22.55660001725822994, -30.45235066353972542, -22.16622550485903886 ) ) ;
#76158=VERTEX_POINT ( 'NONE', #128295 ) ;
#76186=CIRCLE ( 'NONE', #14869, 38.00000000000000000 ) ;
#76193=CARTESIAN_POINT ( 'NONE',  ( 0.000000000000000000, 0.000000000000000000, -63.95112321872120731 ) ) ;
#76238=AXIS2_PLACEMENT_3D ( 'NONE', #8473, #162150, #131818 ) ;
#76241=CARTESIAN_POINT ( 'NONE',  ( -21.02754888379051934, -22.92766777125494215, -50.14365614045077990 ) ) ;
#76278=ORIENTED_EDGE ( 'NONE', *, *, #125471, .T. ) ;
#76288=EDGE_CURVE ( 'NONE', #112813, #139989, #115137, .T. ) ;
#76293=CARTESIAN_POINT ( 'NONE',  ( -22.27567441218681665, -30.36413145305472483, -19.29304740691864950 ) ) ;
#76299=ORIENTED_EDGE ( 'NONE', *, *, #9338, .F. ) ;
#76316=CARTESIAN_POINT ( 'NONE',  ( 22.02260766363856348, -20.08456848261498351, -48.57241000235018191 ) ) ;
#76319=LINE ( 'NONE', #184508, #14545 ) ;
#76322=EDGE_CURVE ( 'NONE', #189816, #36546, #54467, .T. ) ;
#76331=ORIENTED_EDGE ( 'NONE', *, *, #135199, .T. ) ;
#76335=ADVANCED_FACE ( 'NONE', ( #83783 ), #116137, .F. ) ;
#76336=CARTESIAN_POINT ( 'NONE',  ( 11.40812507854755253, -35.11059874428192273, -6.024999997268814411 ) ) ;
#76347=LINE ( 'NONE', #89541, #159202 ) ;
#76374=VERTEX_POINT ( 'NONE', #68623 ) ;
#76440=DIRECTION ( 'NONE',  ( 1.000000000000000000, 0.000000000000000000, 0.000000000000000000 ) ) ;
#76459=EDGE_CURVE ( 'NONE', #25627, #77120, #162638, .T. ) ;
#76565=CARTESIAN_POINT ( 'NONE',  ( 2.577820198429831642E-15, 9.100000000000001421, -61.89430850415821794 ) ) ;
#76568=FACE_BOUND ( 'NONE', #127324, .T. ) ;
#76574=FACE_OUTER_BOUND ( 'NONE', #96794, .T. ) ;
#76581=EDGE_LOOP ( 'NONE', ( #72465, #172106, #192282, #96783 ) ) ;
#76589=CARTESIAN_POINT ( 'NONE',  ( -30.74264578624800492, -22.33583958711396278, -11.54999999453762527 ) ) ;
#76601=CARTESIAN_POINT ( 'NONE',  ( 4.176031345420748941, 6.297279900606364222, -62.24169944404282973 ) ) ;
#76611=CARTESIAN_POINT ( 'NONE',  ( -24.11964846217544078, 0.7207009035789223583, -56.90195918390940477 ) ) ;
#76638=CARTESIAN_POINT ( 'NONE',  ( 1.468080482507219120, 23.15813577935543677, -57.58210375345692711 ) ) ;
#76644=CARTESIAN_POINT ( 'NONE',  ( 29.40087336786514527, -24.08182305020411462, -17.68713395559149859 ) ) ;
#76659=ORIENTED_EDGE ( 'NONE', *, *, #193305, .T. ) ;
#76696=EDGE_CURVE ( 'NONE', #150038, #123761, #24144, .T. ) ;
#76758=VECTOR ( 'NONE', #105484, 1000.000000000000000 ) ;
#76762=EDGE_CURVE ( 'NONE', #140047, #118127, #191974, .T. ) ;
#76787=CARTESIAN_POINT ( 'NONE',  ( -22.55670631985092456, 22.55670631985084995, -45.64921306006598201 ) ) ;
#76805=CARTESIAN_POINT ( 'NONE',  ( -5.000000000000000888, 11.45643923738960090, -15.00000000000000000 ) ) ;
#76824=CARTESIAN_POINT ( 'NONE',  ( -9.090072183657234461, 0.1985533113406500183, -61.89635373339110913 ) ) ;
#76859=EDGE_CURVE ( 'NONE', #171824, #124248, #192993, .T. ) ;
#76877=CARTESIAN_POINT ( 'NONE',  ( -5.773271879485258218, 3.915140329348332671, -64.38756054665735462 ) ) ;
#76889=ORIENTED_EDGE ( 'NONE', *, *, #184713, .T. ) ;
#76927=ADVANCED_FACE ( 'NONE', ( #190982 ), #20131, .F. ) ;
#76942=CARTESIAN_POINT ( 'NONE',  ( 11.45643923738959735, 5.000000000000007105, -18.00000000000000000 ) ) ;
#76948=ADVANCED_FACE ( 'NONE', ( #36285 ), #97941, .T. ) ;
#76957=CARTESIAN_POINT ( 'NONE',  ( 193.3062444957835453, -155.7167183371837496, -25.00000000000000000 ) ) ;
#76982=CARTESIAN_POINT ( 'NONE',  ( -9.100000000000001421, 9.789526074884739315E-14, -63.95112321872120731 ) ) ;
#77039=CARTESIAN_POINT ( 'NONE',  ( 11.74264578624799427, 36.14014761921585972, -8.349999994537625980 ) ) ;
#77075=CARTESIAN_POINT ( 'NONE',  ( -3.950025424479786551, -4.892422815249006796, -64.50280008989093972 ) ) ;
#77081=DIRECTION ( 'NONE',  ( 3.469446951953612217E-15, 0.000000000000000000, -1.000000000000000000 ) ) ;
#77086=CARTESIAN_POINT ( 'NONE',  ( -16.91340028822897068, 14.83455351965406877, -58.07447375877293894 ) ) ;
#77096=CARTESIAN_POINT ( 'NONE',  ( -6.020228577223754586E-15, 39.95556452105416412, -6.500000000000000000 ) ) ;
#77120=VERTEX_POINT ( 'NONE', #131300 ) ;
#77122=CARTESIAN_POINT ( 'NONE',  ( 8.963443992379767522, -45.12205215321816354, -22.08927284594079765 ) ) ;
#77127=ORIENTED_EDGE ( 'NONE', *, *, #195610, .T. ) ;
#77156=AXIS2_PLACEMENT_3D ( 'NONE', #72122, #27640, #59923 ) ;
#77186=CARTESIAN_POINT ( 'NONE',  ( 1.500000000000000888, 15.20000000000002061, -59.79525829764741474 ) ) ;
#77190=ADVANCED_FACE ( 'NONE', ( #192989 ), #100953, .F. ) ;
#77226=CARTESIAN_POINT ( 'NONE',  ( 0.000000000000000000, 0.000000000000000000, -15.00000000000000000 ) ) ;
#77236=CARTESIAN_POINT ( 'NONE',  ( 16.83259678516731839, 17.45991095687928762, -54.25516819912628108 ) ) ;
#77238=LINE ( 'NONE', #62059, #14282 ) ;
#77286=CARTESIAN_POINT ( 'NONE',  ( -7.213464565008907314, -38.12638803158534984, -24.00445952849389641 ) ) ;
#77311=CARTESIAN_POINT ( 'NONE',  ( 22.46875132164074884, -20.34737474481815056, -47.91687182510066378 ) ) ;
#77319=CARTESIAN_POINT ( 'NONE',  ( 21.71562642307798185, -20.00551537737228713, -51.98609762351841113 ) ) ;
#77349=CARTESIAN_POINT ( 'NONE',  ( 8.863853373469035901, -46.11448583660357770, -24.15755306339434227 ) ) ;
#77351=CARTESIAN_POINT ( 'NONE',  ( -11.30013253874036216, -12.15106144227211438, -61.39618700965100828 ) ) ;
#77392=FACE_OUTER_BOUND ( 'NONE', #169763, .T. ) ;
#77425=CARTESIAN_POINT ( 'NONE',  ( 1.500000000000163203, 15.29469527405681184, -61.93010668218706627 ) ) ;
#77441=DIRECTION ( 'NONE',  ( -9.445700745138859830E-17, 1.000000000000000000, 0.000000000000000000 ) ) ;
#77460=EDGE_CURVE ( 'NONE', #111025, #12839, #60708, .T. ) ;
#77511=EDGE_LOOP ( 'NONE', ( #37931, #59760, #132052, #84834 ) ) ;
#77566=CARTESIAN_POINT ( 'NONE',  ( 1.338944653035268662, 22.09907077859329405, -58.31495840562853061 ) ) ;
#77573=ORIENTED_EDGE ( 'NONE', *, *, #30682, .F. ) ;
#77581=CARTESIAN_POINT ( 'NONE',  ( 22.81625015709509441, 31.40387420917330275, -1.824999997268813567 ) ) ;
#77631=CARTESIAN_POINT ( 'NONE',  ( -11.40812507854754720, -35.11059874428192273, -10.72499999726881548 ) ) ;
#77704=VERTEX_POINT ( 'NONE', #70641 ) ;
#77756=CARTESIAN_POINT ( 'NONE',  ( 1.304798881014889833, 6.853701371036049039, -62.35416993336013292 ) ) ;
#77778=CARTESIAN_POINT ( 'NONE',  ( -22.65278057777883092, 22.46063206192296136, -45.64921306006598911 ) ) ;
#77780=CARTESIAN_POINT ( 'NONE',  ( 20.43538597629129328, 20.43538597629121156, -49.67367017693150189 ) ) ;
#77789=ORIENTED_EDGE ( 'NONE', *, *, #47276, .T. ) ;
#77825=CARTESIAN_POINT ( 'NONE',  ( 21.39352396646988552, -0.5319302666794151202, -58.79417398750191381 ) ) ;
#77827=DIRECTION ( 'NONE',  ( 1.000000000000000000, 0.000000000000000000, 0.000000000000000000 ) ) ;
#77874=CARTESIAN_POINT ( 'NONE',  ( -25.83521962401025007, -30.44105770729785121, -17.07601944841967523 ) ) ;
#77879=FACE_OUTER_BOUND ( 'NONE', #27253, .T. ) ;
#77880=CYLINDRICAL_SURFACE ( 'NONE', #115449, 12.50000000000000000 ) ;
#77897=EDGE_CURVE ( 'NONE', #119352, #182346, #115620, .T. ) ;
#77913=CARTESIAN_POINT ( 'NONE',  ( -0.3920586954752057207, -9.051216217265922737, -61.90435651123959104 ) ) ;
#78060=CARTESIAN_POINT ( 'NONE',  ( -4.243048740927896745, -4.383653989548000673, -64.53213882399991519 ) ) ;
#78065=CARTESIAN_POINT ( 'NONE',  ( 17.18269478283316332, -17.18269478283309226, -56.77278709839600879 ) ) ;
#78070=CARTESIAN_POINT ( 'NONE',  ( -17.49235657833709467, 16.74109322108048659, -56.83968056806632774 ) ) ;
#78081=AXIS2_PLACEMENT_3D ( 'NONE', #84102, #161958, #23454 ) ;
#78105=CARTESIAN_POINT ( 'NONE',  ( 8.122171662651544111, -45.80197342711153397, -22.32604245071861371 ) ) ;
#78149=CYLINDRICAL_SURFACE ( 'NONE', #85491, 1.499999999999997780 ) ;
#78173=CARTESIAN_POINT ( 'NONE',  ( 7.503800738396989800, -1.500046863536464992, -62.22166870076608092 ) ) ;
#78192=DIRECTION ( 'NONE',  ( -0.000000000000000000, -0.000000000000000000, 1.000000000000000000 ) ) ;
#78228=EDGE_CURVE ( 'NONE', #39558, #121632, #195771, .T. ) ;
#78263=EDGE_CURVE ( 'NONE', #194207, #28673, #164231, .T. ) ;
#78269=CARTESIAN_POINT ( 'NONE',  ( -23.37981185087361524, -29.75599608462389156, -21.51565039292586690 ) ) ;
#78294=CARTESIAN_POINT ( 'NONE',  ( 3.920520744267807167, 4.990514878257738651, -64.49346902751020139 ) ) ;
#78302=EDGE_CURVE ( 'NONE', #45716, #59419, #140254, .T. ) ;
#78309=DIRECTION ( 'NONE',  ( 0.000000000000000000, 0.000000000000000000, 1.000000000000000000 ) ) ;
#78319=DIRECTION ( 'NONE',  ( 1.000000000000000000, 0.000000000000000000, 0.000000000000000000 ) ) ;
#78327=CARTESIAN_POINT ( 'NONE',  ( 6.434671708797603529, -6.434671708797564449, -64.92279855667830191 ) ) ;
#78329=CARTESIAN_POINT ( 'NONE',  ( 22.88436389169569196, -32.73361847831127847, -22.76175135428369956 ) ) ;
#78386=CARTESIAN_POINT ( 'NONE',  ( 37.99999999999999289, 2.893978650043524126E-14, -3.000000000000000000 ) ) ;
#78412=DIRECTION ( 'NONE',  ( -0.000000000000000000, 0.000000000000000000, 1.000000000000000000 ) ) ;
#78418=AXIS2_PLACEMENT_3D ( 'NONE', #23733, #85382, #8559 ) ;
#78423=EDGE_CURVE ( 'NONE', #16157, #41521, #57480, .T. ) ;
#78446=ORIENTED_EDGE ( 'NONE', *, *, #100204, .F. ) ;
#78474=B_SPLINE_CURVE_WITH_KNOTS ( 'NONE', 3,
 ( #152929, #76091, #46762, #93240, #3228, #45764, #15427, #79070, #61904, #169089, #156922, #77086, #170096, #154925, #138755, #123575, #94237, #124586, #139738, #78070, #108421, #16423, #1227, #62905 ),
 .UNSPECIFIED., .F., .F.,
 ( 4, 2, 2, 2, 2, 2, 2, 2, 2, 2, 2, 4 ),
 ( 2.784816138783909714E-07, 0.0003261688173017302525, 0.0006520591529895821293, 0.0009779494886774341145, 0.001303839824365285883, 0.001955620495740971205, 0.002607401167116656527, 0.003259181838492341415, 0.003910962509868023268, 0.004562743181243703386, 0.004888633516931540843, 0.005214523852619376565 ),
 .UNSPECIFIED. ) ;
#78550=CARTESIAN_POINT ( 'NONE',  ( 12.24802307403557577, -10.74802307403608737, -59.32879157176802920 ) ) ;
#78557=ORIENTED_EDGE ( 'NONE', *, *, #40630, .F. ) ;
#78560=ORIENTED_EDGE ( 'NONE', *, *, #150015, .F. ) ;
#78563=CARTESIAN_POINT ( 'NONE',  ( -6.434671708797603529, 6.434671708797564449, -61.89430850415821794 ) ) ;
#78567=CARTESIAN_POINT ( 'NONE',  ( -36.91746825000001309, 11.99521256947798342, -3.224999997268813257 ) ) ;
#78580=CARTESIAN_POINT ( 'NONE',  ( 4.023452810412280201, 4.713873842512024126, -62.49134662286012087 ) ) ;
#78604=CARTESIAN_POINT ( 'NONE',  ( -11.74264578624800670, 36.14014761921585972, -8.400000000000000355 ) ) ;
#78616=CARTESIAN_POINT ( 'NONE',  ( -36.91746825000000598, 2.428612866367529932E-14, -9.124999997268814056 ) ) ;
#78618=CARTESIAN_POINT ( 'NONE',  ( 29.86685920354754842, -21.69954338932559068, -4.324999997268814234 ) ) ;
#78627=CARTESIAN_POINT ( 'NONE',  ( -12.20200080651912344, 10.33258783678502546, -61.66593582935060880 ) ) ;
#78686=EDGE_LOOP ( 'NONE', ( #153966, #8599, #125621, #156957, #108188, #160994, #110425, #136810 ) ) ;
#78692=ORIENTED_EDGE ( 'NONE', *, *, #151524, .T. ) ;
#78745=CARTESIAN_POINT ( 'NONE',  ( 3.735172737399431091E-16, 6.100000000000006750, -62.50719930893269805 ) ) ;
#78764=CARTESIAN_POINT ( 'NONE',  ( 193.3062444957835453, -155.7167183371837496, -25.00000000000000000 ) ) ;
#78768=CARTESIAN_POINT ( 'NONE',  ( -22.73357338108569081, 22.35296335725854533, -45.67722784712131556 ) ) ;
#78770=VECTOR ( 'NONE', #57495, 1000.000000000000000 ) ;
#78795=AXIS2_PLACEMENT_3D ( 'NONE', #99481, #161162, #163166 ) ;
#78806=LINE ( 'NONE', #189980, #166578 ) ;
#78808=CARTESIAN_POINT ( 'NONE',  ( -6.293264767923588465, 0.7627558185761745824, -62.46802126132831035 ) ) ;
#78854=DIRECTION ( 'NONE',  ( -0.000000000000000000, -0.000000000000000000, 1.000000000000000000 ) ) ;
#78864=CARTESIAN_POINT ( 'NONE',  ( -5.000000000000000000, 11.45643923738959913, -18.00000000000000000 ) ) ;
#78872=ORIENTED_EDGE ( 'NONE', *, *, #23760, .F. ) ;
#78894=LINE ( 'NONE', #126399, #113583 ) ;
#78905=CARTESIAN_POINT ( 'NONE',  ( -15.66706267174403067, 1.428615351859272575, -61.77652290643390387 ) ) ;
#78926=DIRECTION ( 'NONE',  ( 0.000000000000000000, 0.000000000000000000, 1.000000000000000000 ) ) ;
#78987=CIRCLE ( 'NONE', #36990, 2.500000000000000000 ) ;
#79043=AXIS2_PLACEMENT_3D ( 'NONE', #77226, #121740, #170238 ) ;
#79047=CARTESIAN_POINT ( 'NONE',  ( 37.99999999999999289, 2.893978650043524126E-14, -5.000000000000000000 ) ) ;
#79058=CARTESIAN_POINT ( 'NONE',  ( 6.918342302711550040, -47.27039221922507295, -24.65254351866712668 ) ) ;
#79059=DIRECTION ( 'NONE',  ( 1.000000000000000000, 0.000000000000000000, 0.000000000000000000 ) ) ;
#79065=CARTESIAN_POINT ( 'NONE',  ( -11.30153831258470731, -190.0000000000000000, -25.00000000000000000 ) ) ;
#79070=CARTESIAN_POINT ( 'NONE',  ( -16.00195535827013771, 14.62341493535840264, -58.61703605924742533 ) ) ;
#79103=CARTESIAN_POINT ( 'NONE',  ( 23.38845648566366364, -29.41134498177906309, -18.89001425235115406 ) ) ;
#79107=ORIENTED_EDGE ( 'NONE', *, *, #55941, .T. ) ;
#79129=VECTOR ( 'NONE', #60012, 1000.000000000000000 ) ;
#79131=ORIENTED_EDGE ( 'NONE', *, *, #749, .F. ) ;
#79171=CARTESIAN_POINT ( 'NONE',  ( -3.874011537017815865, -5.374011537017721274, -64.92279855667830191 ) ) ;
#79174=CARTESIAN_POINT ( 'NONE',  ( 7.989781499195996339, -1.461410587780195947, -62.12232043736379694 ) ) ;
#79195=DIRECTION ( 'NONE',  ( 0.000000000000000000, 0.000000000000000000, 1.000000000000000000 ) ) ;
#79221=CARTESIAN_POINT ( 'NONE',  ( 9.262594875851847931, 10.97788116290291249, -60.18097545586278585 ) ) ;
#79259=ORIENTED_EDGE ( 'NONE', *, *, #60885, .F. ) ;
#79266=AXIS2_PLACEMENT_3D ( 'NONE', #118793, #197617, #90413 ) ;
#79274=EDGE_CURVE ( 'NONE', #41082, #151987, #107053, .T. ) ;
#79276=CARTESIAN_POINT ( 'NONE',  ( -36.30973463498060738, -18.33876584755894612, -18.81039752656815622 ) ) ;
#79299=CARTESIAN_POINT ( 'NONE',  ( 21.75275980508837392, -20.01158182446510736, -48.88299994772790313 ) ) ;
#79325=CARTESIAN_POINT ( 'NONE',  ( 11.40812507854754365, 35.11059874428196537, -5.224999997268813701 ) ) ;
#79333=DIRECTION ( 'NONE',  ( -1.000000000000000000, 3.552713678800500929E-15, 0.000000000000000000 ) ) ;
#79335=CARTESIAN_POINT ( 'NONE',  ( 24.03200911576290366, -31.81637637394766571, -21.77892875004970819 ) ) ;
#79389=CARTESIAN_POINT ( 'NONE',  ( -36.91746825000001309, 11.99521256947798342, -2.724999997268813701 ) ) ;
#79415=CARTESIAN_POINT ( 'NONE',  ( -28.47622644277399928, -25.16156846422451920, -16.68312038616162951 ) ) ;
#79453=ORIENTED_EDGE ( 'NONE', *, *, #192121, .F. ) ;
#79454=( BOUNDED_SURFACE ( )  B_SPLINE_SURFACE ( 1, 2, ( 
 ( #67137, #65146, #128795, #189504, #139992, #51967, #1481, #97447, #50979, #98453, #142971, #4448, #124838, #95482, #187532, #96466, #158154, #113626, #143974, #82282, #66138, #110653, #80308, #19646, #112639, #173339, #109667, #126803, #141981, #171347, #188511, #127801, #34811, #2483, #81287, #36787, #175321, #160146, #21637, #5454, #63159, #174331, #35801, #3469, #49988, #48997, #79325, #48011, #159133, #20630, #186538, #32836, #94486, #156168, #17667, #172333, #125829, #140995, #64164, #33822, #157168, #18662, #117645, #164162, #132809, #10478, #54971, #55968, #176330, #52955, #8468, #53974, #163149, #72138, #86301, #39794, #192491, #148988, #115647, #177337, #194495, #40805, #102475, #25660, #87305, #147990, #22640, #70142, #179342, #9479, #133814, #195505, #118652, #38808, #56978, #83291, #162145, #129780, #191477, #180343, #7448 ),
 ( #100466, #161143, #41811, #116641, #103479, #165157, #37800, #69132, #68129, #114631, #131813, #144967, #84287, #23641, #6448, #99463, #24652, #145966, #178331, #193492, #130800, #101458, #85289, #146981, #71143, #44785, #76100, #150989, #75115, #73157, #29615, #106438, #58951, #168119, #169098, #137775, #13451, #107426, #12481, #166156, #88292, #74142, #91247, #183303, #182315, #123585, #89297, #135814, #181330, #61914, #136783, #152938, #121608, #198469, #184292, #26649, #59940, #199461, #60928, #197484, #14437, #120619, #122602, #185279, #28643, #77096, #43795, #45773, #30605, #119648, #92258, #46771, #105458, #153942, #15437, #90279, #138765, #167144, #246, #108430, #149980, #151963, #11486, #134827, #196506, #57976, #42809, #104471, #27657, #188273, #128559, #48761, #172097, #186290, #66896, #35567, #18428, #16432, #97215, #125593, #112406 ) ),
 .UNSPECIFIED., .F., .F., .F. ) 
 B_SPLINE_SURFACE_WITH_KNOTS ( ( 2, 2 ),
 ( 3, 2, 2, 2, 2, 2, 2, 2, 2, 2, 2, 2, 2, 2, 2, 2, 2, 2, 2, 2, 2, 2, 2, 2, 2, 2, 2, 2, 2, 2, 2, 2, 2, 2, 2, 2, 2, 2, 2, 2, 2, 2, 2, 2, 2, 2, 2, 2, 2, 2, 3 ),
 ( 0.000000000000000000, 1.000000000000000000 ),
 ( 0.000000000000000000, 0.02000000000000000042, 0.04000000000000000083, 0.05999999999999999778, 0.08000000000000000167, 0.1000000000000000056, 0.1199999999999999956, 0.1400000000000000133, 0.1600000000000000033, 0.1799999999999999933, 0.2000000000000000111, 0.2200000000000000011, 0.2399999999999999911, 0.2600000000000000089, 0.2800000000000000266, 0.2999999999999999889, 0.3200000000000000067, 0.3400000000000000244, 0.3599999999999999867, 0.3800000000000000044, 0.4000000000000000222, 0.4199999999999999845, 0.4400000000000000022, 0.4600000000000000200, 0.4799999999999999822, 0.5000000000000000000, 0.5200000000000000178, 0.5400000000000000355, 0.5600000000000000533, 0.5799999999999999600, 0.5999999999999999778, 0.6199999999999999956, 0.6400000000000000133, 0.6600000000000000311, 0.6800000000000000488, 0.6999999999999999556, 0.7199999999999999734, 0.7399999999999999911, 0.7600000000000000089, 0.7800000000000000266, 0.8000000000000000444, 0.8199999999999999512, 0.8399999999999999689, 0.8599999999999999867, 0.8800000000000000044, 0.9000000000000000222, 0.9200000000000000400, 0.9399999999999999467, 0.9599999999999999645, 0.9799999999999999822, 1.000000000000000000 ),
 .UNSPECIFIED. ) 
 GEOMETRIC_REPRESENTATION_ITEM ( )  RATIONAL_B_SPLINE_SURFACE ( (
 ( 1.000000000000000000, 0.9510565162951535312, 1.000000000000000000, 0.9510565162951535312, 1.000000000000000000, 0.9510565162951535312, 1.000000000000000000, 0.9510565162951535312, 1.000000000000000000, 0.9510565162951535312, 1.000000000000000000, 0.9510565162951535312, 1.000000000000000000, 0.9510565162951535312, 1.000000000000000000, 0.9510565162951535312, 1.000000000000000000, 0.9510565162951535312, 1.000000000000000000, 0.9510565162951535312, 1.000000000000000000, 0.9510565162951535312, 1.000000000000000000, 0.9510565162951535312, 1.000000000000000000, 0.9510565162951535312, 1.000000000000000000, 0.9510565162951535312, 1.000000000000000000, 0.9510565162951535312, 1.000000000000000000, 0.9510565162951535312, 1.000000000000000000, 0.9510565162951535312, 1.000000000000000000, 0.9510565162951535312, 1.000000000000000000, 0.9510565162951535312, 1.000000000000000000, 0.9510565162951535312, 1.000000000000000000, 0.9510565162951535312, 1.000000000000000000, 0.9510565162951535312, 1.000000000000000000, 0.9510565162951535312, 1.000000000000000000, 0.9510565162951535312, 1.000000000000000000, 0.9510565162951535312, 1.000000000000000000, 0.9510565162951535312, 1.000000000000000000, 0.9510565162951535312, 1.000000000000000000, 0.9510565162951535312, 1.000000000000000000, 0.9510565162951535312, 1.000000000000000000, 0.9510565162951535312, 1.000000000000000000, 0.9510565162951535312, 1.000000000000000000, 0.9510565162951535312, 1.000000000000000000, 0.9510565162951535312, 1.000000000000000000, 0.9510565162951535312, 1.000000000000000000, 0.9510565162951535312, 1.000000000000000000, 0.9510565162951535312, 1.000000000000000000, 0.9510565162951535312, 1.000000000000000000, 0.9510565162951535312, 1.000000000000000000, 0.9510565162951535312, 1.000000000000000000, 0.9510565162951535312, 1.000000000000000000, 0.9510565162951535312, 1.000000000000000000, 0.9510565162951535312, 1.000000000000000000, 0.9510565162951535312, 1.000000000000000000, 0.9510565162951535312, 1.000000000000000000, 0.9510565162951535312, 1.000000000000000000, 0.9510565162951535312, 1.000000000000000000, 0.9510565162951535312, 1.000000000000000000, 0.9510565162951535312, 1.000000000000000000, 0.9510565162951535312, 1.000000000000000000, 0.9510565162951535312, 1.000000000000000000),
 ( 1.000000000000000000, 0.9510565162951535312, 1.000000000000000000, 0.9510565162951535312, 1.000000000000000000, 0.9510565162951535312, 1.000000000000000000, 0.9510565162951535312, 1.000000000000000000, 0.9510565162951535312, 1.000000000000000000, 0.9510565162951535312, 1.000000000000000000, 0.9510565162951535312, 1.000000000000000000, 0.9510565162951535312, 1.000000000000000000, 0.9510565162951535312, 1.000000000000000000, 0.9510565162951535312, 1.000000000000000000, 0.9510565162951535312, 1.000000000000000000, 0.9510565162951535312, 1.000000000000000000, 0.9510565162951535312, 1.000000000000000000, 0.9510565162951535312, 1.000000000000000000, 0.9510565162951535312, 1.000000000000000000, 0.9510565162951535312, 1.000000000000000000, 0.9510565162951535312, 1.000000000000000000, 0.9510565162951535312, 1.000000000000000000, 0.9510565162951535312, 1.000000000000000000, 0.9510565162951535312, 1.000000000000000000, 0.9510565162951535312, 1.000000000000000000, 0.9510565162951535312, 1.000000000000000000, 0.9510565162951535312, 1.000000000000000000, 0.9510565162951535312, 1.000000000000000000, 0.9510565162951535312, 1.000000000000000000, 0.9510565162951535312, 1.000000000000000000, 0.9510565162951535312, 1.000000000000000000, 0.9510565162951535312, 1.000000000000000000, 0.9510565162951535312, 1.000000000000000000, 0.9510565162951535312, 1.000000000000000000, 0.9510565162951535312, 1.000000000000000000, 0.9510565162951535312, 1.000000000000000000, 0.9510565162951535312, 1.000000000000000000, 0.9510565162951535312, 1.000000000000000000, 0.9510565162951535312, 1.000000000000000000, 0.9510565162951535312, 1.000000000000000000, 0.9510565162951535312, 1.000000000000000000, 0.9510565162951535312, 1.000000000000000000, 0.9510565162951535312, 1.000000000000000000, 0.9510565162951535312, 1.000000000000000000, 0.9510565162951535312, 1.000000000000000000, 0.9510565162951535312, 1.000000000000000000, 0.9510565162951535312, 1.000000000000000000, 0.9510565162951535312, 1.000000000000000000, 0.9510565162951535312, 1.000000000000000000, 0.9510565162951535312, 1.000000000000000000, 0.9510565162951535312, 1.000000000000000000, 0.9510565162951535312, 1.000000000000000000, 0.9510565162951535312, 1.000000000000000000, 0.9510565162951535312, 1.000000000000000000) ) ) 
 REPRESENTATION_ITEM ( '' )  SURFACE ( )  );
#79470=AXIS2_PLACEMENT_3D ( 'NONE', #92592, #126900, #15771 ) ;
#79473=EDGE_CURVE ( 'NONE', #71451, #194525, #125223, .T. ) ;
#79482=CARTESIAN_POINT ( 'NONE',  ( -38.00000000000000711, 2.428612866367529932E-14, 0.000000000000000000 ) ) ;
#79558=DIRECTION ( 'NONE',  ( -0.000000000000000000, -0.000000000000000000, 1.000000000000000000 ) ) ;
#79561=AXIS2_PLACEMENT_3D ( 'NONE', #19423, #81070, #20402 ) ;
#79607=CARTESIAN_POINT ( 'NONE',  ( 23.48529157249599564, 32.32473071737754111, -8.700000000000002842 ) ) ;
#79617=EDGE_CURVE ( 'NONE', #40993, #179372, #49375, .T. ) ;
#79619=LINE ( 'NONE', #81575, #25293 ) ;
#79622=CARTESIAN_POINT ( 'NONE',  ( -29.86685920354755552, 21.69954338932564397, -3.324999997268813345 ) ) ;
#79623=CARTESIAN_POINT ( 'NONE',  ( -22.64734518408119612, 22.46606745562059970, -49.13275782002548198 ) ) ;
#79630=CARTESIAN_POINT ( 'NONE',  ( -11.42987701755558128, 9.408549014593454274, -62.15975709196302290 ) ) ;
#79691=ORIENTED_EDGE ( 'NONE', *, *, #156319, .F. ) ;
#79704=AXIS2_PLACEMENT_3D ( 'NONE', #160679, #37331, #100993 ) ;
#79776=CARTESIAN_POINT ( 'NONE',  ( -21.53159096656795768, 0.8285391498305729741, -56.30101842015761804 ) ) ;
#79799=CIRCLE ( 'NONE', #186482, 38.00000000000000000 ) ;
#79814=CARTESIAN_POINT ( 'NONE',  ( 23.48529157249599919, 32.32473071737754111, -2.449999994537626069 ) ) ;
#79825=ADVANCED_FACE ( 'NONE', ( #127187 ), #129173, .F. ) ;
#79826=CARTESIAN_POINT ( 'NONE',  ( 31.73029476377072555, -20.92000799991017246, -24.48145274275710292 ) ) ;
#79842=VECTOR ( 'NONE', #41271, 1000.000000000000000 ) ;
#79880=ORIENTED_EDGE ( 'NONE', *, *, #75962, .F. ) ;
#79899=CARTESIAN_POINT ( 'NONE',  ( 37.99999999999999289, 2.893978650043524126E-14, -8.749999994537628112 ) ) ;
#79909=CARTESIAN_POINT ( 'NONE',  ( -1.314123079931730054, -8.348819774032584462, -62.04874212273343659 ) ) ;
#80035=CARTESIAN_POINT ( 'NONE',  ( 13.90353822939981931, -0.7813480796679665996, -62.49831333862085359 ) ) ;
#80101=CARTESIAN_POINT ( 'NONE',  ( 22.64239272338469178, -30.05593529206061021, -19.14955533182169845 ) ) ;
#80159=DIRECTION ( 'NONE',  ( 1.000000000000000000, 0.000000000000000000, 0.000000000000000000 ) ) ;
#80209=DIRECTION ( 'NONE',  ( 1.000000000000000000, 0.000000000000000000, 0.000000000000000000 ) ) ;
#80238=AXIS2_PLACEMENT_3D ( 'NONE', #71435, #23935, #118949 ) ;
#80278=DIRECTION ( 'NONE',  ( -0.000000000000000000, -0.000000000000000000, 1.000000000000000000 ) ) ;
#80283=CARTESIAN_POINT ( 'NONE',  ( -3.573655867282028392E-15, 2.428612866367529932E-14, -25.00000000000000000 ) ) ;
#80286=CARTESIAN_POINT ( 'NONE',  ( 3.874965782148156457, 5.576804854476206330, -64.41982836185009376 ) ) ;
#80308=CARTESIAN_POINT ( 'NONE',  ( -29.86685920354755552, 21.69954338932564397, -2.824999997268813345 ) ) ;
#80318=CARTESIAN_POINT ( 'NONE',  ( 25.90378602754583071, -30.37248848106526822, -17.06839622125441736 ) ) ;
#80366=DIRECTION ( 'NONE',  ( 0.000000000000000000, -0.000000000000000000, 1.000000000000000000 ) ) ;
#80370=CARTESIAN_POINT ( 'NONE',  ( 29.86685920354754842, -21.69954338932559068, -10.32499999726881335 ) ) ;
#80379=DIRECTION ( 'NONE',  ( 0.000000000000000000, 0.000000000000000000, 1.000000000000000000 ) ) ;
#80391=CARTESIAN_POINT ( 'NONE',  ( -0.2000799437544613923, -6.100000000000011191, -64.53213882399992940 ) ) ;
#80402=EDGE_CURVE ( 'NONE', #173153, #25217, #157618, .T. ) ;
#80406=CARTESIAN_POINT ( 'NONE',  ( -11.74264578624799782, -36.14014761921581709, -1.599999999999999867 ) ) ;
#80496=AXIS2_PLACEMENT_3D ( 'NONE', #141675, #81962, #108352 ) ;
#80533=CARTESIAN_POINT ( 'NONE',  ( 1.314372631020014115, 8.348397508521239629, -62.04882876100633382 ) ) ;
#80536=LINE ( 'NONE', #21866, #144485 ) ;
#80552=DIRECTION ( 'NONE',  ( -0.000000000000000000, -0.000000000000000000, 1.000000000000000000 ) ) ;
#80555=CARTESIAN_POINT ( 'NONE',  ( -36.91746825000001309, 11.99521256947798342, -9.224999997268813701 ) ) ;
#80563=DIRECTION ( 'NONE',  ( 1.000000000000000000, 0.000000000000000000, 0.000000000000000000 ) ) ;
#80604=CARTESIAN_POINT ( 'NONE',  ( -11.40812507854755609, 35.11059874428196537, -5.524999997268813523 ) ) ;
#80606=CIRCLE ( 'NONE', #3107, 24.30000000000003268 ) ;
#80613=CARTESIAN_POINT ( 'NONE',  ( 2.662494480112515660, -37.13692398601924793, -32.59999999999999432 ) ) ;
#80694=CARTESIAN_POINT ( 'NONE',  ( -1.227931366032057224E-14, -24.30000000000003268, -54.21489346206828230 ) ) ;
#80739=EDGE_CURVE ( 'NONE', #34342, #56776, #164654, .T. ) ;
#80753=DIRECTION ( 'NONE',  ( 1.000000000000000000, 5.372046893347532792E-15, 0.000000000000000000 ) ) ;
#80757=DIRECTION ( 'NONE',  ( 1.000000000000000000, 0.000000000000000000, 0.000000000000000000 ) ) ;
#80775=CARTESIAN_POINT ( 'NONE',  ( -31.90000000000002700, 0.1282610754047256441, -49.13275782002543934 ) ) ;
#80794=CARTESIAN_POINT ( 'NONE',  ( -23.48529157249599919, -32.32473071737750558, -3.449999994537626957 ) ) ;
#80804=CARTESIAN_POINT ( 'NONE',  ( 21.52594032250407352, -0.8193109935767731722, -58.70475745007095014 ) ) ;
#80862=CARTESIAN_POINT ( 'NONE',  ( -17.75813068129445327, -35.78296932995274204, -27.23805928211587002 ) ) ;
#80879=DIRECTION ( 'NONE',  ( -1.000000000000000000, 0.000000000000000000, 0.000000000000000000 ) ) ;
#80918=DIRECTION ( 'NONE',  ( 0.9930308165857338887, 0.1178549842436482642, 0.000000000000000000 ) ) ;
#80928=CARTESIAN_POINT ( 'NONE',  ( -3.962867913677101228, -5.961113794123787279, -62.32090908991690981 ) ) ;
#80939=EDGE_CURVE ( 'NONE', #45831, #29612, #180474, .T. ) ;
#80974=EDGE_CURVE ( 'NONE', #127568, #150038, #147962, .T. ) ;
#80998=B_SPLINE_CURVE_WITH_KNOTS ( 'NONE', 3,
 ( #16262, #97048, #156762, #77913, #1065, #63751, #124420, #187121, #32420, #96067, #79909, #158730, #20220, #141580, #111239, #142571, #143559, #5042, #123413, #70736, #8048, #86893, #191077, #117232, #102066, #162735 ),
 .UNSPECIFIED., .F., .F.,
 ( 4, 2, 2, 2, 2, 2, 2, 2, 2, 2, 2, 2, 4 ),
 ( 1.971390914159136004E-07, 0.0002963316798228975667, 0.0005924662205543791650, 0.0008886007612858607633, 0.001184735302017342470, 0.001777004383480305667, 0.002369273464943269080, 0.002665408005674750787, 0.002961542546406232494, 0.003257677087137714200, 0.003553811627869195473, 0.004146080709332164091, 0.004738349790795131841 ),
 .UNSPECIFIED. ) ;
#81009=ORIENTED_EDGE ( 'NONE', *, *, #85538, .F. ) ;
#81011=DIRECTION ( 'NONE',  ( -0.000000000000000000, -0.000000000000000000, 1.000000000000000000 ) ) ;
#81020=CARTESIAN_POINT ( 'NONE',  ( 15.57446157010957855, -1.455575599910922557, -61.81477736546833768 ) ) ;
#81059=ORIENTED_EDGE ( 'NONE', *, *, #105844, .T. ) ;
#81070=DIRECTION ( 'NONE',  ( -0.000000000000000000, -0.000000000000000000, 1.000000000000000000 ) ) ;
#81082=ADVANCED_FACE ( 'NONE', ( #147775 ), #9262, .T. ) ;
#81084=CARTESIAN_POINT ( 'NONE',  ( 24.94166821950292956, -28.00113106726958989, -18.51304999530601947 ) ) ;
#81108=ORIENTED_EDGE ( 'NONE', *, *, #119454, .T. ) ;
#81142=DIRECTION ( 'NONE',  ( -1.000000000000000000, 6.391086490440865492E-16, 0.000000000000000000 ) ) ;
#81241=CARTESIAN_POINT ( 'NONE',  ( -33.60028042027822437, -17.96933036163185449, -21.71044752825889290 ) ) ;
#81263=CARTESIAN_POINT ( 'NONE',  ( -29.34370184275724114, 1.069973119863280697, -49.12095057784389951 ) ) ;
#81266=CARTESIAN_POINT ( 'NONE',  ( 0.000000000000000000, 0.000000000000000000, -58.85720012050612837 ) ) ;
#81271=CARTESIAN_POINT ( 'NONE',  ( 6.874011537017776341, -5.570717421327670671, -64.00967186878696680 ) ) ;
#81287=CARTESIAN_POINT ( 'NONE',  ( 11.40812507854755253, -35.11059874428192273, -4.024999997268814411 ) ) ;
#81297=CARTESIAN_POINT ( 'NONE',  ( 23.74378949185148358, -32.05510596162020676, -22.01707947879874538 ) ) ;
#81324=CYLINDRICAL_SURFACE ( 'NONE', #41278, 9.100000000000001421 ) ;
#81336=FACE_OUTER_BOUND ( 'NONE', #114177, .T. ) ;
#81348=CARTESIAN_POINT ( 'NONE',  ( 36.91746824999999887, 11.99521256947799053, -3.524999997268813079 ) ) ;
#81352=DIRECTION ( 'NONE',  ( -0.000000000000000000, -0.000000000000000000, -1.000000000000000000 ) ) ;
#81367=CARTESIAN_POINT ( 'NONE',  ( -3.735172737399431091E-16, -6.100000000000006750, -64.53213882399991519 ) ) ;
#81381=CARTESIAN_POINT ( 'NONE',  ( 29.39134536520995766, -1.114265510929745240, -52.10946600208646373 ) ) ;
#81403=DIRECTION ( 'NONE',  ( -0.000000000000000000, -0.000000000000000000, 1.000000000000000000 ) ) ;
#81424=CARTESIAN_POINT ( 'NONE',  ( 37.99999999999999289, 2.893978650043524126E-14, -4.749999994537627224 ) ) ;
#81509=CARTESIAN_POINT ( 'NONE',  ( 37.99999999999999289, 2.893978650043524126E-14, -9.000000000000001776 ) ) ;
#81522=ORIENTED_EDGE ( 'NONE', *, *, #195610, .F. ) ;
#81530=CARTESIAN_POINT ( 'NONE',  ( -29.86685920354755197, -21.69954338932560134, -8.924999997268812990 ) ) ;
#81538=DIRECTION ( 'NONE',  ( 0.000000000000000000, 0.000000000000000000, 1.000000000000000000 ) ) ;
#81543=( BOUNDED_CURVE ( )  B_SPLINE_CURVE ( 2, ( #43740, #13398, #123529, #76047, #199407, #45718, #77039, #107371, #185223, #108377, #46714 ),
 .UNSPECIFIED., .F., .T. ) 
 B_SPLINE_CURVE_WITH_KNOTS ( ( 3, 2, 2, 2, 2, 3 ),
 ( 0.6000000000000000888, 0.6200000000000001066, 0.6400000000000001243, 0.6600000000000002531, 0.6800000000000002709, 0.7000000000000001776 ),
 .UNSPECIFIED. ) 
 CURVE ( )  GEOMETRIC_REPRESENTATION_ITEM ( )  RATIONAL_B_SPLINE_CURVE ( ( 0.9999999999999997780, 0.9510565162951537532, 1.000000000000000000, 0.9510565162951535312, 1.000000000000000000, 0.9510565162951535312, 1.000000000000000000, 0.9510565162951535312, 1.000000000000000000, 0.9510565162951529761, 1.000000000000000444 ) ) 
 REPRESENTATION_ITEM ( '' )  );
#81573=AXIS2_PLACEMENT_3D ( 'NONE', #23486, #132659, #85135 ) ;
#81575=CARTESIAN_POINT ( 'NONE',  ( 21.23184647844211881, -181.1785498424364675, -25.00000000000000000 ) ) ;
#81578=CARTESIAN_POINT ( 'NONE',  ( -36.91746825000001309, 11.99521256947798342, -5.224999997268811924 ) ) ;
#81653=ORIENTED_EDGE ( 'NONE', *, *, #41383, .T. ) ;
#81731=CARTESIAN_POINT ( 'NONE',  ( -24.30000000000002913, 0.1121107154833756725, -54.21489346206829651 ) ) ;
#81744=CARTESIAN_POINT ( 'NONE',  ( 23.48529157249599564, 32.32473071737754111, -0.6999999999999997335 ) ) ;
#81747=CARTESIAN_POINT ( 'NONE',  ( -29.85394078251578520, 1.399641368456010060, -51.58569050288880931 ) ) ;
#81756=EDGE_CURVE ( 'NONE', #56919, #120176, #86286, .T. ) ;
#81763=CARTESIAN_POINT ( 'NONE',  ( 28.92784451463930040, -27.23096741515436392, -20.32502560054408747 ) ) ;
#81765=CARTESIAN_POINT ( 'NONE',  ( -11.74264578624799782, -36.14014761921581709, -3.349999994537626868 ) ) ;
#81776=DIRECTION ( 'NONE',  ( 1.000000000000000000, 0.000000000000000000, 0.000000000000000000 ) ) ;
#81779=CARTESIAN_POINT ( 'NONE',  ( 26.42731554605158095, -26.90581007260905366, -20.33945912742372286 ) ) ;
#81791=CARTESIAN_POINT ( 'NONE',  ( -20.43538597629143538, -20.43538597629106945, -49.67367017693150189 ) ) ;
#81802=CARTESIAN_POINT ( 'NONE',  ( -3.573655867282028392E-15, 2.428612866367529932E-14, 0.000000000000000000 ) ) ;
#81814=CARTESIAN_POINT ( 'NONE',  ( -36.91746825000000598, 2.428612866367529932E-14, -1.124999997268813390 ) ) ;
#81817=EDGE_LOOP ( 'NONE', ( #116867, #87482, #89768, #108079 ) ) ;
#81822=CARTESIAN_POINT ( 'NONE',  ( -1.359215367441039879, -31.05479031690790492, -46.85916094508147012 ) ) ;
#81833=CARTESIAN_POINT ( 'NONE',  ( -17.67029085834473889, -36.01944455193051908, -22.64778610421867100 ) ) ;
#81868=CARTESIAN_POINT ( 'NONE',  ( -14.30340603398753885, 1.218621689577188416, -62.33590500446655369 ) ) ;
#81890=CARTESIAN_POINT ( 'NONE',  ( -9.349452323154864075, -36.27485578735121408, -31.39434858484993640 ) ) ;
#81900=CARTESIAN_POINT ( 'NONE',  ( -5.069580672095056251, -6.850104167616680506, -62.03238449839263069 ) ) ;
#81934=CIRCLE ( 'NONE', #78795, 10.00000000000000178 ) ;
#81962=DIRECTION ( 'NONE',  ( -0.000000000000000000, 0.000000000000000000, 1.000000000000000000 ) ) ;
#82012=CARTESIAN_POINT ( 'NONE',  ( 0.000000000000000000, 0.000000000000000000, -15.00000000000000000 ) ) ;
#82020=CIRCLE ( 'NONE', #159989, 40.00000000000000000 ) ;
#82035=VERTEX_POINT ( 'NONE', #92793 ) ;
#82036=CIRCLE ( 'NONE', #95345, 38.00000000000000000 ) ;
#82044=EDGE_CURVE ( 'NONE', #191474, #185826, #156105, .T. ) ;
#82046=VECTOR ( 'NONE', #60912, 1000.000000000000000 ) ;
#82054=AXIS2_PLACEMENT_3D ( 'NONE', #82060, #99242, #83075 ) ;
#82060=CARTESIAN_POINT ( 'NONE',  ( 0.000000000000000000, 0.000000000000000000, 0.000000000000000000 ) ) ;
#82064=CARTESIAN_POINT ( 'NONE',  ( 33.17841651222155974, -18.64421535753841397, -21.40882326905910560 ) ) ;
#82068=ORIENTED_EDGE ( 'NONE', *, *, #181804, .T. ) ;
#82080=AXIS2_PLACEMENT_3D ( 'NONE', #194047, #192022, #24193 ) ;
#82094=ORIENTED_EDGE ( 'NONE', *, *, #131324, .F. ) ;
#82222=ORIENTED_EDGE ( 'NONE', *, *, #178686, .T. ) ;
#82233=CARTESIAN_POINT ( 'NONE',  ( -26.63963442026891570, -26.88931099783081180, -16.54750829168120418 ) ) ;
#82259=LINE ( 'NONE', #5431, #179029 ) ;
#82264=CARTESIAN_POINT ( 'NONE',  ( 30.66720998790079022, -25.69103205420833902, -17.62974664729441798 ) ) ;
#82278=ORIENTED_EDGE ( 'NONE', *, *, #110488, .T. ) ;
#82282=CARTESIAN_POINT ( 'NONE',  ( -36.91746825000001309, -11.99521256947794789, -2.524999997268813523 ) ) ;
#82293=CARTESIAN_POINT ( 'NONE',  ( 23.17010908000658631, -32.51358278116848055, -22.50838357033831727 ) ) ;
#82342=VECTOR ( 'NONE', #122973, 1000.000000000000000 ) ;
#82345=CARTESIAN_POINT ( 'NONE',  ( 11.40812507854755253, -35.11059874428192273, -10.52499999726881263 ) ) ;
#82382=CARTESIAN_POINT ( 'NONE',  ( 31.82351365011403743, -0.4884129450683361018, -49.22894560581804058 ) ) ;
#82426=CIRCLE ( 'NONE', #43633, 6.100000000000006750 ) ;
#82496=CARTESIAN_POINT ( 'NONE',  ( 21.42625476241836679, 22.99713674769907001, -46.35568673344853607 ) ) ;
#82523=CARTESIAN_POINT ( 'NONE',  ( -36.91746825000000598, 11.99521256947798520, -2.724999997268813701 ) ) ;
#82538=CARTESIAN_POINT ( 'NONE',  ( -5.950531402560715689E-15, 38.81732327939063509, -9.624999997268815832 ) ) ;
#82564=AXIS2_PLACEMENT_3D ( 'NONE', #163038, #37689, #71036 ) ;
#82585=CARTESIAN_POINT ( 'NONE',  ( -22.81625015709510507, 31.40387420917330275, -5.424999997268812990 ) ) ;
#82586=CARTESIAN_POINT ( 'NONE',  ( -22.92260996908694892, 21.00373069265135584, -50.16862556671883056 ) ) ;
#82595=CARTESIAN_POINT ( 'NONE',  ( 16.24235425892372930, 17.62966412709566910, -57.02231465076383898 ) ) ;
#82607=ORIENTED_EDGE ( 'NONE', *, *, #195188, .T. ) ;
#82664=CIRCLE ( 'NONE', #198894, 2.500000000000000000 ) ;
#82673=CARTESIAN_POINT ( 'NONE',  ( -11.14892969833547198, -12.20117655778085819, -59.21778057892716163 ) ) ;
#82692=DIRECTION ( 'NONE',  ( 1.000000000000000000, 0.000000000000000000, 0.000000000000000000 ) ) ;
#82703=ORIENTED_EDGE ( 'NONE', *, *, #138326, .F. ) ;
#82712=CARTESIAN_POINT ( 'NONE',  ( -15.06137443927351072, 15.06137443927345210, -56.46919128290398504 ) ) ;
#82720=B_SPLINE_CURVE_WITH_KNOTS ( 'NONE', 3,
 ( #149053, #23707, #56030, #10541, #150047, #89359, #135873, #57043, #59012, #165220, #70210, #40868, #26715, #100530, #134890, #85355 ),
 .UNSPECIFIED., .F., .F.,
 ( 4, 2, 2, 2, 2, 2, 2, 4 ),
 ( 2.788292365851994434E-07, 0.0004449923513095699877, 0.0008897058733825547209, 0.001779132917528529392, 0.002223846439601516890, 0.002668559961674504388, 0.003113273483747491886, 0.003557987005820478950 ),
 .UNSPECIFIED. ) ;
#82732=CARTESIAN_POINT ( 'NONE',  ( -5.985463302383371875, -36.83348364107523309, -32.36600886826531109 ) ) ;
#82739=DIRECTION ( 'NONE',  ( 0.000000000000000000, 0.000000000000000000, 1.000000000000000000 ) ) ;
#82771=CARTESIAN_POINT ( 'NONE',  ( 30.65641173115121276, -25.45263461537905769, -21.37460845010012989 ) ) ;
#82787=CARTESIAN_POINT ( 'NONE',  ( 25.05471026796681500, -28.22563722313803325, -20.55515279800749795 ) ) ;
#82802=CIRCLE ( 'NONE', #66651, 40.00000000000000000 ) ;
#82810=CARTESIAN_POINT ( 'NONE',  ( -28.90000000000004476, 2.980639576201346218E-13, -52.65483682830183199 ) ) ;
#82823=CARTESIAN_POINT ( 'NONE',  ( -11.40812507854755609, 35.11059874428196537, -1.524999997268813301 ) ) ;
#82833=EDGE_CURVE ( 'NONE', #34604, #3755, #163292, .T. ) ;
#82845=CARTESIAN_POINT ( 'NONE',  ( -11.70497261680383261, -44.13276428439564825, -23.15274968897044516 ) ) ;
#82860=CIRCLE ( 'NONE', #108714, 2.500000000000000000 ) ;
#82874=CARTESIAN_POINT ( 'NONE',  ( 0.000000000000000000, -165.0000000000000000, 12.00000000000000355 ) ) ;
#82958=ORIENTED_EDGE ( 'NONE', *, *, #46060, .F. ) ;
#82996=ORIENTED_EDGE ( 'NONE', *, *, #34762, .T. ) ;
#83002=DIRECTION ( 'NONE',  ( -0.000000000000000000, -0.000000000000000000, 1.000000000000000000 ) ) ;
#83038=FACE_OUTER_BOUND ( 'NONE', #141773, .T. ) ;
#83047=B_SPLINE_CURVE_WITH_KNOTS ( 'NONE', 3,
 ( #84749, #80775, #19125, #142453, #190952, #68592, #20103, #83752, #176797, #146427, #52429, #38270, #188984, #4920, #112119, #81747, #157636, #99924, #143434, #145431, #7917, #69601, #66603, #51440, #54435, #113100, #97910, #159601 ),
 .UNSPECIFIED., .F., .F.,
 ( 4, 2, 2, 2, 2, 2, 2, 2, 2, 2, 2, 2, 2, 4 ),
 ( 1.961533960614312002E-07, 0.0003775868847195944732, 0.0007549776160431275265, 0.001132368347366660742, 0.001509759078690194175, 0.002264540541337254752, 0.003019322003984315113, 0.003774103466631376341, 0.004151494197954899365, 0.004528884929278421956, 0.004906275660601946281, 0.005283666391925468872, 0.005661057123248991463, 0.006038447854572514054 ),
 .UNSPECIFIED. ) ;
#83071=EDGE_CURVE ( 'NONE', #52978, #112132, #192285, .T. ) ;
#83075=DIRECTION ( 'NONE',  ( 1.000000000000000000, 0.000000000000000000, 0.000000000000000000 ) ) ;
#83079=CARTESIAN_POINT ( 'NONE',  ( 29.30938409335578854, -24.40035533028643755, -16.80062434859663512 ) ) ;
#83094=CIRCLE ( 'NONE', #73481, 21.30000000000002913 ) ;
#83102=EDGE_CURVE ( 'NONE', #188707, #149684, #21097, .T. ) ;
#83142=CARTESIAN_POINT ( 'NONE',  ( 17.18269478283314911, 17.18269478283310647, -56.77278709839600879 ) ) ;
#83267=CARTESIAN_POINT ( 'NONE',  ( -28.90000000000003411, 0.1353689087806527469, -49.67367017693149478 ) ) ;
#83271=LINE ( 'NONE', #9458, #4618 ) ;
#83291=CARTESIAN_POINT ( 'NONE',  ( 3.556970738554033499E-15, -38.81732327939057825, -10.12499999726881228 ) ) ;
#83301=CARTESIAN_POINT ( 'NONE',  ( 30.85002141291950295, -24.92539791875765331, -19.32025355660333688 ) ) ;
#83348=ORIENTED_EDGE ( 'NONE', *, *, #7609, .F. ) ;
#83350=CARTESIAN_POINT ( 'NONE',  ( -14.93657930744004148, -17.05128149819693917, -55.49887180089014294 ) ) ;
#83353=CARTESIAN_POINT ( 'NONE',  ( 3.556970738554033499E-15, -38.81732327939057825, -2.124999997268813612 ) ) ;
#83354=DIRECTION ( 'NONE',  ( 0.000000000000000000, 0.000000000000000000, 1.000000000000000000 ) ) ;
#83387=CARTESIAN_POINT ( 'NONE',  ( 29.12650189376885024, -0.8004727011104447731, -52.40478149256041007 ) ) ;
#83512=CARTESIAN_POINT ( 'NONE',  ( -22.78725946537530334, -32.81619059092837887, -22.84582334174709928 ) ) ;
#83524=CARTESIAN_POINT ( 'NONE',  ( -5.950531402560715689E-15, 38.81732327939063509, -5.124999997268813168 ) ) ;
#83572=CARTESIAN_POINT ( 'NONE',  ( 0.000000000000000000, -165.0000000000000000, 7.000000000000003553 ) ) ;
#83620=EDGE_CURVE ( 'NONE', #182074, #171133, #75897, .T. ) ;
#83715=ORIENTED_EDGE ( 'NONE', *, *, #28639, .F. ) ;
#83730=CARTESIAN_POINT ( 'NONE',  ( -6.020883695541781933, -38.43099163646787986, -23.90977630326744929 ) ) ;
#83736=CARTESIAN_POINT ( 'NONE',  ( -0.7813480796679098672, -13.90353822939981754, -62.49831333862088911 ) ) ;
#83749=CARTESIAN_POINT ( 'NONE',  ( -38.00000000000000711, 2.428612866367529932E-14, 0.000000000000000000 ) ) ;
#83752=CARTESIAN_POINT ( 'NONE',  ( -31.49504140153648635, 1.029908246020472040, -49.63772645510943704 ) ) ;
#83765=ORIENTED_EDGE ( 'NONE', *, *, #145712, .T. ) ;
#83777=AXIS2_PLACEMENT_3D ( 'NONE', #197342, #11338, #137633 ) ;
#83783=FACE_OUTER_BOUND ( 'NONE', #130737, .T. ) ;
#83786=CARTESIAN_POINT ( 'NONE',  ( -0.5954834035867282438, -31.78116016545939360, -49.28208245900471240 ) ) ;
#83806=DIRECTION ( 'NONE',  ( 0.000000000000000000, 0.000000000000000000, 1.000000000000000000 ) ) ;
#83821=CARTESIAN_POINT ( 'NONE',  ( -1.044764468832696025, -23.88070017481513929, -57.07230391339724918 ) ) ;
#83833=CARTESIAN_POINT ( 'NONE',  ( 0.000000000000000000, 0.000000000000000000, -58.85720012050612837 ) ) ;
#83839=CARTESIAN_POINT ( 'NONE',  ( -4.576660509524040243, -38.96431129323312348, -32.99999999890196989 ) ) ;
#84003=EDGE_CURVE ( 'NONE', #62967, #15377, #123131, .T. ) ;
#84010=CARTESIAN_POINT ( 'NONE',  ( 0.8197377589650296503, 24.06023304481832170, -54.40145518167209104 ) ) ;
#84028=FACE_BOUND ( 'NONE', #57034, .T. ) ;
#84030=CARTESIAN_POINT ( 'NONE',  ( 29.64655366937556380, -26.74020568361524752, -17.07338589137926022 ) ) ;
#84044=CARTESIAN_POINT ( 'NONE',  ( -13.74275686049844403, 0.4100021152178338069, -60.42614020214175241 ) ) ;
#84052=ORIENTED_EDGE ( 'NONE', *, *, #68000, .T. ) ;
#84072=CARTESIAN_POINT ( 'NONE',  ( -6.020228577223754586E-15, 39.95556452105416412, -10.24999999453762456 ) ) ;
#84091=AXIS2_PLACEMENT_3D ( 'NONE', #59065, #183417, #167259 ) ;
#84102=CARTESIAN_POINT ( 'NONE',  ( -3.573655867282028392E-15, 2.428612866367529932E-14, -25.00000000000000000 ) ) ;
#84151=CARTESIAN_POINT ( 'NONE',  ( -6.856101608890801443E-16, -64.85304063214812231, -22.99999966871703094 ) ) ;
#84178=CARTESIAN_POINT ( 'NONE',  ( -29.82770300773734107, -26.65766548392525692, -16.82146946961924527 ) ) ;
#84184=CARTESIAN_POINT ( 'NONE',  ( -20.00321537600460431, -21.32363904033505975, -52.29808436870553123 ) ) ;
#84237=VERTEX_POINT ( 'NONE', #13972 ) ;
#84264=DIRECTION ( 'NONE',  ( 1.000000000000000000, 0.000000000000000000, 0.000000000000000000 ) ) ;
#84265=CARTESIAN_POINT ( 'NONE',  ( -38.00000000000000711, 2.428612866367529932E-14, -7.749999994537626336 ) ) ;
#84287=CARTESIAN_POINT ( 'NONE',  ( 30.74264578624800137, -22.33583958711395212, -1.200000000000000178 ) ) ;
#84310=VERTEX_POINT ( 'NONE', #91784 ) ;
#84317=ORIENTED_EDGE ( 'NONE', *, *, #95584, .T. ) ;
#84349=CARTESIAN_POINT ( 'NONE',  ( 36.91746824999999887, 11.99521256947799053, -5.524999997268812635 ) ) ;
#84384=CARTESIAN_POINT ( 'NONE',  ( 30.26186088262144835, -1.502453648625374116, -51.11561252063852834 ) ) ;
#84387=DIRECTION ( 'NONE',  ( -0.000000000000000000, -0.000000000000000000, 1.000000000000000000 ) ) ;
#84390=EDGE_CURVE ( 'NONE', #76158, #16157, #183613, .T. ) ;
#84516=EDGE_LOOP ( 'NONE', ( #5420, #74084, #155981, #198406, #112581 ) ) ;
#84520=DIRECTION ( 'NONE',  ( 0.000000000000000000, 0.000000000000000000, -1.000000000000000000 ) ) ;
#84531=CARTESIAN_POINT ( 'NONE',  ( 28.86264817322070542, -27.69526727176378245, -15.91384944864139861 ) ) ;
#84592=CARTESIAN_POINT ( 'NONE',  ( 14.98335265924517579, 15.13939621930179058, -58.85720012050614969 ) ) ;
#84623=B_SPLINE_CURVE_WITH_KNOTS ( 'NONE', 3,
 ( #154628, #45465, #106134, #136480, #198160, #93942, #59630, #29317, #60615, #169796, #140445, #16123, #17117, #46452, #28341, #90947, #200139, #152634, #109116, #928, #122290, #78768, #77778, #76787 ),
 .UNSPECIFIED., .F., .F.,
 ( 4, 2, 2, 2, 2, 2, 2, 2, 2, 2, 2, 4 ),
 ( 2.775519118949223281E-07, 0.0003993838752237342609, 0.0007984901985355736219, 0.001596702845159247899, 0.002394915491782921742, 0.003193128138406596019, 0.003991340785030269428, 0.004789553431653943705, 0.005188659754965783445, 0.005587766078277624920, 0.005986872401589464661, 0.006385978724901306136 ),
 .UNSPECIFIED. ) ;
#84631=EDGE_CURVE ( 'NONE', #100015, #76158, #79619, .T. ) ;
#84741=EDGE_CURVE ( 'NONE', #197513, #89826, #65436, .T. ) ;
#84749=CARTESIAN_POINT ( 'NONE',  ( -31.90000000000003411, 3.219216299777112361E-13, -49.13275782002545355 ) ) ;
#84754=CARTESIAN_POINT ( 'NONE',  ( -6.434671708797603529, 6.434671708797564449, -63.95112321872120731 ) ) ;
#84762=ORIENTED_EDGE ( 'NONE', *, *, #32808, .F. ) ;
#84765=FACE_OUTER_BOUND ( 'NONE', #134673, .T. ) ;
#84767=CARTESIAN_POINT ( 'NONE',  ( -6.020228577223754586E-15, 39.95556452105416412, -6.249999994537626336 ) ) ;
#84776=DIRECTION ( 'NONE',  ( -0.000000000000000000, -0.000000000000000000, 1.000000000000000000 ) ) ;
#84780=DIRECTION ( 'NONE',  ( -0.000000000000000000, -0.000000000000000000, 1.000000000000000000 ) ) ;
#84784=CARTESIAN_POINT ( 'NONE',  ( -1.046637022530759076, -29.32058373238551852, -52.18867397238358308 ) ) ;
#84802=CYLINDRICAL_SURFACE ( 'NONE', #189261, 59.99999999999998579 ) ;
#84817=CARTESIAN_POINT ( 'NONE',  ( 29.86685920354754487, 21.69954338932564752, -7.924999997268814766 ) ) ;
#84826=CARTESIAN_POINT ( 'NONE',  ( -0.9155518048963315891, -29.20736712825161874, -49.29216761470102881 ) ) ;
#84834=ORIENTED_EDGE ( 'NONE', *, *, #17351, .F. ) ;
#84840=CARTESIAN_POINT ( 'NONE',  ( 0.000000000000000000, 0.000000000000000000, -18.00000000000000000 ) ) ;
#84841=ORIENTED_EDGE ( 'NONE', *, *, #10071, .T. ) ;
#84852=CARTESIAN_POINT ( 'NONE',  ( 9.687362902255726382, 9.687362902255699737, -62.58071313852362039 ) ) ;
#84867=CYLINDRICAL_SURFACE ( 'NONE', #8128, 13.70000000000001528 ) ;
#84873=VECTOR ( 'NONE', #184532, 1000.000000000000000 ) ;
#84875=CARTESIAN_POINT ( 'NONE',  ( 0.000000000000000000, 0.000000000000000000, -64.92179855667829713 ) ) ;
#84911=DIRECTION ( 'NONE',  ( -0.000000000000000000, -0.000000000000000000, 1.000000000000000000 ) ) ;
#84974=AXIS2_PLACEMENT_3D ( 'NONE', #42536, #56706, #134550 ) ;
#84994=CARTESIAN_POINT ( 'NONE',  ( 0.000000000000000000, 0.000000000000000000, -64.53213882399991519 ) ) ;
#85040=CARTESIAN_POINT ( 'NONE',  ( -16.70000000000002061, 1.759457951533292443E-13, -59.13370768023891344 ) ) ;
#85074=CARTESIAN_POINT ( 'NONE',  ( 26.63963442026837214, -26.88931099783062351, -16.54750829168370529 ) ) ;
#85102=VERTEX_POINT ( 'NONE', #144263 ) ;
#85111=CIRCLE ( 'NONE', #130418, 4.000000000000000888 ) ;
#85135=DIRECTION ( 'NONE',  ( 1.000000000000000000, 0.000000000000000000, 0.000000000000000000 ) ) ;
#85138=ORIENTED_EDGE ( 'NONE', *, *, #59660, .T. ) ;
#85188=EDGE_CURVE ( 'NONE', #4644, #171283, #95949, .T. ) ;
#85226=VERTEX_POINT ( 'NONE', #99756 ) ;
#85233=CARTESIAN_POINT ( 'NONE',  ( -38.00000000000000711, -12.34694845685042708, -3.899999999999999911 ) ) ;
#85242=CARTESIAN_POINT ( 'NONE',  ( 1.037572752228153927, 29.31194926455886929, -52.19832300604669229 ) ) ;
#85259=AXIS2_PLACEMENT_3D ( 'NONE', #5204, #36539, #97205 ) ;
#85269=CARTESIAN_POINT ( 'NONE',  ( 37.99999999999999289, 2.893978650043524126E-14, -6.749999994537627224 ) ) ;
#85273=CARTESIAN_POINT ( 'NONE',  ( 0.000000000000000000, -105.0000000000000000, -23.00000000000000000 ) ) ;
#85289=CARTESIAN_POINT ( 'NONE',  ( -30.74264578624800492, 22.33583958711400186, -2.200000000000000178 ) ) ;
#85298=CARTESIAN_POINT ( 'NONE',  ( 35.08666314276448617, -21.80769648729754806, -18.77091308353056576 ) ) ;
#85310=AXIS2_PLACEMENT_3D ( 'NONE', #132024, #68342, #129992 ) ;
#85313=VERTEX_POINT ( 'NONE', #131095 ) ;
#85350=CARTESIAN_POINT ( 'NONE',  ( 22.81625015709510151, -31.40387420917324590, -9.924999997268814766 ) ) ;
#85355=CARTESIAN_POINT ( 'NONE',  ( 6.874011537017776341, -5.374011537017756801, -64.03675147074802965 ) ) ;
#85361=EDGE_CURVE ( 'NONE', #115644, #50694, #128574, .T. ) ;
#85382=DIRECTION ( 'NONE',  ( -0.000000000000000000, -0.000000000000000000, -1.000000000000000000 ) ) ;
#85491=AXIS2_PLACEMENT_3D ( 'NONE', #20454, #141808, #2307 ) ;
#85502=CARTESIAN_POINT ( 'NONE',  ( 21.15706064682975196, 22.96834507599301034, -46.65423976109394033 ) ) ;
#85517=CARTESIAN_POINT ( 'NONE',  ( 0.000000000000000000, 0.000000000000000000, -56.46919128290398504 ) ) ;
#85528=CARTESIAN_POINT ( 'NONE',  ( 22.81625015709510151, -31.40387420917324590, -3.924999997268812102 ) ) ;
#85538=EDGE_CURVE ( 'NONE', #53136, #107603, #117944, .T. ) ;
#85539=CARTESIAN_POINT ( 'NONE',  ( -30.44363203418366481, -22.74636568843913409, -19.69742113251491489 ) ) ;
#85566=ORIENTED_EDGE ( 'NONE', *, *, #87955, .F. ) ;
#85604=CARTESIAN_POINT ( 'NONE',  ( 15.19424636789221417, 17.31426855362213146, -57.70166256124680615 ) ) ;
#85608=ORIENTED_EDGE ( 'NONE', *, *, #182123, .T. ) ;
#85641=VECTOR ( 'NONE', #154276, 1000.000000000000000 ) ;
#85682=DIRECTION ( 'NONE',  ( -0.000000000000000000, -0.000000000000000000, 1.000000000000000000 ) ) ;
#85699=AXIS2_PLACEMENT_3D ( 'NONE', #157909, #77081, #189257 ) ;
#85722=DIRECTION ( 'NONE',  ( -0.000000000000000000, -0.000000000000000000, 1.000000000000000000 ) ) ;
#85744=CARTESIAN_POINT ( 'NONE',  ( 10.34110108248005133, -9.296341836507240330, -62.50551787159913886 ) ) ;
#85746=CARTESIAN_POINT ( 'NONE',  ( -1.022580077288041090E-15, -16.70000000000002061, -61.34707691135562868 ) ) ;
#85764=AXIS2_PLACEMENT_3D ( 'NONE', #172993, #126470, #62803 ) ;
#85779=ADVANCED_FACE ( 'NONE', ( #77392 ), #166452, .F. ) ;
#85783=CARTESIAN_POINT ( 'NONE',  ( 11.74264578624800315, -36.14014761921581709, -7.149999994537626691 ) ) ;
#85790=CARTESIAN_POINT ( 'NONE',  ( 4.419823376501902601, -4.206879353973994817, -62.50719930893271226 ) ) ;
#85796=CARTESIAN_POINT ( 'NONE',  ( -3.573655867282028392E-15, 2.428612866367529932E-14, -25.00000000000000000 ) ) ;
#85833=CARTESIAN_POINT ( 'NONE',  ( 36.91746824999999887, -11.99521256947793546, -6.224999997268814589 ) ) ;
#85843=CARTESIAN_POINT ( 'NONE',  ( -0.5143648618586742494, -28.98522958361497359, -49.56847006845431736 ) ) ;
#85847=CARTESIAN_POINT ( 'NONE',  ( -4.313351365237961588, 4.313351365237934942, -64.53213882399992940 ) ) ;
#85854=CARTESIAN_POINT ( 'NONE',  ( -23.69010019206611872, -31.82897765507213705, -19.48018210901399883 ) ) ;
#85855=ORIENTED_EDGE ( 'NONE', *, *, #85188, .F. ) ;
#85866=ORIENTED_EDGE ( 'NONE', *, *, #85994, .F. ) ;
#85868=TOROIDAL_SURFACE ( 'NONE', #137534, 69.99999999999998579, 8.000000000000000000 ) ;
#85871=CARTESIAN_POINT ( 'NONE',  ( -17.18269478283316332, 17.18269478283309226, -56.77278709839600879 ) ) ;
#85899=ORIENTED_EDGE ( 'NONE', *, *, #24537, .F. ) ;
#85989=CARTESIAN_POINT ( 'NONE',  ( 0.2731799622684817352, 31.88037471264000544, -45.67814385241111808 ) ) ;
#85994=EDGE_CURVE ( 'NONE', #100015, #87857, #47940, .T. ) ;
#86007=ORIENTED_EDGE ( 'NONE', *, *, #173264, .F. ) ;
#86010=CYLINDRICAL_SURFACE ( 'NONE', #34336, 4.000000000000000888 ) ;
#86038=CARTESIAN_POINT ( 'NONE',  ( 20.43538597629129328, 20.43538597629121156, -52.65483682830182488 ) ) ;
#86084=( NAMED_UNIT ( * ) PLANE_ANGLE_UNIT ( ) SI_UNIT ( $, .RADIAN. ) );
#86154=DIRECTION ( 'NONE',  ( -0.000000000000000000, -0.000000000000000000, -1.000000000000000000 ) ) ;
#86244=CARTESIAN_POINT ( 'NONE',  ( 3.766062262543149401E-15, -39.95556452105413570, -3.499999999999999556 ) ) ;
#86278=CARTESIAN_POINT ( 'NONE',  ( 37.99999999999999289, 2.428612866367529932E-14, 0.000000000000000000 ) ) ;
#86279=CARTESIAN_POINT ( 'NONE',  ( 15.06137443927351249, -15.06137443927345210, -58.85720012050613548 ) ) ;
#86281=CARTESIAN_POINT ( 'NONE',  ( 16.16661445520356821, -1.151164073136631272, -59.37042179516131313 ) ) ;
#86283=CARTESIAN_POINT ( 'NONE',  ( -69.65682714487590488, -71.74905178543390605, -25.00000000000000000 ) ) ;
#86286=B_SPLINE_CURVE_WITH_KNOTS ( 'NONE', 3,
 ( #48305, #124126, #198010, #122144, #168646, #44330, #184821, #46306, #107962, #59480, #185825, #15974, #32136, #14978 ),
 .UNSPECIFIED., .F., .F.,
 ( 4, 2, 2, 2, 2, 2, 4 ),
 ( 1.971416326048476669E-07, 0.0002961152624844829405, 0.0005920333833363609737, 0.0008879515041882391152, 0.001183869625040117257, 0.001775705866743883081, 0.002367542108447648688 ),
 .UNSPECIFIED. ) ;
#86301=CARTESIAN_POINT ( 'NONE',  ( 11.40812507854755253, -35.11059874428192273, -8.024999997268814411 ) ) ;
#86310=CARTESIAN_POINT ( 'NONE',  ( 34.63261191446840570, -20.08610687337147382, -21.92908410840965772 ) ) ;
#86315=B_SPLINE_CURVE_WITH_KNOTS ( 'NONE', 3,
 ( #131704, #84178, #68023, #55859, #7340, #129674 ),
 .UNSPECIFIED., .F., .F.,
 ( 4, 2, 4 ),
 ( 0.02150008358963344246, 0.02352197444946371035, 0.02554386530929397825 ),
 .UNSPECIFIED. ) ;
#86328=CARTESIAN_POINT ( 'NONE',  ( 3.620324696381902907, -38.95353743399085289, -23.38767721381919884 ) ) ;
#86338=CARTESIAN_POINT ( 'NONE',  ( -21.71309667856399628, -34.72214947970702781, -18.33762378602112264 ) ) ;
#86347=AXIS2_PLACEMENT_3D ( 'NONE', #162604, #24108, #26112 ) ;
#86357=EDGE_LOOP ( 'NONE', ( #105686, #15093, #145758, #61939 ) ) ;
#86362=CARTESIAN_POINT ( 'NONE',  ( 36.91746825000000598, -11.99521256947793546, -5.724999997268813701 ) ) ;
#86396=DIRECTION ( 'NONE',  ( 1.000000000000000000, 0.000000000000000000, 0.000000000000000000 ) ) ;
#86398=CARTESIAN_POINT ( 'NONE',  ( 193.3062444957835453, -155.7167183371837496, -23.00000000000000000 ) ) ;
#86401=DIRECTION ( 'NONE',  ( 1.000000000000000000, 0.000000000000000000, 0.000000000000000000 ) ) ;
#86442=LINE ( 'NONE', #101605, #92638 ) ;
#86482=ORIENTED_EDGE ( 'NONE', *, *, #75962, .T. ) ;
#86485=CARTESIAN_POINT ( 'NONE',  ( -3.735172737399431091E-16, -6.100000000000006750, -62.50719930893269805 ) ) ;
#86532=ORIENTED_EDGE ( 'NONE', *, *, #31655, .F. ) ;
#86536=CARTESIAN_POINT ( 'NONE',  ( 36.91746824999999177, 11.99521256947799230, -1.524999997268813523 ) ) ;
#86579=AXIS2_PLACEMENT_3D ( 'NONE', #91940, #89983, #153633 ) ;
#86595=CARTESIAN_POINT ( 'NONE',  ( 31.77050690183225257, -0.6194686979412523664, -45.83912112027729080 ) ) ;
#86612=ORIENTED_EDGE ( 'NONE', *, *, #83102, .T. ) ;
#86619=VERTEX_POINT ( 'NONE', #61224 ) ;
#86664=ORIENTED_EDGE ( 'NONE', *, *, #12763, .T. ) ;
#86665=EDGE_LOOP ( 'NONE', ( #39990, #157482, #111442, #81009 ) ) ;
#86720=CARTESIAN_POINT ( 'NONE',  ( 16.12203461105333702, -16.12203461105326951, -64.92279855667830191 ) ) ;
#86738=CARTESIAN_POINT ( 'NONE',  ( -22.30909568229876072, -31.30078617544283048, -17.06157116626747694 ) ) ;
#86744=VECTOR ( 'NONE', #36846, 1000.000000000000000 ) ;
#86745=CARTESIAN_POINT ( 'NONE',  ( -0.9460486868805269012, -16.38029848613151174, -61.48057501744756337 ) ) ;
#86782=CARTESIAN_POINT ( 'NONE',  ( -23.48529157249600985, 32.32473071737754111, -8.049999994537627046 ) ) ;
#86790=DIRECTION ( 'NONE',  ( -0.000000000000000000, -0.000000000000000000, -1.000000000000000000 ) ) ;
#86795=CARTESIAN_POINT ( 'NONE',  ( -11.67169337655814410, 9.562403590618668403, -59.87610203618464766 ) ) ;
#86799=ORIENTED_EDGE ( 'NONE', *, *, #88864, .T. ) ;
#86821=EDGE_CURVE ( 'NONE', #56776, #188843, #37941, .T. ) ;
#86834=CARTESIAN_POINT ( 'NONE',  ( -11.40812507854754720, -35.11059874428192273, -4.724999997268812812 ) ) ;
#86845=CARTESIAN_POINT ( 'NONE',  ( -26.46959431505283789, -27.26463967846487435, -15.00000000000000178 ) ) ;
#86858=CARTESIAN_POINT ( 'NONE',  ( -28.30573922537829290, -27.84595035627394921, -20.14355118861611516 ) ) ;
#86884=CARTESIAN_POINT ( 'NONE',  ( 0.1032920037969625171, 16.70000000000001705, -61.34707691135563579 ) ) ;
#86890=( BOUNDED_CURVE ( )  B_SPLINE_CURVE ( 2, ( #67338, #64367, #141201, #172546, #96672, #174536, #111858, #65351, #171551, #20836, #33040 ),
 .UNSPECIFIED., .F., .T. ) 
 B_SPLINE_CURVE_WITH_KNOTS ( ( 3, 2, 2, 2, 2, 3 ),
 ( 0.5000000000000000000, 0.5200000000000000178, 0.5400000000000000355, 0.5600000000000001643, 0.5800000000000000711, 0.6000000000000000888 ),
 .UNSPECIFIED. ) 
 CURVE ( )  GEOMETRIC_REPRESENTATION_ITEM ( )  RATIONAL_B_SPLINE_CURVE ( ( 1.000000000000000000, 0.9510565162951535312, 1.000000000000000000, 0.9510565162951535312, 1.000000000000000000, 0.9510565162951535312, 1.000000000000000000, 0.9510565162951535312, 1.000000000000000000, 0.9510565162951533091, 1.000000000000000222 ) ) 
 REPRESENTATION_ITEM ( '' )  );
#86893=CARTESIAN_POINT ( 'NONE',  ( -0.9277198534072325087, -6.404810000729023400, -62.44539631020980863 ) ) ;
#86911=CARTESIAN_POINT ( 'NONE',  ( -5.374011537017813644, -5.374011537017721274, -64.92279855667830191 ) ) ;
#86919=ADVANCED_FACE ( 'NONE', ( #20687 ), #171407, .T. ) ;
#86988=DIRECTION ( 'NONE',  ( -0.000000000000000000, -0.000000000000000000, 1.000000000000000000 ) ) ;
#87009=ORIENTED_EDGE ( 'NONE', *, *, #98272, .T. ) ;
#87095=ORIENTED_EDGE ( 'NONE', *, *, #182320, .T. ) ;
#87156=ORIENTED_EDGE ( 'NONE', *, *, #32194, .T. ) ;
#87165=EDGE_CURVE ( 'NONE', #167693, #174271, #96522, .T. ) ;
#87256=CARTESIAN_POINT ( 'NONE',  ( -9.444051989377744150, -10.00006765622181604, -62.56086220006871912 ) ) ;
#87275=CARTESIAN_POINT ( 'NONE',  ( 1.304248841091933035E-15, 21.30000000000002913, -56.46919128290398504 ) ) ;
#87282=DIRECTION ( 'NONE',  ( 1.000000000000000000, 6.391086490440868450E-16, 0.000000000000000000 ) ) ;
#87298=CIRCLE ( 'NONE', #113106, 4.000000000000000888 ) ;
#87302=ORIENTED_EDGE ( 'NONE', *, *, #131670, .T. ) ;
#87305=CARTESIAN_POINT ( 'NONE',  ( -11.40812507854755609, 35.11059874428196537, -9.024999997268814411 ) ) ;
#87310=CARTESIAN_POINT ( 'NONE',  ( 0.4053451330847814282, 16.64779159201958691, -59.15694982147774539 ) ) ;
#87327=ORIENTED_EDGE ( 'NONE', *, *, #5408, .F. ) ;
#87330=CARTESIAN_POINT ( 'NONE',  ( 5.985463302384318673, -36.83348364107504835, -32.36600886826526136 ) ) ;
#87334=ORIENTED_EDGE ( 'NONE', *, *, #168981, .F. ) ;
#87364=CARTESIAN_POINT ( 'NONE',  ( -29.86685920354755197, -21.69954338932560134, -6.424999997268812990 ) ) ;
#87397=DIRECTION ( 'NONE',  ( -0.000000000000000000, -0.000000000000000000, 1.000000000000000000 ) ) ;
#87482=ORIENTED_EDGE ( 'NONE', *, *, #144540, .T. ) ;
#87497=ORIENTED_EDGE ( 'NONE', *, *, #183262, .T. ) ;
#87510=CARTESIAN_POINT ( 'NONE',  ( -9.979912183652590585, -44.24332767168411351, -21.75883150241363495 ) ) ;
#87526=CARTESIAN_POINT ( 'NONE',  ( -33.78191506369886810, -21.41920200728862511, -24.99999999999999289 ) ) ;
#87536=CARTESIAN_POINT ( 'NONE',  ( -22.81625015709510507, 31.40387420917330275, -6.924999997268812990 ) ) ;
#87666=PRESENTATION_STYLE_ASSIGNMENT (( #73526 ) ) ;
#87740=FACE_OUTER_BOUND ( 'NONE', #154124, .T. ) ;
#87768=ORIENTED_EDGE ( 'NONE', *, *, #111598, .F. ) ;
#87772=DIRECTION ( 'NONE',  ( 0.000000000000000000, 0.000000000000000000, -1.000000000000000000 ) ) ;
#87776=CARTESIAN_POINT ( 'NONE',  ( -30.74264578624800492, 22.33583958711400186, -9.949999994537627401 ) ) ;
#87784=CARTESIAN_POINT ( 'NONE',  ( 22.99604614807110181, -21.49604614807103786, -46.28618945597792589 ) ) ;
#87792=EDGE_LOOP ( 'NONE', ( #90131, #126341, #105868, #28880 ) ) ;
#87824=CARTESIAN_POINT ( 'NONE',  ( -29.86685920354755552, 21.69954338932564397, -7.324999997268814234 ) ) ;
#87834=CARTESIAN_POINT ( 'NONE',  ( 31.22300027783691334, -21.66299953960490043, -21.91126201009245023 ) ) ;
#87846=CARTESIAN_POINT ( 'NONE',  ( -21.53686564358551792, -33.52628202223520759, -20.57266355564332727 ) ) ;
#87857=VERTEX_POINT ( 'NONE', #164218 ) ;
#87886=EDGE_CURVE ( 'NONE', #19028, #197049, #71136, .T. ) ;
#87890=ORIENTED_EDGE ( 'NONE', *, *, #89537, .F. ) ;
#87908=B_SPLINE_CURVE_WITH_KNOTS ( 'NONE', 3,
 ( #100449, #82264, #116625, #143956, #159118, #71126, #147974, #162129, #53957, #22623, #23625, #7432, #67120, #128778 ),
 .UNSPECIFIED., .F., .F.,
 ( 4, 2, 2, 2, 2, 2, 4 ),
 ( 6.009258394948636926E-18, 0.002470145813542335908, 0.004940291627084665745, 0.007410437440626995581, 0.008645510347398159198, 0.009263046800783741874, 0.009880583254169324550 ),
 .UNSPECIFIED. ) ;
#87916=CARTESIAN_POINT ( 'NONE',  ( 193.3062444957835453, -155.7167183371837496, -23.00000000000000000 ) ) ;
#87955=EDGE_CURVE ( 'NONE', #133509, #101645, #192549, .T. ) ;
#87982=CARTESIAN_POINT ( 'NONE',  ( 1.499999999999985123, 30.56208168264224412, -47.53402626646857954 ) ) ;
#88027=CARTESIAN_POINT ( 'NONE',  ( 22.55670631985092811, 22.55670631985084640, -49.13275782002545355 ) ) ;
#88053=ORIENTED_EDGE ( 'NONE', *, *, #42790, .F. ) ;
#88073=CARTESIAN_POINT ( 'NONE',  ( -6.863278975470372245, 5.170161995863669979, -64.06628402976478753 ) ) ;
#88107=VECTOR ( 'NONE', #46615, 1000.000000000000000 ) ;
#88144=DIRECTION ( 'NONE',  ( -0.000000000000000000, -0.000000000000000000, 1.000000000000000000 ) ) ;
#88162=APPLICATION_CONTEXT ( 'automotive_design' ) ;
#88188=LINE ( 'NONE', #73047, #24839 ) ;
#88245=CARTESIAN_POINT ( 'NONE',  ( -9.285263851164359039, -10.36200767871436490, -62.50269714056246073 ) ) ;
#88262=CARTESIAN_POINT ( 'NONE',  ( 69.65682714487590488, -71.74905178543389184, -15.00000000000000178 ) ) ;
#88277=CARTESIAN_POINT ( 'NONE',  ( 12.24802307403555446, -10.74802307403551715, -64.92279855667830191 ) ) ;
#88292=CARTESIAN_POINT ( 'NONE',  ( -38.00000000000000711, 2.428612866367529932E-14, -4.000000000000000000 ) ) ;
#88297=CARTESIAN_POINT ( 'NONE',  ( 0.9489761088441257542, 16.37794455013558093, -59.27687827943704946 ) ) ;
#88318=CARTESIAN_POINT ( 'NONE',  ( 7.840974544913427380, -46.02298249793697948, -22.40017284086515303 ) ) ;
#88345=ORIENTED_EDGE ( 'NONE', *, *, #191015, .T. ) ;
#88350=CARTESIAN_POINT ( 'NONE',  ( -36.91746825000000598, 2.428612866367529932E-14, -6.624999997268814056 ) ) ;
#88392=TOROIDAL_SURFACE ( 'NONE', #188567, 206.0437394197456911, 10.00000000000000000 ) ;
#88460=VECTOR ( 'NONE', #60918, 1000.000000000000000 ) ;
#88480=CIRCLE ( 'NONE', #56440, 61.99999999999998579 ) ;
#88504=CARTESIAN_POINT ( 'NONE',  ( -27.93585545099111656, -25.65867777193844645, -16.61539413803384946 ) ) ;
#88509=EDGE_CURVE ( 'NONE', #19675, #74853, #6197, .T. ) ;
#88530=CARTESIAN_POINT ( 'NONE',  ( -30.66585169841567193, -25.69259602932061881, -17.62843888640922785 ) ) ;
#88548=CARTESIAN_POINT ( 'NONE',  ( 7.095528360788435407, -39.96100899395969464, -25.59277598899998196 ) ) ;
#88561=VECTOR ( 'NONE', #15882, 1000.000000000000000 ) ;
#88602=CARTESIAN_POINT ( 'NONE',  ( -9.297033629063200522E-15, -64.87124026077283645, -24.99999901254159695 ) ) ;
#88665=ORIENTED_EDGE ( 'NONE', *, *, #62849, .F. ) ;
#88676=ADVANCED_FACE ( 'NONE', ( #160266 ), #144091, .F. ) ;
#88722=CARTESIAN_POINT ( 'NONE',  ( -17.45991095687933026, 16.83259678516729707, -54.25516819912629529 ) ) ;
#88773=VERTEX_POINT ( 'NONE', #146083 ) ;
#88775=DIRECTION ( 'NONE',  ( -0.000000000000000000, 0.000000000000000000, 1.000000000000000000 ) ) ;
#88779=CARTESIAN_POINT ( 'NONE',  ( -23.48529157249600985, 32.32473071737754111, -6.049999994537625270 ) ) ;
#88792=CARTESIAN_POINT ( 'NONE',  ( -10.01085954718718440, 9.437681514439628216, -60.42207423661104571 ) ) ;
#88810=DIRECTION ( 'NONE',  ( 1.000000000000000000, 0.000000000000000000, 0.000000000000000000 ) ) ;
#88829=CARTESIAN_POINT ( 'NONE',  ( -36.91746825000000598, -11.99521256947794789, -7.024999997268812635 ) ) ;
#88830=CARTESIAN_POINT ( 'NONE',  ( -0.4315818942737878472, -21.35939100396077706, -58.81718527612537883 ) ) ;
#88832=CARTESIAN_POINT ( 'NONE',  ( -29.86685920354755552, 21.69954338932564397, -1.324999997268813345 ) ) ;
#88850=CARTESIAN_POINT ( 'NONE',  ( -31.47347929072011397, -24.22385046035113731, -19.66336643902676329 ) ) ;
#88864=EDGE_CURVE ( 'NONE', #43345, #171283, #129898, .T. ) ;
#88866=CARTESIAN_POINT ( 'NONE',  ( -0.4877194249720437358, -9.021937450273805226, -63.96635223026897421 ) ) ;
#88903=ORIENTED_EDGE ( 'NONE', *, *, #61218, .F. ) ;
#88922=DIRECTION ( 'NONE',  ( -0.000000000000000000, -0.000000000000000000, -1.000000000000000000 ) ) ;
#88935=B_SPLINE_CURVE_WITH_KNOTS ( 'NONE', 3,
 ( #41057, #54220, #73400, #178574, #84531, #53207, #164409, #163403 ),
 .UNSPECIFIED., .F., .F.,
 ( 4, 2, 2, 4 ),
 ( -3.098386792788301083E-05, 0.0009765746000771589885, 0.001984133068082204274, 0.003999250004092276198 ),
 .UNSPECIFIED. ) ;
#88954=AXIS2_PLACEMENT_3D ( 'NONE', #2188, #4166, #17368 ) ;
#88986=CARTESIAN_POINT ( 'NONE',  ( -24.75282386541777413, -28.51018972888603642, -20.68147073028497118 ) ) ;
#89002=EDGE_LOOP ( 'NONE', ( #50932, #92528, #39975, #35183, #146978 ) ) ;
#89013=AXIS2_PLACEMENT_3D ( 'NONE', #27401, #150736, #185030 ) ;
#89021=ORIENTED_EDGE ( 'NONE', *, *, #175399, .F. ) ;
#89051=AXIS2_PLACEMENT_3D ( 'NONE', #193982, #132290, #55444 ) ;
#89070=CARTESIAN_POINT ( 'NONE',  ( 1.500000000000008216, 22.80000000000002913, -65.00100000000003320 ) ) ;
#89142=CARTESIAN_POINT ( 'NONE',  ( 0.000000000000000000, -105.0000000000000000, 12.00000000000000355 ) ) ;
#89147=CARTESIAN_POINT ( 'NONE',  ( -20.43538597629128262, 20.43538597629122222, -65.00100000000003320 ) ) ;
#89167=CARTESIAN_POINT ( 'NONE',  ( -9.687362902255793884, -9.687362902255632235, -62.58071313852362039 ) ) ;
#89182=CARTESIAN_POINT ( 'NONE',  ( 23.48529157249600630, -32.32473071737748427, -3.049999994537627046 ) ) ;
#89236=VERTEX_POINT ( 'NONE', #34931 ) ;
#89240=AXIS2_PLACEMENT_3D ( 'NONE', #69655, #67652, #6966 ) ;
#89245=AXIS2_PLACEMENT_3D ( 'NONE', #43805, #62925, #186300 ) ;
#89279=CARTESIAN_POINT ( 'NONE',  ( -1.374935097489159874, -23.51385019162033174, -54.82293943248599533 ) ) ;
#89294=ORIENTED_EDGE ( 'NONE', *, *, #57363, .T. ) ;
#89297=CARTESIAN_POINT ( 'NONE',  ( 11.74264578624799427, 36.14014761921585972, -4.599999999999999645 ) ) ;
#89302=CARTESIAN_POINT ( 'NONE',  ( 1.429357700123697894, 15.66473995800721575, -59.59166688515647792 ) ) ;
#89340=AXIS2_PLACEMENT_3D ( 'NONE', #2889, #21039, #186944 ) ;
#89350=DIRECTION ( 'NONE',  ( 1.000000000000000000, 0.000000000000000000, 0.000000000000000000 ) ) ;
#89355=CARTESIAN_POINT ( 'NONE',  ( 0.2065856650645460646, 13.70000000000002061, -62.58071313852362039 ) ) ;
#89359=CARTESIAN_POINT ( 'NONE',  ( 5.379963195099918494, -3.845052905827775369, -64.45073299057952454 ) ) ;
#89367=CARTESIAN_POINT ( 'NONE',  ( 37.99999999999999289, 2.428612866367529932E-14, -25.00000000000000000 ) ) ;
#89390=CARTESIAN_POINT ( 'NONE',  ( 4.999999999999999112, 11.45643923738960090, -18.00000000000000000 ) ) ;
#89424=ORIENTED_EDGE ( 'NONE', *, *, #49003, .T. ) ;
#89447=EDGE_CURVE ( 'NONE', #1233, #171664, #187476, .T. ) ;
#89530=CARTESIAN_POINT ( 'NONE',  ( -31.74953202133205110, -24.33172034662469940, -19.41189923848662247 ) ) ;
#89537=EDGE_CURVE ( 'NONE', #45261, #165759, #9807, .T. ) ;
#89541=CARTESIAN_POINT ( 'NONE',  ( -4.000000000000000888, -105.0000000000000000, 12.00000000000000355 ) ) ;
#89549=CARTESIAN_POINT ( 'NONE',  ( 11.23063180226361091, -38.81524874329667796, -25.08899775095413531 ) ) ;
#89551=LINE ( 'NONE', #58224, #134099 ) ;
#89622=AXIS2_PLACEMENT_3D ( 'NONE', #3037, #93045, #154732 ) ;
#89630=CARTESIAN_POINT ( 'NONE',  ( 37.66961640367472341, -4.999999999999976019, -15.00000000000000000 ) ) ;
#89639=ADVANCED_FACE ( 'NONE', ( #23763, #101584 ), #26769, .T. ) ;
#89664=VERTEX_POINT ( 'NONE', #148107 ) ;
#89684=CARTESIAN_POINT ( 'NONE',  ( -1.304248841091933035E-15, -21.30000000000002913, -58.85720012050612837 ) ) ;
#89720=CARTESIAN_POINT ( 'NONE',  ( -16.93990830356624855, 14.81572341150380012, -55.62237631978509711 ) ) ;
#89738=CARTESIAN_POINT ( 'NONE',  ( -19.99604614807126524, -21.49604614807088154, -64.92279855667830191 ) ) ;
#89754=LINE ( 'NONE', #195971, #163881 ) ;
#89768=ORIENTED_EDGE ( 'NONE', *, *, #134940, .T. ) ;
#89770=VERTEX_POINT ( 'NONE', #165275 ) ;
#89772=CYLINDRICAL_SURFACE ( 'NONE', #121368, 1.499999999999996225 ) ;
#89776=CARTESIAN_POINT ( 'NONE',  ( -11.40812507854755609, 35.11059874428196537, -3.524999997268813523 ) ) ;
#89826=VERTEX_POINT ( 'NONE', #164284 ) ;
#89829=CARTESIAN_POINT ( 'NONE',  ( 36.91746824999999177, 2.880721459617395097E-14, -8.124999997268814056 ) ) ;
#89844=ORIENTED_EDGE ( 'NONE', *, *, #52535, .F. ) ;
#89850=CARTESIAN_POINT ( 'NONE',  ( -30.87493573979928385, -25.21320017017148984, -21.56479137964121406 ) ) ;
#89851=ORIENTED_EDGE ( 'NONE', *, *, #16988, .F. ) ;
#89877=CARTESIAN_POINT ( 'NONE',  ( 6.853560127763690168, -1.304723572972866119, -64.38700459888464422 ) ) ;
#89908=B_SPLINE_CURVE_WITH_KNOTS ( 'NONE', 3,
 ( #121300, #29313, #166836, #133491, #195183, #120307, #58641, #164843, #26339, #152630, #182000, #89976, #151657, #14120, #104158, #165839, #199145, #197176, #73835, #59626, #122286, #135506, #43483, #183975, #45461, #105150 ),
 .UNSPECIFIED., .F., .F.,
 ( 4, 2, 2, 2, 2, 2, 2, 2, 2, 2, 2, 2, 4 ),
 ( 2.788259459799404871E-07, 0.0002964138711649451233, 0.0005925489163839094348, 0.0008886839616028737463, 0.001184819006821837733, 0.001777089097259766572, 0.002369359187697695195, 0.002665494232916662543, 0.002961629278135629890, 0.003257764323354597237, 0.003553899368573564151, 0.004146169459011502315, 0.004738439549449439611 ),
 .UNSPECIFIED. ) ;
#89976=CARTESIAN_POINT ( 'NONE',  ( -6.132035242901182848, 4.065169771515680708, -62.28151743970310861 ) ) ;
#89983=DIRECTION ( 'NONE',  ( -0.000000000000000000, -0.000000000000000000, 1.000000000000000000 ) ) ;
#90014=EDGE_LOOP ( 'NONE', ( #188540, #84317, #92195, #142356 ) ) ;
#90016=CARTESIAN_POINT ( 'NONE',  ( -7.215019197202725110, 1.452998035947277833, -62.28058590214430268 ) ) ;
#90023=DIRECTION ( 'NONE',  ( 1.000000000000000000, 0.000000000000000000, 0.000000000000000000 ) ) ;
#90031=EDGE_CURVE ( 'NONE', #42534, #157648, #10598, .T. ) ;
#90039=CARTESIAN_POINT ( 'NONE',  ( 0.000000000000000000, 0.000000000000000000, -65.00100000000003320 ) ) ;
#90044=CARTESIAN_POINT ( 'NONE',  ( -4.288219549287815902, -6.449757054545090185, -64.24412156979190058 ) ) ;
#90131=ORIENTED_EDGE ( 'NONE', *, *, #7790, .F. ) ;
#90146=AXIS2_PLACEMENT_3D ( 'NONE', #30575, #92226, #153912 ) ;
#90162=CARTESIAN_POINT ( 'NONE',  ( -38.00000000000000711, 2.428612866367529932E-14, -3.749999994537626780 ) ) ;
#90168=CARTESIAN_POINT ( 'NONE',  ( -6.853560127763669740, 1.304723572972908086, -64.38700459888461580 ) ) ;
#90258=CARTESIAN_POINT ( 'NONE',  ( 15.61223984149541799, -14.70183385125136333, -58.76599187376303490 ) ) ;
#90261=CARTESIAN_POINT ( 'NONE',  ( 14.02111363790003828, -0.9482109960935805049, -60.30654223653039736 ) ) ;
#90263=CARTESIAN_POINT ( 'NONE',  ( 39.99999999999999289, 2.428612866367529932E-14, 0.000000000000000000 ) ) ;
#90279=CARTESIAN_POINT ( 'NONE',  ( 3.766062262543149401E-15, -39.95556452105413570, -7.500000000000000888 ) ) ;
#90332=ORIENTED_EDGE ( 'NONE', *, *, #7594, .T. ) ;
#90391=EDGE_CURVE ( 'NONE', #71084, #74970, #126109, .T. ) ;
#90413=DIRECTION ( 'NONE',  ( 0.000000000000000000, 0.000000000000000000, -1.000000000000000000 ) ) ;
#90421=CARTESIAN_POINT ( 'NONE',  ( 14.98214168267148949, 15.14060719587546622, -56.46919128290397794 ) ) ;
#90463=ORIENTED_EDGE ( 'NONE', *, *, #196878, .T. ) ;
#90468=AXIS2_PLACEMENT_3D ( 'NONE', #15297, #13317, #105320 ) ;
#90474=CARTESIAN_POINT ( 'NONE',  ( -23.57492084471414628, -29.96337447969917633, -16.79025860371109502 ) ) ;
#90513=CARTESIAN_POINT ( 'NONE',  ( -5.950531402560715689E-15, 38.81732327939063509, -7.124999997268814056 ) ) ;
#90520=EDGE_LOOP ( 'NONE', ( #12191, #161221, #105072, #76889 ) ) ;
#90531=CARTESIAN_POINT ( 'NONE',  ( 4.755560754627824238, -48.37114524149939854, -25.00000000000000000 ) ) ;
#90589=DIRECTION ( 'NONE',  ( 0.000000000000000000, 0.000000000000000000, 1.000000000000000000 ) ) ;
#90607=VECTOR ( 'NONE', #119761, 1000.000000000000000 ) ;
#90650=FILL_AREA_STYLE ('',( #119028 ) ) ;
#90658=EDGE_CURVE ( 'NONE', #102786, #4269, #98436, .T. ) ;
#90699=DIRECTION ( 'NONE',  ( 1.000000000000000000, 0.000000000000000000, 0.000000000000000000 ) ) ;
#90732=CARTESIAN_POINT ( 'NONE',  ( -0.9482109960935514170, -14.02111363790006138, -60.30654223653038315 ) ) ;
#90738=CARTESIAN_POINT ( 'NONE',  ( 9.909549000311971056, -9.465176804199456839, -60.44446360152741704 ) ) ;
#90750=B_SPLINE_CURVE_WITH_KNOTS ( 'NONE', 3,
 ( #101037, #147567, #67712, #10054 ),
 .UNSPECIFIED., .F., .F.,
 ( 4, 4 ),
 ( -3.069853556319535759E-05, 0.003328242942582103868 ),
 .UNSPECIFIED. ) ;
#90754=CARTESIAN_POINT ( 'NONE',  ( 11.74264578624800315, -36.14014761921581709, -11.14999999453762669 ) ) ;
#90802=DIRECTION ( 'NONE',  ( 0.000000000000000000, 0.000000000000000000, 1.000000000000000000 ) ) ;
#90806=CARTESIAN_POINT ( 'NONE',  ( 0.1105433493105908715, 24.30000000000003268, -56.77278709839600879 ) ) ;
#90817=EDGE_LOOP ( 'NONE', ( #3289, #133837, #22392, #184844 ) ) ;
#90824=EDGE_LOOP ( 'NONE', ( #43402, #152144, #159960, #149453 ) ) ;
#90868=CARTESIAN_POINT ( 'NONE',  ( 3.735172737399431091E-16, 6.100000000000006750, -64.53213882399991519 ) ) ;
#90943=CARTESIAN_POINT ( 'NONE',  ( 37.99999999999999289, 2.893978650043524126E-14, -7.000000000000000000 ) ) ;
#90947=CARTESIAN_POINT ( 'NONE',  ( -22.99713674769915173, 21.42625476241829219, -46.35568673344857160 ) ) ;
#90985=CARTESIAN_POINT ( 'NONE',  ( -9.021779378622673207, 0.4881926659582808137, -61.91041879129566183 ) ) ;
#90994=( BOUNDED_SURFACE ( )  B_SPLINE_SURFACE ( 1, 2, ( 
 ( #33317, #160629, #142472, #98938, #188006, #190971, #128285, #79814, #49476, #172829, #4937, #52448, #34308, #157655, #20121, #114105, #81765, #80794, #66621, #37281, #145450, #189002, #50477, #143452, #165634, #25140, #103955, #70627, #56455, #150472, #27132, #69621, #118134, #147469, #148467, #100940, #40283, #196975, #24131, #23122, #38288, #119136, #134305, #88779, #9960, #84767, #11967, #73632, #8959, #55448, #135303, #7938, #54454, #179823, #85783, #146445, #101957, #178813, #131287, #115123, #192975, #161628, #117119, #86782, #177813, #180816, #71620, #176816, #194976, #132294, #193986, #99942, #116124, #39283, #162624, #133286, #72630, #163638, #41293, #102954, #164638, #26133, #87776, #149461, #10956, #195991, #57464, #42295, #198952, #43279, #729, #123083, #140240, #153431, #90754, #139253, #61412, #152437, #76589, #13923, #138265 ),
 ( #155424, #62401, #124071, #58442, #197956, #75590, #184769, #77581, #74614, #166634, #185772, #120110, #28136, #122092, #104948, #45269, #16914, #47259, #181800, #183783, #106923, #78567, #108916, #154429, #89776, #151461, #107909, #15923, #170596, #168596, #12949, #137269, #30096, #136280, #14929, #59425, #60419, #91735, #32086, #199948, #46255, #169595, #31093, #92741, #93743, #121099, #182793, #44276, #105934, #167619, #29115, #142230, #143217, #18910, #19889, #158400, #112886, #109908, #144220, #4698, #187772, #95730, #35057, #173588, #96712, #49242, #65392, #36045, #33080, #3715, #110900, #157416, #141241, #172585, #127053, #125086, #63411, #34072, #81530, #66389, #174580, #80555, #5704, #188759, #50244, #82538, #111900, #156415, #128051, #189753, #51225, #97694, #159385, #20880, #67381, #1733, #186784, #2730, #48254, #171592, #94736 ) ),
 .UNSPECIFIED., .F., .F., .F. ) 
 B_SPLINE_SURFACE_WITH_KNOTS ( ( 2, 2 ),
 ( 3, 2, 2, 2, 2, 2, 2, 2, 2, 2, 2, 2, 2, 2, 2, 2, 2, 2, 2, 2, 2, 2, 2, 2, 2, 2, 2, 2, 2, 2, 2, 2, 2, 2, 2, 2, 2, 2, 2, 2, 2, 2, 2, 2, 2, 2, 2, 2, 2, 2, 3 ),
 ( 0.000000000000000000, 1.000000000000000000 ),
 ( 0.000000000000000000, 0.02000000000000000042, 0.04000000000000000083, 0.05999999999999999778, 0.08000000000000000167, 0.1000000000000000056, 0.1199999999999999956, 0.1400000000000000133, 0.1600000000000000033, 0.1799999999999999933, 0.2000000000000000111, 0.2200000000000000011, 0.2399999999999999911, 0.2600000000000000089, 0.2800000000000000266, 0.2999999999999999889, 0.3200000000000000067, 0.3400000000000000244, 0.3599999999999999867, 0.3800000000000000044, 0.4000000000000000222, 0.4199999999999999845, 0.4400000000000000022, 0.4600000000000000200, 0.4799999999999999822, 0.5000000000000000000, 0.5200000000000000178, 0.5400000000000000355, 0.5600000000000000533, 0.5799999999999999600, 0.5999999999999999778, 0.6199999999999999956, 0.6400000000000000133, 0.6600000000000000311, 0.6800000000000000488, 0.6999999999999999556, 0.7199999999999999734, 0.7399999999999999911, 0.7600000000000000089, 0.7800000000000000266, 0.8000000000000000444, 0.8199999999999999512, 0.8399999999999999689, 0.8599999999999999867, 0.8800000000000000044, 0.9000000000000000222, 0.9200000000000000400, 0.9399999999999999467, 0.9599999999999999645, 0.9799999999999999822, 1.000000000000000000 ),
 .UNSPECIFIED. ) 
 GEOMETRIC_REPRESENTATION_ITEM ( )  RATIONAL_B_SPLINE_SURFACE ( (
 ( 1.000000000000000000, 0.9510565162951535312, 1.000000000000000000, 0.9510565162951535312, 1.000000000000000000, 0.9510565162951535312, 1.000000000000000000, 0.9510565162951535312, 1.000000000000000000, 0.9510565162951535312, 1.000000000000000000, 0.9510565162951535312, 1.000000000000000000, 0.9510565162951535312, 1.000000000000000000, 0.9510565162951535312, 1.000000000000000000, 0.9510565162951535312, 1.000000000000000000, 0.9510565162951535312, 1.000000000000000000, 0.9510565162951535312, 1.000000000000000000, 0.9510565162951535312, 1.000000000000000000, 0.9510565162951535312, 1.000000000000000000, 0.9510565162951535312, 1.000000000000000000, 0.9510565162951535312, 1.000000000000000000, 0.9510565162951535312, 1.000000000000000000, 0.9510565162951535312, 1.000000000000000000, 0.9510565162951535312, 1.000000000000000000, 0.9510565162951535312, 1.000000000000000000, 0.9510565162951535312, 1.000000000000000000, 0.9510565162951535312, 1.000000000000000000, 0.9510565162951535312, 1.000000000000000000, 0.9510565162951535312, 1.000000000000000000, 0.9510565162951535312, 1.000000000000000000, 0.9510565162951535312, 1.000000000000000000, 0.9510565162951535312, 1.000000000000000000, 0.9510565162951535312, 1.000000000000000000, 0.9510565162951535312, 1.000000000000000000, 0.9510565162951535312, 1.000000000000000000, 0.9510565162951535312, 1.000000000000000000, 0.9510565162951535312, 1.000000000000000000, 0.9510565162951535312, 1.000000000000000000, 0.9510565162951535312, 1.000000000000000000, 0.9510565162951535312, 1.000000000000000000, 0.9510565162951535312, 1.000000000000000000, 0.9510565162951535312, 1.000000000000000000, 0.9510565162951535312, 1.000000000000000000, 0.9510565162951535312, 1.000000000000000000, 0.9510565162951535312, 1.000000000000000000, 0.9510565162951535312, 1.000000000000000000, 0.9510565162951535312, 1.000000000000000000, 0.9510565162951535312, 1.000000000000000000, 0.9510565162951535312, 1.000000000000000000, 0.9510565162951535312, 1.000000000000000000, 0.9510565162951535312, 1.000000000000000000, 0.9510565162951535312, 1.000000000000000000, 0.9510565162951535312, 1.000000000000000000, 0.9510565162951535312, 1.000000000000000000, 0.9510565162951535312, 1.000000000000000000, 0.9510565162951535312, 1.000000000000000000),
 ( 1.000000000000000000, 0.9510565162951535312, 1.000000000000000000, 0.9510565162951535312, 1.000000000000000000, 0.9510565162951535312, 1.000000000000000000, 0.9510565162951535312, 1.000000000000000000, 0.9510565162951535312, 1.000000000000000000, 0.9510565162951535312, 1.000000000000000000, 0.9510565162951535312, 1.000000000000000000, 0.9510565162951535312, 1.000000000000000000, 0.9510565162951535312, 1.000000000000000000, 0.9510565162951535312, 1.000000000000000000, 0.9510565162951535312, 1.000000000000000000, 0.9510565162951535312, 1.000000000000000000, 0.9510565162951535312, 1.000000000000000000, 0.9510565162951535312, 1.000000000000000000, 0.9510565162951535312, 1.000000000000000000, 0.9510565162951535312, 1.000000000000000000, 0.9510565162951535312, 1.000000000000000000, 0.9510565162951535312, 1.000000000000000000, 0.9510565162951535312, 1.000000000000000000, 0.9510565162951535312, 1.000000000000000000, 0.9510565162951535312, 1.000000000000000000, 0.9510565162951535312, 1.000000000000000000, 0.9510565162951535312, 1.000000000000000000, 0.9510565162951535312, 1.000000000000000000, 0.9510565162951535312, 1.000000000000000000, 0.9510565162951535312, 1.000000000000000000, 0.9510565162951535312, 1.000000000000000000, 0.9510565162951535312, 1.000000000000000000, 0.9510565162951535312, 1.000000000000000000, 0.9510565162951535312, 1.000000000000000000, 0.9510565162951535312, 1.000000000000000000, 0.9510565162951535312, 1.000000000000000000, 0.9510565162951535312, 1.000000000000000000, 0.9510565162951535312, 1.000000000000000000, 0.9510565162951535312, 1.000000000000000000, 0.9510565162951535312, 1.000000000000000000, 0.9510565162951535312, 1.000000000000000000, 0.9510565162951535312, 1.000000000000000000, 0.9510565162951535312, 1.000000000000000000, 0.9510565162951535312, 1.000000000000000000, 0.9510565162951535312, 1.000000000000000000, 0.9510565162951535312, 1.000000000000000000, 0.9510565162951535312, 1.000000000000000000, 0.9510565162951535312, 1.000000000000000000, 0.9510565162951535312, 1.000000000000000000, 0.9510565162951535312, 1.000000000000000000, 0.9510565162951535312, 1.000000000000000000, 0.9510565162951535312, 1.000000000000000000, 0.9510565162951535312, 1.000000000000000000, 0.9510565162951535312, 1.000000000000000000) ) ) 
 REPRESENTATION_ITEM ( '' )  SURFACE ( )  );
#91014=CARTESIAN_POINT ( 'NONE',  ( -3.874011537017660434, -5.521060904931721858, -64.42755313133395134 ) ) ;
#91019=ORIENTED_EDGE ( 'NONE', *, *, #50162, .F. ) ;
#91038=CARTESIAN_POINT ( 'NONE',  ( -6.686840650406351116, 6.126184129041750914, -63.95889547717843726 ) ) ;
#91069=CARTESIAN_POINT ( 'NONE',  ( 11.30153831258471797, -180.0000000000000000, -15.00000000000000178 ) ) ;
#91219=CARTESIAN_POINT ( 'NONE',  ( -23.48529157249600985, 32.32473071737754111, -6.049999994537626158 ) ) ;
#91229=CARTESIAN_POINT ( 'NONE',  ( -0.4346045811322798991, -24.23981148858511503, -54.26183423998840993 ) ) ;
#91239=LINE ( 'NONE', #137766, #88460 ) ;
#91244=VERTEX_POINT ( 'NONE', #139863 ) ;
#91247=CARTESIAN_POINT ( 'NONE',  ( -30.74264578624800492, 22.33583958711400186, -4.200000000000000178 ) ) ;
#91273=CARTESIAN_POINT ( 'NONE',  ( 7.213464565009756413, -38.12638803158730383, -24.00445952849677056 ) ) ;
#91315=EDGE_CURVE ( 'NONE', #138197, #164346, #87298, .T. ) ;
#91338=ADVANCED_FACE ( 'NONE', ( #24276 ), #187404, .F. ) ;
#91392=CARTESIAN_POINT ( 'NONE',  ( -22.55670631985108443, -22.55670631985069008, -49.13275782002545355 ) ) ;
#91413=B_SPLINE_CURVE_WITH_KNOTS ( 'NONE', 3,
 ( #49441, #109119, #139449, #930, #170797, #155623 ),
 .UNSPECIFIED., .F., .F.,
 ( 4, 2, 4 ),
 ( 0.003562460574610347517, 0.004150450062026994624, 0.004738439549443641298 ),
 .UNSPECIFIED. ) ;
#91430=EDGE_LOOP ( 'NONE', ( #107694, #9658, #111603, #10949 ) ) ;
#91443=CARTESIAN_POINT ( 'NONE',  ( -20.47606263883548294, -31.78721852327825914, -20.08103504831861130 ) ) ;
#91467=CARTESIAN_POINT ( 'NONE',  ( 20.76286210753433181, -20.18345802296806113, -49.60777730575491518 ) ) ;
#91481=ORIENTED_EDGE ( 'NONE', *, *, #16720, .F. ) ;
#91485=CARTESIAN_POINT ( 'NONE',  ( -5.950531402560715689E-15, 38.81732327939063509, -9.124999997268814056 ) ) ;
#91495=DIRECTION ( 'NONE',  ( 0.000000000000000000, 0.000000000000000000, 1.000000000000000000 ) ) ;
#91505=CARTESIAN_POINT ( 'NONE',  ( -10.41657218803457674, -12.21822558928538172, -61.63650692604122838 ) ) ;
#91512=EDGE_CURVE ( 'NONE', #172040, #167830, #17536, .T. ) ;
#91522=ORIENTED_EDGE ( 'NONE', *, *, #91752, .T. ) ;
#91544=VECTOR ( 'NONE', #69994, 1000.000000000000000 ) ;
#91547=ORIENTED_EDGE ( 'NONE', *, *, #9668, .F. ) ;
#91606=AXIS2_PLACEMENT_3D ( 'NONE', #172234, #95381, #157067 ) ;
#91628=LINE ( 'NONE', #156301, #8039 ) ;
#91683=EDGE_CURVE ( 'NONE', #152430, #1611, #145595, .T. ) ;
#91684=VECTOR ( 'NONE', #153190, 1000.000000000000000 ) ;
#91696=CARTESIAN_POINT ( 'NONE',  ( 22.55670631985092456, -22.55670631985084995, -45.64921306006598201 ) ) ;
#91698=LINE ( 'NONE', #153391, #63203 ) ;
#91720=CARTESIAN_POINT ( 'NONE',  ( 0.4308872995781310444, 21.35919609616788506, -58.81731666137213210 ) ) ;
#91735=CARTESIAN_POINT ( 'NONE',  ( -22.81625015709509441, -31.40387420917324590, -4.824999997268813345 ) ) ;
#91736=AXIS2_PLACEMENT_3D ( 'NONE', #70127, #131799, #150973 ) ;
#91748=CARTESIAN_POINT ( 'NONE',  ( 12.21174782391248392, -11.13111847464308468, -59.22005018971564283 ) ) ;
#91752=EDGE_CURVE ( 'NONE', #25387, #38805, #38431, .T. ) ;
#91759=CARTESIAN_POINT ( 'NONE',  ( -21.31248648291600389, 0.2211803504531069942, -58.84879416108404371 ) ) ;
#91784=CARTESIAN_POINT ( 'NONE',  ( -3.503282210674363295, -48.86437366581481001, -25.00000000000000000 ) ) ;
#91787=DIRECTION ( 'NONE',  ( -0.000000000000000000, 0.000000000000000000, 1.000000000000000000 ) ) ;
#91912=CARTESIAN_POINT ( 'NONE',  ( 1.452840677238310674, 7.214434113892650657, -62.28070517238707282 ) ) ;
#91940=CARTESIAN_POINT ( 'NONE',  ( -10.74802307403563084, -10.74802307403544077, -64.92279855667830191 ) ) ;
#91974=CARTESIAN_POINT ( 'NONE',  ( -6.854124442541994711, 1.305043071815353395, -62.35408385982739077 ) ) ;
#91988=CIRCLE ( 'NONE', #146850, 214.0437394197456342 ) ;
#92092=VECTOR ( 'NONE', #152148, 1000.000000000000000 ) ;
#92099=CARTESIAN_POINT ( 'NONE',  ( 0.000000000000000000, 0.000000000000000000, -56.46919128290398504 ) ) ;
#92114=FACE_OUTER_BOUND ( 'NONE', #26945, .T. ) ;
#92134=DIRECTION ( 'NONE',  ( -1.000000000000000000, 0.000000000000000000, 0.000000000000000000 ) ) ;
#92141=CARTESIAN_POINT ( 'NONE',  ( -9.021937450273798120, 0.4877194249721380492, -63.96635223026897421 ) ) ;
#92144=DIRECTION ( 'NONE',  ( 0.000000000000000000, 0.000000000000000000, 1.000000000000000000 ) ) ;
#92179=SHAPE_REPRESENTATION ( 'Rear Air Intake Grille & Cap', ( #82054 ), #24091 ) ;
#92192=VERTEX_POINT ( 'NONE', #165779 ) ;
#92195=ORIENTED_EDGE ( 'NONE', *, *, #68319, .F. ) ;
#92196=ORIENTED_EDGE ( 'NONE', *, *, #188361, .T. ) ;
#92226=DIRECTION ( 'NONE',  ( -0.000000000000000000, 0.000000000000000000, 1.000000000000000000 ) ) ;
#92233=CARTESIAN_POINT ( 'NONE',  ( 28.90000000000004476, 0.000000000000000000, -52.65483682830183199 ) ) ;
#92246=AXIS2_PLACEMENT_3D ( 'NONE', #159313, #144150, #162324 ) ;
#92250=EDGE_CURVE ( 'NONE', #164346, #515, #27274, .T. ) ;
#92258=CARTESIAN_POINT ( 'NONE',  ( 37.99999999999999289, 2.893978650043524126E-14, -7.000000000000000000 ) ) ;
#92263=CYLINDRICAL_SURFACE ( 'NONE', #192437, 38.00000000000000000 ) ;
#92284=CARTESIAN_POINT ( 'NONE',  ( 11.44429459766798729, -35.82063519324240275, -30.53178620540658983 ) ) ;
#92289=ORIENTED_EDGE ( 'NONE', *, *, #163088, .F. ) ;
#92398=DIRECTION ( 'NONE',  ( 0.000000000000000000, 0.000000000000000000, -1.000000000000000000 ) ) ;
#92435=( BOUNDED_CURVE ( )  B_SPLINE_CURVE ( 2, ( #8210, #176074, #22386, #68880, #116384, #129532, #147737, #158885, #37542, #53718, #6199 ),
 .UNSPECIFIED., .F., .T. ) 
 B_SPLINE_CURVE_WITH_KNOTS ( ( 3, 2, 2, 2, 2, 3 ),
 ( 0.3000000000000000444, 0.3200000000000000622, 0.3400000000000000799, 0.3599999999999999867, 0.3800000000000000044, 0.4000000000000000222 ),
 .UNSPECIFIED. ) 
 CURVE ( )  GEOMETRIC_REPRESENTATION_ITEM ( )  RATIONAL_B_SPLINE_CURVE ( ( 0.9999999999999998890, 0.9510565162951536422, 1.000000000000000000, 0.9510565162951535312, 1.000000000000000000, 0.9510565162951535312, 1.000000000000000000, 0.9510565162951535312, 1.000000000000000000, 0.9510565162951535312, 1.000000000000000000 ) ) 
 REPRESENTATION_ITEM ( '' )  );
#92449=CARTESIAN_POINT ( 'NONE',  ( -12.81081878835845522, -36.21111560917540828, -23.25335493477762583 ) ) ;
#92472=FACE_OUTER_BOUND ( 'NONE', #163714, .T. ) ;
#92509=CARTESIAN_POINT ( 'NONE',  ( 2.919401842228637189, -40.72031138817901308, -24.99999999999999645 ) ) ;
#92528=ORIENTED_EDGE ( 'NONE', *, *, #161100, .T. ) ;
#92542=AXIS2_PLACEMENT_3D ( 'NONE', #110196, #142520, #111187 ) ;
#92552=EDGE_LOOP ( 'NONE', ( #183300, #108372, #25966, #28909 ) ) ;
#92563=CARTESIAN_POINT ( 'NONE',  ( -10.74802307403563084, -10.74802307403544077, -64.92279855667830191 ) ) ;
#92592=CARTESIAN_POINT ( 'NONE',  ( -69.65682714487590488, -71.74905178543390605, -15.00000000000000178 ) ) ;
#92638=VECTOR ( 'NONE', #132949, 1000.000000000000000 ) ;
#92725=CARTESIAN_POINT ( 'NONE',  ( -20.02040504322455305, -21.79936378052101631, -48.83307992000326436 ) ) ;
#92741=CARTESIAN_POINT ( 'NONE',  ( -22.81625015709510507, 31.40387420917330275, -5.424999997268812990 ) ) ;
#92754=CARTESIAN_POINT ( 'NONE',  ( 5.563226388833935943, 6.875118674992778622, -61.95704554880761350 ) ) ;
#92778=CARTESIAN_POINT ( 'NONE',  ( 37.99999999999999289, 12.34694845685046793, -8.899999999999996803 ) ) ;
#92793=CARTESIAN_POINT ( 'NONE',  ( -11.30153831258470731, -190.0000000000000000, 0.000000000000000000 ) ) ;
#92800=CARTESIAN_POINT ( 'NONE',  ( -10.97407593764241618, 9.252314257645080531, -62.33638803020407693 ) ) ;
#92815=CARTESIAN_POINT ( 'NONE',  ( -32.28837973138505646, -23.54499195901729180, -23.03346093386547722 ) ) ;
#92816=ORIENTED_EDGE ( 'NONE', *, *, #16747, .F. ) ;
#92936=CARTESIAN_POINT ( 'NONE',  ( -5.000000000000003553, -4.999999999999996447, -18.00000000000000000 ) ) ;
#92940=CARTESIAN_POINT ( 'NONE',  ( -4.647474457565486646E-15, 28.90000000000004476, -49.67367017693150189 ) ) ;
#92944=CARTESIAN_POINT ( 'NONE',  ( -22.62812085840268495, 1.500606516337707586, -55.49205433527804132 ) ) ;
#92980=CARTESIAN_POINT ( 'NONE',  ( 27.86273085795036408, -28.69962071417356242, -15.00000000000000178 ) ) ;
#93039=CARTESIAN_POINT ( 'NONE',  ( -6.259396865588131575, -47.62116666102458851, -24.77619460540839569 ) ) ;
#93045=DIRECTION ( 'NONE',  ( 0.000000000000000000, 0.000000000000000000, 1.000000000000000000 ) ) ;
#93080=CARTESIAN_POINT ( 'NONE',  ( -14.01879992551667442, 0.9453496423220366651, -62.45159313300388959 ) ) ;
#93083=VECTOR ( 'NONE', #162641, 1000.000000000000000 ) ;
#93194=EDGE_LOOP ( 'NONE', ( #188218, #74139, #198885, #10789, #187345, #51917, #37500, #134296, #38599, #4818, #179524, #164864, #143939, #183777 ) ) ;
#93230=CARTESIAN_POINT ( 'NONE',  ( -0.7284999611695081034, -24.11542121825891627, -54.35861002160294930 ) ) ;
#93235=FACE_BOUND ( 'NONE', #90817, .T. ) ;
#93240=CARTESIAN_POINT ( 'NONE',  ( -15.40597107458654591, 14.79957802611868978, -58.81775317265829273 ) ) ;
#93266=EDGE_CURVE ( 'NONE', #102786, #186567, #160537, .T. ) ;
#93275=CARTESIAN_POINT ( 'NONE',  ( 16.98531384169471892, -34.11756901830160160, -21.70785296103238693 ) ) ;
#93302=ORIENTED_EDGE ( 'NONE', *, *, #161479, .T. ) ;
#93345=CARTESIAN_POINT ( 'NONE',  ( 6.404810000729014519, -0.9277198534072479408, -62.44539631020982284 ) ) ;
#93364=CARTESIAN_POINT ( 'NONE',  ( 1.106442667531312596, 31.41700946213341794, -49.73385396542428794 ) ) ;
#93441=CARTESIAN_POINT ( 'NONE',  ( -22.01160362601145337, -30.88790364210668926, -22.63296439182591513 ) ) ;
#93458=B_SPLINE_CURVE_WITH_KNOTS ( 'NONE', 3,
 ( #191711, #159367, #189737, #5689, #18896, #173574, #99696 ),
 .UNSPECIFIED., .F., .F.,
 ( 4, 3, 4 ),
 ( 0.006877813788783031929, 0.01375562809188913063, 0.01380070845639008031 ),
 .UNSPECIFIED. ) ;
#93473=CARTESIAN_POINT ( 'NONE',  ( 6.835613355214110953, -5.764477180739371320, -63.98825660581650254 ) ) ;
#93484=AXIS2_PLACEMENT_3D ( 'NONE', #54650, #55652, #116324 ) ;
#93490=EDGE_LOOP ( 'NONE', ( #176088, #137628, #58007, #56797 ) ) ;
#93493=LINE ( 'NONE', #30853, #7379 ) ;
#93502=DIRECTION ( 'NONE',  ( 1.000000000000000000, 0.000000000000000000, 3.469446951953612217E-15 ) ) ;
#93504=CARTESIAN_POINT ( 'NONE',  ( 15.53529872673065704, -37.10890965030476707, -23.64498726423094510 ) ) ;
#93562=CARTESIAN_POINT ( 'NONE',  ( 38.00000000000001421, 12.34694845685043951, -2.900000000000000799 ) ) ;
#93721=FACE_BOUND ( 'NONE', #24848, .T. ) ;
#93727=CARTESIAN_POINT ( 'NONE',  ( 1.243777456120027214, 21.93922656192045650, -58.42410701432510223 ) ) ;
#93735=VERTEX_POINT ( 'NONE', #89684 ) ;
#93737=ORIENTED_EDGE ( 'NONE', *, *, #195370, .F. ) ;
#93739=DIRECTION ( 'NONE',  ( 1.000000000000000000, 0.000000000000000000, 0.000000000000000000 ) ) ;
#93743=CARTESIAN_POINT ( 'NONE',  ( -11.40812507854755609, 35.11059874428196537, -5.524999997268813523 ) ) ;
#93756=CARTESIAN_POINT ( 'NONE',  ( 3.873512393789732222, 5.284191517680363326, -62.43104308550748982 ) ) ;
#93779=CARTESIAN_POINT ( 'NONE',  ( 30.74264578624799782, 22.33583958711400541, -8.800000000000000711 ) ) ;
#93790=CARTESIAN_POINT ( 'NONE',  ( -38.00000000000000711, 2.428612866367529932E-14, -11.74999999453762634 ) ) ;
#93793=CARTESIAN_POINT ( 'NONE',  ( 36.91746824999999887, 11.99521256947799053, -6.024999997268811747 ) ) ;
#93794=CARTESIAN_POINT ( 'NONE',  ( 0.5319425161145064918, 24.20639721642469411, -56.83990048018080188 ) ) ;
#93801=CARTESIAN_POINT ( 'NONE',  ( 16.49801837613234667, -34.15639402546909764, -27.41207208920353011 ) ) ;
#93860=VERTEX_POINT ( 'NONE', #59332 ) ;
#93910=VERTEX_POINT ( 'NONE', #27040 ) ;
#93919=CARTESIAN_POINT ( 'NONE',  ( 1.136082944010448514, 6.615573198874504790, -62.40258669366784972 ) ) ;
#93938=LINE ( 'NONE', #17113, #41859 ) ;
#93942=CARTESIAN_POINT ( 'NONE',  ( -21.30378117525442860, 19.99074948409473862, -49.30207733784024526 ) ) ;
#93944=CARTESIAN_POINT ( 'NONE',  ( -21.39623730026198700, 0.5392447798058846997, -56.39940532337661239 ) ) ;
#93987=CARTESIAN_POINT ( 'NONE',  ( 19.97888994334919843, -34.65319547504301312, -10.00000000000000000 ) ) ;
#94067=B_SPLINE_CURVE_WITH_KNOTS ( 'NONE', 3,
 ( #28621, #198446, #105436, #90258, #12461, #135792, #165135, #149958, #147969, #197463, #133790, #120597, #167121, #180322 ),
 .UNSPECIFIED., .F., .F.,
 ( 4, 2, 2, 2, 2, 2, 4 ),
 ( 2.784816081883512217E-07, 0.0004992641294407349547, 0.0009982497772732814266, 0.001996221072938393019, 0.002994192368603504611, 0.003493178016436066045, 0.003992163664268632249 ),
 .UNSPECIFIED. ) ;
#94095=DIRECTION ( 'NONE',  ( 1.000000000000000000, 0.000000000000000000, 0.000000000000000000 ) ) ;
#94139=CARTESIAN_POINT ( 'NONE',  ( -15.38714178908729124, -36.74766143018473485, -28.97229394964855942 ) ) ;
#94189=VERTEX_POINT ( 'NONE', #79482 ) ;
#94232=FACE_BOUND ( 'NONE', #163939, .T. ) ;
#94237=CARTESIAN_POINT ( 'NONE',  ( -17.61085972261891186, 15.85590801997748756, -57.22569728324523197 ) ) ;
#94272=CARTESIAN_POINT ( 'NONE',  ( 21.54936698786741900, -30.95672727791841439, -19.59590204858815810 ) ) ;
#94386=CARTESIAN_POINT ( 'NONE',  ( -20.38160892792488355, -22.50821459300682648, -51.03861378962740503 ) ) ;
#94422=ORIENTED_EDGE ( 'NONE', *, *, #163088, .T. ) ;
#94437=CARTESIAN_POINT ( 'NONE',  ( -25.98457697381309472, -27.33515243881182144, -20.34861096990052332 ) ) ;
#94460=CARTESIAN_POINT ( 'NONE',  ( 30.74264578624800137, -22.33583958711395212, -9.199999999999999289 ) ) ;
#94486=CARTESIAN_POINT ( 'NONE',  ( 29.86685920354754842, -21.69954338932559068, -5.824999997268813345 ) ) ;
#94496=CARTESIAN_POINT ( 'NONE',  ( 27.35218628822511278, -28.77384467243328459, -20.10380102095120947 ) ) ;
#94515=EDGE_LOOP ( 'NONE', ( #29563, #38581, #38514, #57914 ) ) ;
#94553=( BOUNDED_SURFACE ( )  B_SPLINE_SURFACE ( 3, 2, ( 
 ( #4017, #6009, #53518 ),
 ( #83839, #127360, #38359 ),
 ( #189073, #114176, #8009 ),
 ( #115196, #69692, #173896 ),
 ( #35365, #159691, #193048 ),
 ( #5009, #19212, #131359 ),
 ( #145521, #67689, #39356 ),
 ( #129347, #177887, #175879 ),
 ( #21189, #100014, #54525 ),
 ( #97017, #99009, #82845 ),
 ( #160700, #101015, #7001 ),
 ( #128354, #50545, #191042 ),
 ( #144524, #68683, #130338 ),
 ( #80862, #65695, #158698 ),
 ( #23197, #22191, #176888 ),
 ( #20187, #81833, #143520 ),
 ( #52515, #192036, #66691 ),
 ( #51527, #113190, #174879 ),
 ( #36345, #178888, #197048 ),
 ( #41364, #87846, #163713 ),
 ( #181872, #44347, #166706 ),
 ( #196063, #162700, #42365 ),
 ( #24205, #151533, #103030 ),
 ( #120182, #85854, #150542 ),
 ( #71693, #73706, #132368 ),
 ( #26207, #117195, #70700 ),
 ( #195050, #119205, #147543 ),
 ( #9031, #74687, #194061 ),
 ( #56529, #40356, #135378 ),
 ( #121172, #55522, #104028 ),
 ( #11029, #165707, #148542 ),
 ( #28209, #118207, #102031 ),
 ( #43351, #182866, #25216 ),
 ( #86858, #12042, #59497 ),
 ( #180890, #10033, #133360 ),
 ( #149534, #58516, #27204 ),
 ( #179898, #105022, #164712 ),
 ( #72704, #134377, #57536 ),
 ( #89850, #88850, #13022 ),
 ( #136353, #198029, #62476 ),
 ( #92815, #170670, #125160 ),
 ( #126147, #123155, #15997 ),
 ( #803, #183852, #107982 ),
 ( #17991, #29189, #45340 ) ),
 .UNSPECIFIED., .F., .F., .F. ) 
 B_SPLINE_SURFACE_WITH_KNOTS ( ( 4, 2, 2, 2, 2, 2, 2, 2, 2, 2, 2, 2, 2, 2, 2, 2, 2, 2, 2, 2, 2, 4 ),
 ( 3, 3 ),
 ( 0.1334715276261017047, 0.1400397817209072804, 0.1416818452446086951, 0.1433239087683100821, 0.1466080358157128560, 0.1498921628631156300, 0.1531762899105184039, 0.1564604169579211779, 0.1597445440053239796, 0.1630286710527267813, 0.1646707345764281682, 0.1663127981001295552, 0.1679548616238309422, 0.1695969251475323292, 0.1712389886712337161, 0.1720600204330844096, 0.1728810521949351031, 0.1745231157186364901, 0.1761651792423378771, 0.1794493062897406788, 0.1827334333371434805, 0.1860175603845462544 ),
 ( 0.000000000000000000, 1.000000000000000000 ),
 .UNSPECIFIED. ) 
 GEOMETRIC_REPRESENTATION_ITEM ( )  RATIONAL_B_SPLINE_SURFACE ( (
 ( 1.000000000000000000, 0.7745966692414831822, 1.000000000000000000),
 ( 1.000000000000000000, 0.7873173169477361011, 1.000000000000000000),
 ( 1.000000000000000000, 0.8012080269090376961, 1.000000000000000000),
 ( 1.000000000000000000, 0.8197272276933634805, 1.000000000000000000),
 ( 1.000000000000000000, 0.8234885421913328285, 1.000000000000000000),
 ( 1.000000000000000000, 0.8311157573375301810, 1.000000000000000000),
 ( 1.000000000000000000, 0.8349728938256689714, 1.000000000000000000),
 ( 1.000000000000000000, 0.8465302108191189445, 1.000000000000000000),
 ( 1.000000000000000000, 0.8542644918356308015, 1.000000000000000000),
 ( 1.000000000000000000, 0.8696747091108885108, 1.000000000000000000),
 ( 1.000000000000000000, 0.8773507960692286112, 1.000000000000000000),
 ( 1.000000000000000000, 0.8925002889088409219, 1.000000000000000000),
 ( 1.000000000000000000, 0.8999891582780782384, 1.000000000000000000),
 ( 1.000000000000000000, 0.9145203485641840713, 1.000000000000000000),
 ( 1.000000000000000000, 0.9215166741120195404, 1.000000000000000000),
 ( 1.000000000000000000, 0.9348196634156171747, 1.000000000000000000),
 ( 1.000000000000000000, 0.9411264847295628400, 1.000000000000000000),
 ( 1.000000000000000000, 0.9528821887673051272, 1.000000000000000000),
 ( 1.000000000000000000, 0.9583320463343940609, 1.000000000000000000),
 ( 1.000000000000000000, 0.9657141226242619281, 1.000000000000000000),
 ( 1.000000000000000000, 0.9680424144921330187, 1.000000000000000000),
 ( 1.000000000000000000, 0.9724014971077669101, 1.000000000000000000),
 ( 1.000000000000000000, 0.9744334801158447412, 1.000000000000000000),
 ( 1.000000000000000000, 0.9781204877085358795, 1.000000000000000000),
 ( 1.000000000000000000, 0.9797809101336111270, 1.000000000000000000),
 ( 1.000000000000000000, 0.9826818083352576449, 1.000000000000000000),
 ( 1.000000000000000000, 0.9839230189806436044, 1.000000000000000000),
 ( 1.000000000000000000, 0.9859013487405714482, 1.000000000000000000),
 ( 1.000000000000000000, 0.9866146582094302842, 1.000000000000000000),
 ( 1.000000000000000000, 0.9872250220265940124, 1.000000000000000000),
 ( 1.000000000000000000, 0.9873522598263919647, 1.000000000000000000),
 ( 1.000000000000000000, 0.9874472609175171112, 1.000000000000000000),
 ( 1.000000000000000000, 0.9874138636738953867, 1.000000000000000000),
 ( 1.000000000000000000, 0.9870735186573816877, 1.000000000000000000),
 ( 1.000000000000000000, 0.9865315217161264583, 1.000000000000000000),
 ( 1.000000000000000000, 0.9848873008857174094, 1.000000000000000000),
 ( 1.000000000000000000, 0.9837743821442677117, 1.000000000000000000),
 ( 1.000000000000000000, 0.9797976954002749483, 1.000000000000000000),
 ( 1.000000000000000000, 0.9763000371664851684, 1.000000000000000000),
 ( 1.000000000000000000, 0.9680363503266700143, 1.000000000000000000),
 ( 1.000000000000000000, 0.9632464763793491258, 1.000000000000000000),
 ( 1.000000000000000000, 0.9526889542241591124, 1.000000000000000000),
 ( 1.000000000000000000, 0.9469283804590782339, 1.000000000000000000),
 ( 1.000000000000000000, 0.9407878411039237720, 1.000000000000000000) ) ) 
 REPRESENTATION_ITEM ( '' )  SURFACE ( )  );
#94556=CIRCLE ( 'NONE', #181762, 2.500000000000000000 ) ;
#94585=CARTESIAN_POINT ( 'NONE',  ( 12.24802307403557933, -10.74802307403627921, -61.53034260416801260 ) ) ;
#94644=ADVANCED_FACE ( 'NONE', ( #47695 ), #174022, .F. ) ;
#94659=EDGE_CURVE ( 'NONE', #17478, #151987, #35493, .T. ) ;
#94686=EDGE_CURVE ( 'NONE', #153996, #138940, #177522, .T. ) ;
#94715=FACE_BOUND ( 'NONE', #103238, .T. ) ;
#94721=CARTESIAN_POINT ( 'NONE',  ( -20.56300917109736304, -22.67728815268617737, -47.51549809214670006 ) ) ;
#94731=AXIS2_PLACEMENT_3D ( 'NONE', #7544, #147081, #126901 ) ;
#94736=CARTESIAN_POINT ( 'NONE',  ( -36.91746825000000598, 2.428612866367529932E-14, -11.12499999726881228 ) ) ;
#94783=CARTESIAN_POINT ( 'NONE',  ( -193.3062444957834884, -155.7167183371838064, -15.00000000000000178 ) ) ;
#94786=CARTESIAN_POINT ( 'NONE',  ( -5.950531402560715689E-15, 38.81732327939063509, -7.624999997268814056 ) ) ;
#94823=ORIENTED_EDGE ( 'NONE', *, *, #140691, .T. ) ;
#94857=ORIENTED_EDGE ( 'NONE', *, *, #191573, .T. ) ;
#94898=CYLINDRICAL_SURFACE ( 'NONE', #111837, 12.50000000000000000 ) ;
#94919=PRODUCT_DEFINITION_CONTEXT ( 'detailed design', #88162, 'design' ) ;
#94939=CARTESIAN_POINT ( 'NONE',  ( 9.687362902255733488, -9.687362902255692632, -62.58071313852362039 ) ) ;
#94941=AXIS2_PLACEMENT_3D ( 'NONE', #129681, #125731, #188408 ) ;
#94942=CARTESIAN_POINT ( 'NONE',  ( -21.30000000000002913, 2.244099063931684814E-13, -56.46919128290398504 ) ) ;
#94956=CARTESIAN_POINT ( 'NONE',  ( -3.921756399366283397, -4.986025004891486923, -62.46690648838622906 ) ) ;
#94972=ORIENTED_EDGE ( 'NONE', *, *, #85361, .T. ) ;
#94976=CARTESIAN_POINT ( 'NONE',  ( 33.78191506369888941, -21.41920200728860380, -24.99999999999997868 ) ) ;
#95041=VECTOR ( 'NONE', #64610, 1000.000000000000000 ) ;
#95066=AXIS2_PLACEMENT_3D ( 'NONE', #174427, #35897, #33921 ) ;
#95074=CARTESIAN_POINT ( 'NONE',  ( -13.70000000000001528, 1.443387660838688656E-13, -62.58071313852362039 ) ) ;
#95137=CARTESIAN_POINT ( 'NONE',  ( -19.82991159619237820, -34.74521775907871302, -25.51696690232505915 ) ) ;
#95152=CIRCLE ( 'NONE', #130657, 206.0437394197456342 ) ;
#95180=ADVANCED_FACE ( 'NONE', ( #115333 ), #113318, .F. ) ;
#95181=AXIS2_PLACEMENT_3D ( 'NONE', #16545, #78192, #122715 ) ;
#95199=VECTOR ( 'NONE', #57448, 1000.000000000000000 ) ;
#95224=CARTESIAN_POINT ( 'NONE',  ( 8.207766490800741721, -46.52841682978063886, -24.35011552986999916 ) ) ;
#95255=EDGE_CURVE ( 'NONE', #34342, #127568, #130705, .T. ) ;
#95256=ORIENTED_EDGE ( 'NONE', *, *, #84631, .T. ) ;
#95270=CARTESIAN_POINT ( 'NONE',  ( 13.57915378923102523, -35.22819508409087064, -29.39033328706047854 ) ) ;
#95274=ORIENTED_EDGE ( 'NONE', *, *, #14847, .T. ) ;
#95345=AXIS2_PLACEMENT_3D ( 'NONE', #186546, #171356, #79333 ) ;
#95379=CARTESIAN_POINT ( 'NONE',  ( -38.00000000000000711, 2.428612866367529932E-14, -8.000000000000000000 ) ) ;
#95381=DIRECTION ( 'NONE',  ( 1.000000000000000000, 9.445700745138859830E-17, -0.000000000000000000 ) ) ;
#95420=ORIENTED_EDGE ( 'NONE', *, *, #154300, .F. ) ;
#95432=ADVANCED_FACE ( 'NONE', ( #162827 ), #146652, .T. ) ;
#95434=CARTESIAN_POINT ( 'NONE',  ( -27.86627820654446808, -25.72419401236984982, -16.61045157392797122 ) ) ;
#95451=FACE_OUTER_BOUND ( 'NONE', #117455, .T. ) ;
#95456=CARTESIAN_POINT ( 'NONE',  ( 22.99604614807110181, -21.34824663401120759, -46.43544609871632645 ) ) ;
#95462=CYLINDRICAL_SURFACE ( 'NONE', #20910, 24.30000000000003268 ) ;
#95464=CARTESIAN_POINT ( 'NONE',  ( 21.24746703654597724, -20.01434088805876144, -52.34924278636284356 ) ) ;
#95482=CARTESIAN_POINT ( 'NONE',  ( 22.81625015709510151, -31.40387420917324590, -1.924999997268813434 ) ) ;
#95492=CARTESIAN_POINT ( 'NONE',  ( 25.01910340989057246, -31.27285607038160364, -17.23782325461877107 ) ) ;
#95543=CARTESIAN_POINT ( 'NONE',  ( -5.950531402560715689E-15, 38.81732327939063509, -3.124999997268813168 ) ) ;
#95563=CARTESIAN_POINT ( 'NONE',  ( -1.135848680322148585, -6.615299585309119657, -64.43295106733368982 ) ) ;
#95565=CIRCLE ( 'NONE', #56924, 8.000000000000007105 ) ;
#95578=CARTESIAN_POINT ( 'NONE',  ( 31.21487366219226445, -1.272595016298689430, -49.98150452412664180 ) ) ;
#95584=EDGE_CURVE ( 'NONE', #36546, #115704, #119367, .T. ) ;
#95674=EDGE_CURVE ( 'NONE', #39588, #126569, #42631, .T. ) ;
#95706=CARTESIAN_POINT ( 'NONE',  ( 0.2242313521320748737, 21.31285307430665554, -56.45988244333290851 ) ) ;
#95716=LINE ( 'NONE', #68361, #188892 ) ;
#95727=CARTESIAN_POINT ( 'NONE',  ( -19.99999999999998224, -190.0000000000000000, -25.00000000000000000 ) ) ;
#95730=CARTESIAN_POINT ( 'NONE',  ( -36.91746825000001309, 11.99521256947798342, -7.224999997268814589 ) ) ;
#95766=CARTESIAN_POINT ( 'NONE',  ( 37.99999999999999289, 2.893978650043524126E-14, -9.000000000000001776 ) ) ;
#95780=CARTESIAN_POINT ( 'NONE',  ( -22.81625015709510507, 31.40387420917330275, -7.424999997268812990 ) ) ;
#95788=CARTESIAN_POINT ( 'NONE',  ( 9.349452323154965327, -36.27485578735120697, -31.39434858484990798 ) ) ;
#95909=CARTESIAN_POINT ( 'NONE',  ( 1.500000000004064082, 7.599999999999568878, -62.20201607440122871 ) ) ;
#95949=B_SPLINE_CURVE_WITH_KNOTS ( 'NONE', 3,
 ( #5750, #52257, #135120, #41104, #86595, #8766, #10773, #54266, #102768, #72437, #134114, #40084, #100752, #7742, #38101, #9771, #148278, #149278, #57275, #70435, #69428, #22932, #101763, #146258, #132101, #55260 ),
 .UNSPECIFIED., .F., .F.,
 ( 4, 2, 2, 2, 2, 2, 2, 2, 2, 2, 2, 2, 4 ),
 ( 1.969502666007334865E-07, 0.0004009345686709441360, 0.0008016721870752876794, 0.001603147423883954708, 0.002404622660692621629, 0.003206097897501288766, 0.004007573134309955903, 0.004408310752714287087, 0.004809048371118616536, 0.005209785989522947719, 0.005610523607927278902, 0.006011261226331608351, 0.006411998844735939534 ),
 .UNSPECIFIED. ) ;
#95951=CARTESIAN_POINT ( 'NONE',  ( 15.62200626734387754, -14.69813070946463718, -56.36792940895625748 ) ) ;
#95981=CARTESIAN_POINT ( 'NONE',  ( 0.000000000000000000, -64.82615989628266107, -25.00000000000000000 ) ) ;
#95983=CARTESIAN_POINT ( 'NONE',  ( -1.497147075633523894, -30.58708291193884676, -50.73425184351846440 ) ) ;
#96035=DIRECTION ( 'NONE',  ( 0.000000000000000000, 0.000000000000000000, 1.000000000000000000 ) ) ;
#96067=CARTESIAN_POINT ( 'NONE',  ( -1.203758653825231395, -8.516083024820099823, -62.01440738234572336 ) ) ;
#96102=CARTESIAN_POINT ( 'NONE',  ( -6.206452982517636663, -6.630588440586430821, -61.89901439314702003 ) ) ;
#96110=VECTOR ( 'NONE', #151594, 1000.000000000000000 ) ;
#96130=CYLINDRICAL_SURFACE ( 'NONE', #43783, 61.99999999999998579 ) ;
#96184=CYLINDRICAL_SURFACE ( 'NONE', #150317, 21.30000000000002913 ) ;
#96193=CARTESIAN_POINT ( 'NONE',  ( 0.1123858161134816402, 24.30000000000003979, -54.21489346206829651 ) ) ;
#96214=CARTESIAN_POINT ( 'NONE',  ( 27.99526582847387957, -28.30548820594174586, -16.92425894792105723 ) ) ;
#96220=FACE_BOUND ( 'NONE', #118898, .T. ) ;
#96232=ORIENTED_EDGE ( 'NONE', *, *, #83620, .T. ) ;
#96249=AXIS2_PLACEMENT_3D ( 'NONE', #114003, #116024, #69519 ) ;
#96259=CARTESIAN_POINT ( 'NONE',  ( 30.67396074481323254, -22.36774236107039471, -23.13178788717692314 ) ) ;
#96295=EDGE_CURVE ( 'NONE', #50694, #190550, #89908, .T. ) ;
#96319=DIRECTION ( 'NONE',  ( 1.000000000000000000, 0.000000000000000000, 0.000000000000000000 ) ) ;
#96324=CARTESIAN_POINT ( 'NONE',  ( 6.139906835403837526, -0.3968392070109495462, -62.49911542708241541 ) ) ;
#96367=CARTESIAN_POINT ( 'NONE',  ( 9.250641775538104739, 10.87998047749157493, -60.21451611132644643 ) ) ;
#96369=CARTESIAN_POINT ( 'NONE',  ( -19.99604614807122971, -21.41083295479474202, -52.23501749411500583 ) ) ;
#96405=ORIENTED_EDGE ( 'NONE', *, *, #81756, .F. ) ;
#96419=ORIENTED_EDGE ( 'NONE', *, *, #110986, .F. ) ;
#96421=CARTESIAN_POINT ( 'NONE',  ( -30.67396074481678525, -22.36774236106498748, -23.13178788717137024 ) ) ;
#96437=FACE_OUTER_BOUND ( 'NONE', #158625, .T. ) ;
#96442=CARTESIAN_POINT ( 'NONE',  ( -29.79829367730025425, 1.376802789501195168, -48.54110828511536369 ) ) ;
#96450=CARTESIAN_POINT ( 'NONE',  ( 21.32838159582145821, -20.00333696053909804, -52.29425578929144791 ) ) ;
#96466=CARTESIAN_POINT ( 'NONE',  ( 3.556970738554033499E-15, -38.81732327939057825, -2.124999997268813612 ) ) ;
#96476=CARTESIAN_POINT ( 'NONE',  ( 21.44681783661738095, -33.76292609718872484, -24.06782133912101074 ) ) ;
#96514=LINE ( 'NONE', #20677, #128181 ) ;
#96522=LINE ( 'NONE', #158212, #86744 ) ;
#96526=CARTESIAN_POINT ( 'NONE',  ( 22.81625015709509441, 31.40387420917330275, -9.824999997268811569 ) ) ;
#96584=DIRECTION ( 'NONE',  ( -1.000000000000000000, 0.000000000000000000, -3.642919299551293321E-15 ) ) ;
#96672=CARTESIAN_POINT ( 'NONE',  ( 11.74264578624800315, -36.14014761921581709, -5.400000000000000355 ) ) ;
#96712=CARTESIAN_POINT ( 'NONE',  ( -11.40812507854755609, 35.11059874428196537, -7.524999997268813523 ) ) ;
#96745=DIRECTION ( 'NONE',  ( 1.000000000000000000, 0.000000000000000000, 0.000000000000000000 ) ) ;
#96758=CARTESIAN_POINT ( 'NONE',  ( -11.40812507854754720, -35.11059874428192273, -2.724999997268813257 ) ) ;
#96760=AXIS2_PLACEMENT_3D ( 'NONE', #134923, #196600, #58071 ) ;
#96766=CARTESIAN_POINT ( 'NONE',  ( 10.74802307403555268, -10.74802307403551715, -64.92279855667830191 ) ) ;
#96770=CARTESIAN_POINT ( 'NONE',  ( 1.500000000002908562, 30.39999999999990266, -50.95361246531977173 ) ) ;
#96774=ORIENTED_EDGE ( 'NONE', *, *, #15073, .T. ) ;
#96783=ORIENTED_EDGE ( 'NONE', *, *, #44126, .F. ) ;
#96794=EDGE_LOOP ( 'NONE', ( #67086, #149170, #173715, #64192 ) ) ;
#96802=EDGE_CURVE ( 'NONE', #150285, #103031, #174182, .T. ) ;
#96832=ORIENTED_EDGE ( 'NONE', *, *, #136692, .T. ) ;
#96835=DIRECTION ( 'NONE',  ( -0.000000000000000000, -0.000000000000000000, 1.000000000000000000 ) ) ;
#96907=CIRCLE ( 'NONE', #35576, 21.30000000000002913 ) ;
#96915=CARTESIAN_POINT ( 'NONE',  ( -23.94081952771225730, 0.9791052130477023718, -54.49391133501602980 ) ) ;
#96928=CARTESIAN_POINT ( 'NONE',  ( -30.74264578624800492, 22.33583958711400186, -0.1999999999999999001 ) ) ;
#96948=CARTESIAN_POINT ( 'NONE',  ( 33.40031027765339644, -22.02106105253703561, -24.45416078184958408 ) ) ;
#96950=CARTESIAN_POINT ( 'NONE',  ( -4.313351365237978463, -4.313351365237916291, -62.50719930893269805 ) ) ;
#96960=DIRECTION ( 'NONE',  ( -0.000000000000000000, -0.000000000000000000, 1.000000000000000000 ) ) ;
#96962=CARTESIAN_POINT ( 'NONE',  ( 21.64789649210667832, -31.17538106138185938, -22.95353217465963880 ) ) ;
#96974=CARTESIAN_POINT ( 'NONE',  ( 10.59477242850415024, -90.60836494048558620, 0.000000000000000000 ) ) ;
#97000=ORIENTED_EDGE ( 'NONE', *, *, #185422, .F. ) ;
#97005=CARTESIAN_POINT ( 'NONE',  ( -0.5097844185665340033, -31.81624771892549575, -45.77220262091588410 ) ) ;
#97017=CARTESIAN_POINT ( 'NONE',  ( -13.56018889279570949, -37.30201529093374546, -30.04439950253825131 ) ) ;
#97029=CARTESIAN_POINT ( 'NONE',  ( 10.91551912637963540, 12.25159394783730882, -61.48002405683646288 ) ) ;
#97033=CARTESIAN_POINT ( 'NONE',  ( 0.000000000000000000, 0.000000000000000000, -64.92279855667830191 ) ) ;
#97036=EDGE_CURVE ( 'NONE', #128045, #117002, #200029, .T. ) ;
#97048=CARTESIAN_POINT ( 'NONE',  ( -0.1001428631146457915, -9.099999999999999645, -61.89430850415823215 ) ) ;
#97070=VECTOR ( 'NONE', #23267, 1000.000000000000000 ) ;
#97082=DIRECTION ( 'NONE',  ( 1.000000000000000000, 0.000000000000000000, 0.000000000000000000 ) ) ;
#97143=CARTESIAN_POINT ( 'NONE',  ( -4.999999999999996447, 5.000000000000003553, -18.00000000000000000 ) ) ;
#97172=CARTESIAN_POINT ( 'NONE',  ( 13.70000000000001528, -4.867217739956692332E-14, -62.58071313852362039 ) ) ;
#97189=CYLINDRICAL_SURFACE ( 'NONE', #121819, 9.100000000000001421 ) ;
#97205=DIRECTION ( 'NONE',  ( 1.000000000000000000, 1.776356839400250465E-15, 0.000000000000000000 ) ) ;
#97215=CARTESIAN_POINT ( 'NONE',  ( -30.74264578624800492, -22.33583958711396278, -9.799999999999998934 ) ) ;
#97233=CARTESIAN_POINT ( 'NONE',  ( -11.45643923738959735, 5.000000000000007105, -18.00000000000000000 ) ) ;
#97237=DIRECTION ( 'NONE',  ( 1.000000000000000000, 0.000000000000000000, 0.000000000000000000 ) ) ;
#97348=CARTESIAN_POINT ( 'NONE',  ( 9.979736640218535015, 12.05038478428676463, -59.62998087139816050 ) ) ;
#97399=CARTESIAN_POINT ( 'NONE',  ( -27.75745401094723874, -25.59313184531950114, -20.67669038791073177 ) ) ;
#97418=EDGE_CURVE ( 'NONE', #117777, #70701, #93938, .T. ) ;
#97441=CARTESIAN_POINT ( 'NONE',  ( 0.000000000000000000, -165.0000000000000000, 5.497848452431111532 ) ) ;
#97447=CARTESIAN_POINT ( 'NONE',  ( 22.81625015709509441, 31.40387420917330275, -1.324999997268813123 ) ) ;
#97457=CARTESIAN_POINT ( 'NONE',  ( 25.95926362436975765, -29.82107321766389063, -18.67624575279086940 ) ) ;
#97465=ADVANCED_FACE ( 'NONE', ( #188962 ), #111097, .F. ) ;
#97496=DIRECTION ( 'NONE',  ( -0.000000000000000000, -0.000000000000000000, 1.000000000000000000 ) ) ;
#97509=CARTESIAN_POINT ( 'NONE',  ( -29.86685920354755197, -21.69954338932560134, -10.92499999726881299 ) ) ;
#97510=CARTESIAN_POINT ( 'NONE',  ( 11.74264578624799427, 36.14014761921585972, -2.349999994537626868 ) ) ;
#97525=ADVANCED_FACE ( 'NONE', ( #16118 ), #139442, .T. ) ;
#97573=ORIENTED_EDGE ( 'NONE', *, *, #145835, .F. ) ;
#97653=CARTESIAN_POINT ( 'NONE',  ( 20.09153389842217763, 22.04836444019709418, -48.54295043639822183 ) ) ;
#97654=ADVANCED_FACE ( 'NONE', ( #47456 ), #109112, .T. ) ;
#97659=CARTESIAN_POINT ( 'NONE',  ( -37.66961640367473052, 5.000000000000023981, -15.00000000000000000 ) ) ;
#97663=CARTESIAN_POINT ( 'NONE',  ( 37.99999999999999289, 2.428612866367529932E-14, -25.00000000000000000 ) ) ;
#97672=CARTESIAN_POINT ( 'NONE',  ( 15.06137443927350361, 15.06137443927346098, -58.85720012050613548 ) ) ;
#97678=CARTESIAN_POINT ( 'NONE',  ( 22.55670631985092811, 22.55670631985084640, -45.64921306006598201 ) ) ;
#97680=CARTESIAN_POINT ( 'NONE',  ( -5.950531402560715689E-15, 38.81732327939063509, -3.124999997268813168 ) ) ;
#97690=DIRECTION ( 'NONE',  ( -0.000000000000000000, -0.000000000000000000, 1.000000000000000000 ) ) ;
#97694=CARTESIAN_POINT ( 'NONE',  ( 36.91746825000000598, -11.99521256947793546, -10.22499999726881548 ) ) ;
#97738=CIRCLE ( 'NONE', #75267, 8.000000000000000000 ) ;
#97743=CARTESIAN_POINT ( 'NONE',  ( -11.40812507854755609, 35.11059874428196537, -1.524999997268813301 ) ) ;
#97744=EDGE_CURVE ( 'NONE', #198744, #154699, #148359, .T. ) ;
#97833=CARTESIAN_POINT ( 'NONE',  ( 26.46959431505287341, -27.26463967846483527, -11.00411086000093519 ) ) ;
#97852=CYLINDRICAL_SURFACE ( 'NONE', #89340, 1.499999999999996225 ) ;
#97893=CARTESIAN_POINT ( 'NONE',  ( -1.218621689577036982, -14.30340603398754418, -62.33590500446654659 ) ) ;
#97894=ADVANCED_FACE ( 'NONE', ( #177771 ), #176775, .F. ) ;
#97907=CARTESIAN_POINT ( 'NONE',  ( -6.020228577223754586E-15, 39.95556452105416412, -0.4999999999999998890 ) ) ;
#97910=CARTESIAN_POINT ( 'NONE',  ( -28.90000000000004121, 0.1280799071100958975, -52.65483682830181777 ) ) ;
#97915=DIRECTION ( 'NONE',  ( -0.000000000000000000, -0.000000000000000000, 1.000000000000000000 ) ) ;
#97940=CIRCLE ( 'NONE', #84974, 216.0437394197456911 ) ;
#97941=CYLINDRICAL_SURFACE ( 'NONE', #25158, 10.00000000000000000 ) ;
#97979=DIRECTION ( 'NONE',  ( -0.000000000000000000, -0.000000000000000000, 1.000000000000000000 ) ) ;
#97991=DIRECTION ( 'NONE',  ( 0.07151044867601324961, 0.9974398506828144884, 0.000000000000000000 ) ) ;
#98021=CARTESIAN_POINT ( 'NONE',  ( 3.766062262543149401E-15, -39.95556452105413570, -9.249999994537628112 ) ) ;
#98051=DIRECTION ( 'NONE',  ( -0.9930308165857338887, 0.1178549842436489581, 0.000000000000000000 ) ) ;
#98131=CARTESIAN_POINT ( 'NONE',  ( -14.71325192251711833, -16.70647688133528064, -58.23439181598958925 ) ) ;
#98151=FACE_OUTER_BOUND ( 'NONE', #99641, .T. ) ;
#98163=ADVANCED_FACE ( 'NONE', ( #162581 ), #41441, .T. ) ;
#98195=CARTESIAN_POINT ( 'NONE',  ( -14.82524568295233891, 1.464953661134127172, -59.95866808466630715 ) ) ;
#98211=CIRCLE ( 'NONE', #133772, 2.500000000000000000 ) ;
#98229=CARTESIAN_POINT ( 'NONE',  ( 27.18398240159043411, -26.16474475603006056, -20.45985799059559085 ) ) ;
#98272=EDGE_CURVE ( 'NONE', #4269, #177278, #53736, .T. ) ;
#98300=EDGE_CURVE ( 'NONE', #35769, #40993, #162247, .T. ) ;
#98302=AXIS2_PLACEMENT_3D ( 'NONE', #49576, #169936, #112238 ) ;
#98346=CARTESIAN_POINT ( 'NONE',  ( 11.30153831258470731, -188.0000000000000000, -15.00000000000000178 ) ) ;
#98385=ORIENTED_EDGE ( 'NONE', *, *, #144467, .F. ) ;
#98431=EDGE_CURVE ( 'NONE', #179471, #137572, #174325, .T. ) ;
#98436=B_SPLINE_CURVE_WITH_KNOTS ( 'NONE', 3,
 ( #184406, #153055, #170223, #136902, #62030, #31716, #93364, #199575, #198589, #28758, #14557, #197599 ),
 .UNSPECIFIED., .F., .F.,
 ( 4, 2, 2, 2, 2, 4 ),
 ( 1.961533960389205320E-07, 0.0007644364765400004508, 0.001146556638111986392, 0.001528676799683972333, 0.002292917122827955491, 0.003057157445971939082 ),
 .UNSPECIFIED. ) ;
#98453=CARTESIAN_POINT ( 'NONE',  ( 36.91746824999999887, 11.99521256947799053, -1.524999997268813745 ) ) ;
#98463=CARTESIAN_POINT ( 'NONE',  ( 29.81671572245950230, -26.02765724076281373, -18.90727510134258793 ) ) ;
#98483=ORIENTED_EDGE ( 'NONE', *, *, #40630, .T. ) ;
#98515=CARTESIAN_POINT ( 'NONE',  ( -36.91746825000001309, -11.99521256947794789, -11.02499999726881263 ) ) ;
#98516=CARTESIAN_POINT ( 'NONE',  ( -12.49999999999997691, -89.99999999999997158, -25.00000000000000000 ) ) ;
#98551=CARTESIAN_POINT ( 'NONE',  ( 30.74735067906814479, -1.468823602708525300, -50.54421433284817056 ) ) ;
#98554=CARTESIAN_POINT ( 'NONE',  ( -69.65682714487590488, -71.74905178543390605, -25.00000000000000000 ) ) ;
#98581=ORIENTED_EDGE ( 'NONE', *, *, #17432, .F. ) ;
#98678=CARTESIAN_POINT ( 'NONE',  ( -32.12256032297297992, -23.75458735917140629, -22.83990191704113926 ) ) ;
#98682=DIRECTION ( 'NONE',  ( 3.469446951953612217E-15, 0.000000000000000000, -1.000000000000000000 ) ) ;
#98690=CARTESIAN_POINT ( 'NONE',  ( 22.81625015709509441, 31.40387420917330275, -5.324999997268813345 ) ) ;
#98752=CARTESIAN_POINT ( 'NONE',  ( -22.02279270211228734, 20.08125529445633006, -51.67964572521218969 ) ) ;
#98784=CIRCLE ( 'NONE', #79470, 59.99999999999998579 ) ;
#98810=EDGE_CURVE ( 'NONE', #6817, #108968, #29018, .T. ) ;
#98820=EDGE_LOOP ( 'NONE', ( #130332, #168172, #41375, #89844, #180374, #61969, #57530, #71862, #14291, #142787 ) ) ;
#98879=EDGE_CURVE ( 'NONE', #117432, #179471, #167845, .T. ) ;
#98896=CARTESIAN_POINT ( 'NONE',  ( -7.840974544915187749, -46.02298249793906137, -22.40017284086422222 ) ) ;
#98925=FACE_OUTER_BOUND ( 'NONE', #101307, .T. ) ;
#98936=CARTESIAN_POINT ( 'NONE',  ( 0.000000000000000000, 0.000000000000000000, -62.91767397929362460 ) ) ;
#98938=CARTESIAN_POINT ( 'NONE',  ( -23.48529157249600985, 32.32473071737754111, -2.049999994537626158 ) ) ;
#98947=CARTESIAN_POINT ( 'NONE',  ( 2.500000000000000000, -165.0000000000000000, 7.000000000000003553 ) ) ;
#98951=CARTESIAN_POINT ( 'NONE',  ( 4.999999999999996447, 37.66961640367475184, -25.00000000000000000 ) ) ;
#98954=CARTESIAN_POINT ( 'NONE',  ( 29.12359114459363951, -24.18000288461011493, -21.55587802759514204 ) ) ;
#98990=CARTESIAN_POINT ( 'NONE',  ( -2.973862142520655727, -93.04182470242766101, -23.00000000000000000 ) ) ;
#98997=DIRECTION ( 'NONE',  ( 0.000000000000000000, 0.000000000000000000, -1.000000000000000000 ) ) ;
#99009=CARTESIAN_POINT ( 'NONE',  ( -11.23063180225521407, -38.81524874330040831, -25.08899775095413531 ) ) ;
#99026=CARTESIAN_POINT ( 'NONE',  ( -12.49999999999997691, -89.99999999999997158, 0.000000000000000000 ) ) ;
#99054=EDGE_CURVE ( 'NONE', #111207, #126376, #16150, .T. ) ;
#99070=CARTESIAN_POINT ( 'NONE',  ( -38.00000000000000711, 2.428612866367529932E-14, -4.000000000000000000 ) ) ;
#99080=DIRECTION ( 'NONE',  ( -0.000000000000000000, -0.000000000000000000, 1.000000000000000000 ) ) ;
#99107=DIRECTION ( 'NONE',  ( 0.000000000000000000, 0.000000000000000000, 1.000000000000000000 ) ) ;
#99147=CARTESIAN_POINT ( 'NONE',  ( -37.99999999999997158, 12.34694845685052123, -6.100000000000001421 ) ) ;
#99187=ORIENTED_EDGE ( 'NONE', *, *, #5609, .F. ) ;
#99196=DIRECTION ( 'NONE',  ( -1.000000000000000000, 0.000000000000000000, 0.000000000000000000 ) ) ;
#99198=DIRECTION ( 'NONE',  ( 0.000000000000000000, 0.000000000000000000, -1.000000000000000000 ) ) ;
#99213=CARTESIAN_POINT ( 'NONE',  ( -15.84196527238551333, 1.359015117358495894, -59.51370404797112457 ) ) ;
#99221=ADVANCED_FACE ( 'NONE', ( #92114 ), #116156, .T. ) ;
#99242=DIRECTION ( 'NONE',  ( 0.000000000000000000, 0.000000000000000000, 1.000000000000000000 ) ) ;
#99246=CARTESIAN_POINT ( 'NONE',  ( -2.973862142520662832, -93.04182470242767522, -25.00000000000000000 ) ) ;
#99250=EDGE_LOOP ( 'NONE', ( #41006, #38510, #20823, #124623 ) ) ;
#99310=VERTEX_POINT ( 'NONE', #75967 ) ;
#99351=FACE_OUTER_BOUND ( 'NONE', #89002, .T. ) ;
#99398=ORIENTED_EDGE ( 'NONE', *, *, #132358, .T. ) ;
#99403=ORIENTED_EDGE ( 'NONE', *, *, #193896, .F. ) ;
#99463=CARTESIAN_POINT ( 'NONE',  ( 3.766062262543149401E-15, -39.95556452105413570, -1.499999999999999778 ) ) ;
#99469=CARTESIAN_POINT ( 'NONE',  ( -37.66961640367473052, 5.000000000000023981, -18.00000000000000355 ) ) ;
#99481=CARTESIAN_POINT ( 'NONE',  ( -11.30153831258470731, -180.0000000000000000, 0.000000000000000000 ) ) ;
#99520=ORIENTED_EDGE ( 'NONE', *, *, #189654, .F. ) ;
#99525=CARTESIAN_POINT ( 'NONE',  ( -11.40812507854755609, 35.11059874428196537, -7.024999997268813523 ) ) ;
#99539=ORIENTED_EDGE ( 'NONE', *, *, #47298, .F. ) ;
#99560=CARTESIAN_POINT ( 'NONE',  ( -30.74264578624800492, -22.33583958711396278, -1.800000000000000044 ) ) ;
#99564=CYLINDRICAL_SURFACE ( 'NONE', #148332, 6.100000000000006750 ) ;
#99641=EDGE_LOOP ( 'NONE', ( #62638, #180612, #163869, #140696 ) ) ;
#99666=ADVANCED_FACE ( 'NONE', ( #187157 ), #35429, .F. ) ;
#99687=CARTESIAN_POINT ( 'NONE',  ( -30.20036327792369235, -26.22857331006468229, -17.18026671435357500 ) ) ;
#99696=CARTESIAN_POINT ( 'NONE',  ( 0.000000000000000000, -78.67194367458512261, -25.00000000000000000 ) ) ;
#99698=CARTESIAN_POINT ( 'NONE',  ( -22.81625015709510507, 31.40387420917330275, -4.924999997268813878 ) ) ;
#99705=ORIENTED_EDGE ( 'NONE', *, *, #30838, .F. ) ;
#99756=CARTESIAN_POINT ( 'NONE',  ( 1.022580077288041090E-15, 16.70000000000002061, -59.13370768023891344 ) ) ;
#99783=VERTEX_POINT ( 'NONE', #34443 ) ;
#99828=ADVANCED_FACE ( 'NONE', ( #4084 ), #20254, .F. ) ;
#99831=VERTEX_POINT ( 'NONE', #66759 ) ;
#99869=CARTESIAN_POINT ( 'NONE',  ( -38.00000000000000711, 12.34694845685046438, -1.849999994537626424 ) ) ;
#99902=CARTESIAN_POINT ( 'NONE',  ( -8.377002814026733191, -36.45346134345093247, -31.71922177526237974 ) ) ;
#99906=CARTESIAN_POINT ( 'NONE',  ( 11.61039618804099049, -9.512461411204764516, -62.07742545104463971 ) ) ;
#99924=CARTESIAN_POINT ( 'NONE',  ( -29.61737564226528363, 1.282731051913388320, -51.85482277101433368 ) ) ;
#99940=CARTESIAN_POINT ( 'NONE',  ( 9.687362902255733488, -9.687362902255692632, -62.58071313852362039 ) ) ;
#99942=CARTESIAN_POINT ( 'NONE',  ( 38.00000000000000711, -12.34694845685040754, -8.849999994537625980 ) ) ;
#99950=CARTESIAN_POINT ( 'NONE',  ( -193.3062444957834884, -155.7167183371838064, -15.00000000000000178 ) ) ;
#99951=CARTESIAN_POINT ( 'NONE',  ( -16.12203461105344005, -16.12203461105316649, -64.92279855667830191 ) ) ;
#99955=DIRECTION ( 'NONE',  ( 1.000000000000000000, 0.000000000000000000, 0.000000000000000000 ) ) ;
#99957=EDGE_CURVE ( 'NONE', #40990, #46712, #154704, .T. ) ;
#100014=CARTESIAN_POINT ( 'NONE',  ( -9.824205582590950669, -39.25481172344220937, -25.36904614590413587 ) ) ;
#100015=VERTEX_POINT ( 'NONE', #157791 ) ;
#100027=ORIENTED_EDGE ( 'NONE', *, *, #83620, .F. ) ;
#100043=DIRECTION ( 'NONE',  ( 0.000000000000000000, 0.000000000000000000, 1.000000000000000000 ) ) ;
#100087=CARTESIAN_POINT ( 'NONE',  ( -15.06137443927351249, 15.06137443927345210, -65.00100000000003320 ) ) ;
#100123=AXIS2_PLACEMENT_3D ( 'NONE', #109286, #169968, #168960 ) ;
#100204=EDGE_CURVE ( 'NONE', #64219, #89664, #113256, .T. ) ;
#100205=CARTESIAN_POINT ( 'NONE',  ( 30.20036327792367814, -26.22857331006468584, -17.18026671435356434 ) ) ;
#100225=ORIENTED_EDGE ( 'NONE', *, *, #90031, .T. ) ;
#100251=CARTESIAN_POINT ( 'NONE',  ( 32.72233185158318491, -19.32382731392758402, -21.08582493607095998 ) ) ;
#100317=CARTESIAN_POINT ( 'NONE',  ( 1.197038699967498898, 6.690841975426986998, -64.41838970491137673 ) ) ;
#100331=ADVANCED_BREP_SHAPE_REPRESENTATION ( '', ( #9086, #82054 ), #24091 ) ;
#100355=CARTESIAN_POINT ( 'NONE',  ( -38.00000000000000711, 2.428612866367529932E-14, -3.749999994537626780 ) ) ;
#100403=VERTEX_POINT ( 'NONE', #62020 ) ;
#100409=CARTESIAN_POINT ( 'NONE',  ( 37.99999999999999289, 2.893978650043524126E-14, -3.000000000000000000 ) ) ;
#100433=ORIENTED_EDGE ( 'NONE', *, *, #186918, .T. ) ;
#100447=FACE_OUTER_BOUND ( 'NONE', #73995, .T. ) ;
#100449=CARTESIAN_POINT ( 'NONE',  ( 30.20036327792367814, -26.22857331006468584, -17.18026671435356434 ) ) ;
#100466=CARTESIAN_POINT ( 'NONE',  ( -38.00000000000000711, 2.428612866367529932E-14, 1.084202172485504434E-16 ) ) ;
#100488=ORIENTED_EDGE ( 'NONE', *, *, #125347, .F. ) ;
#100525=CARTESIAN_POINT ( 'NONE',  ( 36.91746825000000598, -11.99521256947793546, -3.724999997268812812 ) ) ;
#100530=CARTESIAN_POINT ( 'NONE',  ( 6.852337434880861444, -5.080399118595191332, -64.08013955860572253 ) ) ;
#100560=DIRECTION ( 'NONE',  ( 0.000000000000000000, 0.000000000000000000, 1.000000000000000000 ) ) ;
#100563=DIRECTION ( 'NONE',  ( -1.000000000000000000, 0.000000000000000000, 0.000000000000000000 ) ) ;
#100613=EDGE_CURVE ( 'NONE', #146440, #167327, #157599, .T. ) ;
#100656=ORIENTED_EDGE ( 'NONE', *, *, #144097, .F. ) ;
#100683=DIRECTION ( 'NONE',  ( -0.000000000000000000, -0.000000000000000000, 1.000000000000000000 ) ) ;
#100694=CARTESIAN_POINT ( 'NONE',  ( -5.950531402560715689E-15, 38.81732327939063509, -1.124999997268813168 ) ) ;
#100704=CARTESIAN_POINT ( 'NONE',  ( -31.56198012149236121, -21.16321310694279489, -23.06581160126869179 ) ) ;
#100729=ORIENTED_EDGE ( 'NONE', *, *, #1190, .F. ) ;
#100752=CARTESIAN_POINT ( 'NONE',  ( 30.11448378070090470, -1.481880339025618110, -48.12989299794426756 ) ) ;
#100766=CARTESIAN_POINT ( 'NONE',  ( 14.93915603648730261, 17.06172130128247844, -57.95097928225586514 ) ) ;
#100880=CYLINDRICAL_SURFACE ( 'NONE', #11677, 1.500000000000001332 ) ;
#100940=CARTESIAN_POINT ( 'NONE',  ( 3.766062262543149401E-15, -39.95556452105413570, -5.249999994537625447 ) ) ;
#100949=CARTESIAN_POINT ( 'NONE',  ( 22.87077540613818982, -22.10389085601126169, -45.79323219683391244 ) ) ;
#100953=CYLINDRICAL_SURFACE ( 'NONE', #12309, 38.00000000000000000 ) ;
#100992=CARTESIAN_POINT ( 'NONE',  ( 11.40812507854755253, -35.11059874428192273, -4.524999997268813523 ) ) ;
#100993=DIRECTION ( 'NONE',  ( 1.000000000000000000, 0.000000000000000000, 0.000000000000000000 ) ) ;
#101015=CARTESIAN_POINT ( 'NONE',  ( -11.94140034372569303, -38.57382067147337779, -24.90972908440997102 ) ) ;
#101025=CARTESIAN_POINT ( 'NONE',  ( 69.65682714487590488, -71.74905178543389184, -10.00000000000000000 ) ) ;
#101037=CARTESIAN_POINT ( 'NONE',  ( 26.46959431505284499, -27.26463967846488146, -15.00000000000000178 ) ) ;
#101067=CYLINDRICAL_SURFACE ( 'NONE', #4217, 1.499999999999997780 ) ;
#101082=B_SPLINE_CURVE_WITH_KNOTS ( 'NONE', 3,
 ( #107868, #129987, #20839, #174538, #191687, #51186, #177545, #112847, #97653, #66349, #178537, #148195, #67341, #38016, #85502, #82496, #36005, #147191, #128011, #159343, #144179, #192699, #7657, #69341 ),
 .UNSPECIFIED., .F., .F.,
 ( 4, 2, 2, 2, 2, 2, 2, 2, 2, 2, 2, 4 ),
 ( 2.775519118949223281E-07, 0.0003993838752237327430, 0.0007984901985355705861, 0.001596702845159246814, 0.002394915491782922609, 0.003193128138406599054, 0.003991340785030274632, 0.004789553431653949776, 0.005188659754965791251, 0.005587766078277632727, 0.005986872401589474202, 0.006385978724901315677 ),
 .UNSPECIFIED. ) ;
#101157=EDGE_LOOP ( 'NONE', ( #190250, #115671, #3708 ) ) ;
#101210=CARTESIAN_POINT ( 'NONE',  ( -2.500000000000000000, 3.061616997868383141E-16, -62.91767397929362460 ) ) ;
#101219=VECTOR ( 'NONE', #65985, 1000.000000000000000 ) ;
#101239=( LENGTH_UNIT ( ) NAMED_UNIT ( * ) SI_UNIT ( .MILLI., .METRE. ) );
#101270=PLANE ( 'NONE',  #78081 ) ;
#101307=EDGE_LOOP ( 'NONE', ( #104320, #181731, #100656, #130443 ) ) ;
#101313=CARTESIAN_POINT ( 'NONE',  ( -69.65682714487590488, -71.74905178543390605, 0.000000000000000000 ) ) ;
#101399=DIRECTION ( 'NONE',  ( 1.000000000000000000, 0.000000000000000000, 0.000000000000000000 ) ) ;
#101409=CARTESIAN_POINT ( 'NONE',  ( 1.392837473234412426, 29.83693993229687180, -51.60511860951399399 ) ) ;
#101425=VERTEX_POINT ( 'NONE', #82810 ) ;
#101427=MECHANICAL_DESIGN_GEOMETRIC_PRESENTATION_REPRESENTATION('',(#124084),#46593);
#101437=CARTESIAN_POINT ( 'NONE',  ( -3.735172737399431091E-16, -6.100000000000006750, -64.92279855667830191 ) ) ;
#101458=CARTESIAN_POINT ( 'NONE',  ( -38.00000000000001421, 12.34694845685046438, -2.099999999999999645 ) ) ;
#101479=CIRCLE ( 'NONE', #136999, 61.99999999999998579 ) ;
#101519=CARTESIAN_POINT ( 'NONE',  ( 22.81625015709510151, -31.40387420917324590, -7.924999997268812990 ) ) ;
#101554=DIRECTION ( 'NONE',  ( -0.000000000000000000, -0.000000000000000000, 1.000000000000000000 ) ) ;
#101584=FACE_BOUND ( 'NONE', #42839, .T. ) ;
#101605=CARTESIAN_POINT ( 'NONE',  ( -19.99999999999998224, -190.0000000000000000, 0.000000000000000000 ) ) ;
#101613=EDGE_CURVE ( 'NONE', #140935, #112813, #171147, .T. ) ;
#101645=VERTEX_POINT ( 'NONE', #53486 ) ;
#101648=DIRECTION ( 'NONE',  ( -0.000000000000000000, -0.000000000000000000, 1.000000000000000000 ) ) ;
#101680=CYLINDRICAL_SURFACE ( 'NONE', #65965, 38.00000000000000000 ) ;
#101700=CARTESIAN_POINT ( 'NONE',  ( 36.91746824999999887, -11.99521256947793546, -1.724999997268813479 ) ) ;
#101708=ORIENTED_EDGE ( 'NONE', *, *, #125853, .T. ) ;
#101723=CIRCLE ( 'NONE', #195421, 31.90000000000003411 ) ;
#101763=CARTESIAN_POINT ( 'NONE',  ( 28.98522958361494872, -0.5143648618586993404, -49.56847006845436709 ) ) ;
#101775=CARTESIAN_POINT ( 'NONE',  ( 2.500000000000000000, -105.0000000000000000, 12.00000000000000355 ) ) ;
#101788=EDGE_LOOP ( 'NONE', ( #61221, #196968, #129777 ) ) ;
#101794=CIRCLE ( 'NONE', #121128, 6.100000000000006750 ) ;
#101835=ORIENTED_EDGE ( 'NONE', *, *, #63738, .T. ) ;
#101847=EDGE_CURVE ( 'NONE', #16723, #94189, #148502, .T. ) ;
#101872=VECTOR ( 'NONE', #45759, 1000.000000000000000 ) ;
#101913=CARTESIAN_POINT ( 'NONE',  ( -21.90755247610416490, -31.73190472514682270, -17.16613178567115483 ) ) ;
#101919=DIRECTION ( 'NONE',  ( -1.000000000000000000, 0.000000000000000000, 0.000000000000000000 ) ) ;
#101941=LINE ( 'NONE', #166619, #95199 ) ;
#101947=EDGE_LOOP ( 'NONE', ( #164860, #111827, #169160, #95420 ) ) ;
#101949=ORIENTED_EDGE ( 'NONE', *, *, #468, .F. ) ;
#101957=CARTESIAN_POINT ( 'NONE',  ( -11.74264578624799782, -36.14014761921581709, -7.349999994537626868 ) ) ;
#101964=CARTESIAN_POINT ( 'NONE',  ( 6.091322673906378604, -4.048585108065108074, -62.28976796517032000 ) ) ;
#101996=CARTESIAN_POINT ( 'NONE',  ( 9.687362902255731711, -9.687362902255694408, -60.44446360152740993 ) ) ;
#102008=CARTESIAN_POINT ( 'NONE',  ( -36.91746825000000598, 11.99521256947798520, -3.224999997268813257 ) ) ;
#102018=CARTESIAN_POINT ( 'NONE',  ( -27.16368555717297184, -26.59078835260040208, -15.56371235017458510 ) ) ;
#102031=CARTESIAN_POINT ( 'NONE',  ( -27.75718128995210776, -28.53842127823990182, -16.93139376986094291 ) ) ;
#102034=CARTESIAN_POINT ( 'NONE',  ( 19.38985940809749309, -32.68077955211924035, -24.99999999999992895 ) ) ;
#102046=CARTESIAN_POINT ( 'NONE',  ( 23.51385019162036016, -1.374935097489230484, -54.82293943248596690 ) ) ;
#102066=CARTESIAN_POINT ( 'NONE',  ( -0.2002935562469364550, -6.100000000000008527, -62.50719930893266962 ) ) ;
#102097=DIRECTION ( 'NONE',  ( -1.000000000000000000, 0.000000000000000000, 0.000000000000000000 ) ) ;
#102120=EDGE_CURVE ( 'NONE', #35858, #28673, #57504, .T. ) ;
#102160=CARTESIAN_POINT ( 'NONE',  ( 23.48529157249599564, 32.32473071737754111, -6.700000000000000178 ) ) ;
#102163=CARTESIAN_POINT ( 'NONE',  ( -29.12359114459359688, -24.18000288461016112, -21.55587802759511717 ) ) ;
#102181=VERTEX_POINT ( 'NONE', #197017 ) ;
#102184=CYLINDRICAL_SURFACE ( 'NONE', #195888, 1.500000000000001332 ) ;
#102211=CARTESIAN_POINT ( 'NONE',  ( 20.08125529445640467, 22.02279270211222340, -51.67964572521218969 ) ) ;
#102228=LINE ( 'NONE', #179090, #37310 ) ;
#102232=CARTESIAN_POINT ( 'NONE',  ( -4.521033265328978423, -6.642290809010376051, -64.18582806809564545 ) ) ;
#102251=ORIENTED_EDGE ( 'NONE', *, *, #88509, .F. ) ;
#102292=ORIENTED_EDGE ( 'NONE', *, *, #80974, .F. ) ;
#102348=CYLINDRICAL_SURFACE ( 'NONE', #11359, 6.100000000000006750 ) ;
#102375=AXIS2_PLACEMENT_3D ( 'NONE', #128842, #97496, #19694 ) ;
#102427=CARTESIAN_POINT ( 'NONE',  ( -9.687362902255793884, -9.687362902255632235, -62.58071313852362039 ) ) ;
#102466=DIRECTION ( 'NONE',  ( -1.000000000000000000, 1.065814103640150121E-14, 0.000000000000000000 ) ) ;
#102475=CARTESIAN_POINT ( 'NONE',  ( -29.86685920354755552, 21.69954338932564397, -8.824999997268815122 ) ) ;
#102484=CARTESIAN_POINT ( 'NONE',  ( 36.54539699253855645, -20.47674586971434962, -19.42837732572175113 ) ) ;
#102485=CARTESIAN_POINT ( 'NONE',  ( -20.43538597629143538, -20.43538597629106945, -49.67367017693150189 ) ) ;
#102513=CARTESIAN_POINT ( 'NONE',  ( -18.70878831527339159, -37.83292004501378614, -19.76830273372895164 ) ) ;
#102535=CARTESIAN_POINT ( 'NONE',  ( -3.503282210674335317, -48.86437366581480291, -34.99999999999999289 ) ) ;
#102538=CARTESIAN_POINT ( 'NONE',  ( 22.81625015709510151, -31.40387420917324590, -3.924999997268811658 ) ) ;
#102578=FACE_OUTER_BOUND ( 'NONE', #178273, .T. ) ;
#102619=DIRECTION ( 'NONE',  ( -0.000000000000000000, -0.000000000000000000, -1.000000000000000000 ) ) ;
#102625=CIRCLE ( 'NONE', #128407, 5.000000000000000000 ) ;
#102686=CARTESIAN_POINT ( 'NONE',  ( -12.56216403881615307, -41.81473846791989502, -20.79002063418674240 ) ) ;
#102695=CARTESIAN_POINT ( 'NONE',  ( -38.00000000000000711, 2.893978650043524126E-14, -18.00000000000000000 ) ) ;
#102710=CARTESIAN_POINT ( 'NONE',  ( -33.33806273211352078, -22.10771529531805513, -23.55827701141446440 ) ) ;
#102768=CARTESIAN_POINT ( 'NONE',  ( 31.05479031690787650, -1.359215367441156008, -46.85916094508149143 ) ) ;
#102779=CARTESIAN_POINT ( 'NONE',  ( -3.573655867282028392E-15, 2.428612866367529932E-14, -18.00000000000000000 ) ) ;
#102786=VERTEX_POINT ( 'NONE', #136321 ) ;
#102918=CARTESIAN_POINT ( 'NONE',  ( 0.000000000000000000, 0.000000000000000000, -49.67367017693150189 ) ) ;
#102940=EDGE_CURVE ( 'NONE', #147808, #138825, #17384, .T. ) ;
#102954=CARTESIAN_POINT ( 'NONE',  ( -38.00000000000001421, -12.34694845685042708, -9.649999994537626691 ) ) ;
#102960=DIRECTION ( 'NONE',  ( -0.000000000000000000, -0.000000000000000000, -1.000000000000000000 ) ) ;
#102970=VERTEX_POINT ( 'NONE', #101996 ) ;
#102971=CARTESIAN_POINT ( 'NONE',  ( -1.232294487434663965, -29.53952216915897466, -51.94279119241696208 ) ) ;
#103001=ORIENTED_EDGE ( 'NONE', *, *, #49944, .F. ) ;
#103004=CARTESIAN_POINT ( 'NONE',  ( 36.91746824999999177, 2.880721459617395097E-14, -4.124999997268813168 ) ) ;
#103005=CARTESIAN_POINT ( 'NONE',  ( 9.687362902255733488, -9.687362902255692632, -64.92279855667830191 ) ) ;
#103009=AXIS2_PLACEMENT_3D ( 'NONE', #108161, #152680, #90023 ) ;
#103025=ORIENTED_EDGE ( 'NONE', *, *, #133623, .F. ) ;
#103030=CARTESIAN_POINT ( 'NONE',  ( -22.61240241995035305, -33.77560033877102796, -17.98683046886889514 ) ) ;
#103031=VERTEX_POINT ( 'NONE', #149500 ) ;
#103045=CARTESIAN_POINT ( 'NONE',  ( 24.06132300323557516, -0.8180345313831565157, -54.40060964255543041 ) ) ;
#103066=DIRECTION ( 'NONE',  ( -1.000000000000000000, 0.000000000000000000, 0.000000000000000000 ) ) ;
#103099=EDGE_CURVE ( 'NONE', #3755, #102786, #33545, .T. ) ;
#103159=AXIS2_PLACEMENT_3D ( 'NONE', #21738, #40905, #100563 ) ;
#103184=ORIENTED_EDGE ( 'NONE', *, *, #40462, .T. ) ;
#103187=CARTESIAN_POINT ( 'NONE',  ( 0.000000000000000000, -78.67194367458512261, -23.00000000000000000 ) ) ;
#103212=CARTESIAN_POINT ( 'NONE',  ( 21.73741105231470527, 22.97983228106259901, -49.48322453030139911 ) ) ;
#103214=DIRECTION ( 'NONE',  ( -0.000000000000000000, -0.000000000000000000, 1.000000000000000000 ) ) ;
#103233=CARTESIAN_POINT ( 'NONE',  ( -4.926632765927992708, -6.813239905315497502, -64.10665255646803473 ) ) ;
#103238=EDGE_LOOP ( 'NONE', ( #125765, #54004, #39848, #146693, #120559 ) ) ;
#103304=DIRECTION ( 'NONE',  ( 0.000000000000000000, 0.000000000000000000, 1.000000000000000000 ) ) ;
#103333=PLANE ( 'NONE',  #83777 ) ;
#103351=EDGE_CURVE ( 'NONE', #150928, #120381, #184107, .T. ) ;
#103416=DIRECTION ( 'NONE',  ( 1.000000000000000000, 0.000000000000000000, 0.000000000000000000 ) ) ;
#103441=CIRCLE ( 'NONE', #16254, 69.99999999999997158 ) ;
#103451=DIRECTION ( 'NONE',  ( 0.000000000000000000, -0.000000000000000000, -1.000000000000000000 ) ) ;
#103455=DIRECTION ( 'NONE',  ( -1.000000000000000000, 0.000000000000000000, 0.000000000000000000 ) ) ;
#103472=AXIS2_PLACEMENT_3D ( 'NONE', #113743, #81403, #65264 ) ;
#103479=CARTESIAN_POINT ( 'NONE',  ( -11.74264578624800670, 36.14014761921585972, -0.3999999999999999112 ) ) ;
#103484=CYLINDRICAL_SURFACE ( 'NONE', #76238, 13.70000000000001528 ) ;
#103505=ADVANCED_FACE ( 'NONE', ( #53455 ), #10904, .F. ) ;
#103507=CARTESIAN_POINT ( 'NONE',  ( -4.000000000000000888, -165.0000000000000000, 12.00000000000000355 ) ) ;
#103511=ORIENTED_EDGE ( 'NONE', *, *, #173803, .F. ) ;
#103523=EDGE_CURVE ( 'NONE', #157973, #100403, #20538, .T. ) ;
#103541=CARTESIAN_POINT ( 'NONE',  ( 22.81625015709510151, -31.40387420917324590, -5.924999997268812990 ) ) ;
#103611=ORIENTED_EDGE ( 'NONE', *, *, #158176, .F. ) ;
#103619=FACE_OUTER_BOUND ( 'NONE', #78686, .T. ) ;
#103695=CARTESIAN_POINT ( 'NONE',  ( -15.06137443927361019, -15.06137443927335440, -58.85720012050613548 ) ) ;
#103714=CARTESIAN_POINT ( 'NONE',  ( -32.20268589050812125, -23.72850345486251200, -20.40273169984848778 ) ) ;
#103721=ORIENTED_EDGE ( 'NONE', *, *, #111598, .T. ) ;
#103732=CARTESIAN_POINT ( 'NONE',  ( 9.128739734650142879, -39.45218800495355538, -25.46847458086233829 ) ) ;
#103795=ORIENTED_EDGE ( 'NONE', *, *, #105746, .T. ) ;
#103843=ORIENTED_EDGE ( 'NONE', *, *, #52799, .T. ) ;
#103847=( NAMED_UNIT ( * ) PLANE_ANGLE_UNIT ( ) SI_UNIT ( $, .RADIAN. ) );
#103918=CARTESIAN_POINT ( 'NONE',  ( 12.22613352584845359, -10.45440487129810236, -61.62309247082062313 ) ) ;
#103919=DIRECTION ( 'NONE',  ( -0.000000000000000000, -0.000000000000000000, 1.000000000000000000 ) ) ;
#103955=CARTESIAN_POINT ( 'NONE',  ( 11.74264578624799427, 36.14014761921585972, -4.349999994537626868 ) ) ;
#103959=EDGE_CURVE ( 'NONE', #177278, #44838, #183553, .T. ) ;
#103968=CARTESIAN_POINT ( 'NONE',  ( -11.43209428340597711, 9.409695640424857288, -59.99679127084682051 ) ) ;
#103979=DIRECTION ( 'NONE',  ( 0.000000000000000000, 0.000000000000000000, -1.000000000000000000 ) ) ;
#103995=DIRECTION ( 'NONE',  ( 1.000000000000000000, 0.000000000000000000, 0.000000000000000000 ) ) ;
#104006=CARTESIAN_POINT ( 'NONE',  ( -22.81625015709510507, 31.40387420917330275, -7.424999997268812102 ) ) ;
#104007=DIRECTION ( 'NONE',  ( 1.000000000000000000, 0.000000000000000000, 0.000000000000000000 ) ) ;
#104028=CARTESIAN_POINT ( 'NONE',  ( -27.05031264677035807, -29.22974442244507998, -16.95124367203715110 ) ) ;
#104042=CARTESIAN_POINT ( 'NONE',  ( -0.9968436689772768311, -8.725106586199784076, -64.02420483255117745 ) ) ;
#104054=CARTESIAN_POINT ( 'NONE',  ( 4.313351365237949153, 4.313351365237946489, -64.92279855667830191 ) ) ;
#104055=CARTESIAN_POINT ( 'NONE',  ( 0.000000000000000000, 0.000000000000000000, -18.00000000000000000 ) ) ;
#104077=ORIENTED_EDGE ( 'NONE', *, *, #62849, .T. ) ;
#104140=DIRECTION ( 'NONE',  ( -0.000000000000000000, -0.000000000000000000, 1.000000000000000000 ) ) ;
#104158=CARTESIAN_POINT ( 'NONE',  ( -6.565741541539673598, 4.457937930945857552, -62.16217994089669219 ) ) ;
#104162=CARTESIAN_POINT ( 'NONE',  ( 1.067013306609913448, 31.46962149133000608, -46.27433572153971397 ) ) ;
#104206=CARTESIAN_POINT ( 'NONE',  ( 22.46606745562067431, 22.64734518408110020, -49.13275782002543934 ) ) ;
#104211=CARTESIAN_POINT ( 'NONE',  ( -38.00000000000000711, 2.428612866367529932E-14, -4.000000000000000000 ) ) ;
#104250=CARTESIAN_POINT ( 'NONE',  ( -6.297097159419607237, 4.175862767829939592, -64.28037419727766633 ) ) ;
#104320=ORIENTED_EDGE ( 'NONE', *, *, #137670, .T. ) ;
#104342=CARTESIAN_POINT ( 'NONE',  ( 0.000000000000000000, 0.000000000000000000, -64.92279855667830191 ) ) ;
#104351=DIRECTION ( 'NONE',  ( 1.000000000000000000, 0.000000000000000000, 0.000000000000000000 ) ) ;
#104372=ADVANCED_FACE ( 'NONE', ( #14693 ), #171564, .F. ) ;
#104408=VERTEX_POINT ( 'NONE', #178340 ) ;
#104437=DIRECTION ( 'NONE',  ( 0.000000000000000000, 1.000000000000000000, 0.000000000000000000 ) ) ;
#104446=B_SPLINE_CURVE_WITH_KNOTS ( 'NONE', 3,
 ( #198927, #108892, #124046, #30070, #48229, #185745, #155400, #60395 ),
 .UNSPECIFIED., .F., .F.,
 ( 4, 2, 2, 4 ),
 ( 0.004065040094758672930, 0.004372354996941527766, 0.004679669899124381735, 0.005294299703490097479 ),
 .UNSPECIFIED. ) ;
#104453=CARTESIAN_POINT ( 'NONE',  ( 13.74275686049843159, -0.4100021152176986372, -60.42614020214174531 ) ) ;
#104457=DIRECTION ( 'NONE',  ( 0.000000000000000000, -0.000000000000000000, -1.000000000000000000 ) ) ;
#104471=CARTESIAN_POINT ( 'NONE',  ( 23.48529157249599919, 32.32473071737754111, -8.700000000000002842 ) ) ;
#104525=ADVANCED_FACE ( 'NONE', ( #30915 ), #125895, .F. ) ;
#104526=ORIENTED_EDGE ( 'NONE', *, *, #101847, .T. ) ;
#104598=ORIENTED_EDGE ( 'NONE', *, *, #32592, .T. ) ;
#104703=CARTESIAN_POINT ( 'NONE',  ( -22.81625015709510507, 31.40387420917330275, -8.924999997268812990 ) ) ;
#104709=ORIENTED_EDGE ( 'NONE', *, *, #99957, .T. ) ;
#104712=LINE ( 'NONE', #122844, #84873 ) ;
#104720=CARTESIAN_POINT ( 'NONE',  ( 11.70497261681111034, -44.13276428439503007, -23.15274968896633467 ) ) ;
#104722=FACE_OUTER_BOUND ( 'NONE', #157490, .T. ) ;
#104733=AXIS2_PLACEMENT_3D ( 'NONE', #87916, #60551, #102097 ) ;
#104738=ORIENTED_EDGE ( 'NONE', *, *, #108116, .F. ) ;
#104764=CIRCLE ( 'NONE', #140241, 214.0437394197456342 ) ;
#104777=LINE ( 'NONE', #133112, #137080 ) ;
#104846=ADVANCED_FACE ( 'NONE', ( #175384 ), #88392, .T. ) ;
#104924=DIRECTION ( 'NONE',  ( 5.204170427930421283E-16, 0.000000000000000000, -1.000000000000000000 ) ) ;
#104934=CIRCLE ( 'NONE', #133964, 69.99999999999998579 ) ;
#104940=ORIENTED_EDGE ( 'NONE', *, *, #127970, .F. ) ;
#104942=EDGE_LOOP ( 'NONE', ( #60868, #168666, #32770, #143732 ) ) ;
#104944=FACE_OUTER_BOUND ( 'NONE', #93490, .T. ) ;
#104948=CARTESIAN_POINT ( 'NONE',  ( 11.40812507854755253, -35.11059874428192273, -2.524999997268813523 ) ) ;
#104961=CARTESIAN_POINT ( 'NONE',  ( -9.760750291312424665, 9.613975513199005007, -60.44446360152740283 ) ) ;
#104965=DIRECTION ( 'NONE',  ( 3.469446951953612217E-15, 0.000000000000000000, -1.000000000000000000 ) ) ;
#104972=CARTESIAN_POINT ( 'NONE',  ( -21.39352396646987486, 0.5319302666795560075, -58.79417398750191381 ) ) ;
#104998=CARTESIAN_POINT ( 'NONE',  ( 22.81625015709509441, 31.40387420917330275, -7.824999997268813345 ) ) ;
#104999=DIRECTION ( 'NONE',  ( 0.000000000000000000, 0.000000000000000000, 1.000000000000000000 ) ) ;
#105022=CARTESIAN_POINT ( 'NONE',  ( -29.81671572245832280, -26.02765724076686737, -18.90727510135208078 ) ) ;
#105054=AXIS2_PLACEMENT_3D ( 'NONE', #169077, #62892, #17402 ) ;
#105058=CARTESIAN_POINT ( 'NONE',  ( -193.3062444957834884, -155.7167183371838064, -25.00000000000000000 ) ) ;
#105072=ORIENTED_EDGE ( 'NONE', *, *, #111223, .T. ) ;
#105086=CARTESIAN_POINT ( 'NONE',  ( -37.66961640367473052, 5.000000000000023981, -25.00000000000000000 ) ) ;
#105089=LINE ( 'NONE', #137402, #24056 ) ;
#105150=CARTESIAN_POINT ( 'NONE',  ( -6.434671708797603529, 6.434671708797564449, -61.89430850415821794 ) ) ;
#105154=CARTESIAN_POINT ( 'NONE',  ( -26.88621168971704378, -26.45719545518177185, -20.39628335082763044 ) ) ;
#105157=DIRECTION ( 'NONE',  ( -0.000000000000000000, -0.000000000000000000, 1.000000000000000000 ) ) ;
#105172=CARTESIAN_POINT ( 'NONE',  ( 6.856101608890801443E-16, -78.63162257080495010, -22.99999901186701123 ) ) ;
#105199=CARTESIAN_POINT ( 'NONE',  ( 19.24578484527059175, -180.9428398739492820, 0.000000000000000000 ) ) ;
#105213=DIRECTION ( 'NONE',  ( -0.000000000000000000, -0.000000000000000000, 1.000000000000000000 ) ) ;
#105215=CARTESIAN_POINT ( 'NONE',  ( -11.30153831258471442, -180.0000000000000000, -15.00000000000000178 ) ) ;
#105218=CARTESIAN_POINT ( 'NONE',  ( 6.017829804060273347, -47.35862344248570821, -22.79591852006818442 ) ) ;
#105241=DIRECTION ( 'NONE',  ( 0.000000000000000000, 0.000000000000000000, 1.000000000000000000 ) ) ;
#105272=SPHERICAL_SURFACE ( 'NONE', #72434, 8.000000000000000000 ) ;
#105275=CARTESIAN_POINT ( 'NONE',  ( 16.12203461105332636, 16.12203461105328017, -64.92279855667830191 ) ) ;
#105299=AXIS2_PLACEMENT_3D ( 'NONE', #112732, #148080, #9571 ) ;
#105320=DIRECTION ( 'NONE',  ( 1.000000000000000000, 0.000000000000000000, 0.000000000000000000 ) ) ;
#105355=AXIS2_PLACEMENT_3D ( 'NONE', #118362, #83002, #191197 ) ;
#105399=ORIENTED_EDGE ( 'NONE', *, *, #6145, .F. ) ;
#105416=EDGE_CURVE ( 'NONE', #146440, #197049, #111035, .T. ) ;
#105424=CARTESIAN_POINT ( 'NONE',  ( 13.70000000000001528, 0.000000000000000000, -60.44446360152740283 ) ) ;
#105436=CARTESIAN_POINT ( 'NONE',  ( 15.31758167559927841, -14.84543115662826374, -58.83804107897447011 ) ) ;
#105442=( BOUNDED_CURVE ( )  B_SPLINE_CURVE ( 2, ( #138979, #32809, #94460, #45985, #125802, #108644, #33796, #169317, #187504, #155152, #18637 ),
 .UNSPECIFIED., .F., .F. ) 
 B_SPLINE_CURVE_WITH_KNOTS ( ( 3, 2, 2, 2, 2, 3 ),
 ( 0.9000000000000000222, 0.9200000000000000400, 0.9399999999999999467, 0.9599999999999999645, 0.9799999999999999822, 1.000000000000000000 ),
 .UNSPECIFIED. ) 
 CURVE ( )  GEOMETRIC_REPRESENTATION_ITEM ( )  RATIONAL_B_SPLINE_CURVE ( ( 1.000000000000000000, 0.9510565162951535312, 1.000000000000000000, 0.9510565162951535312, 1.000000000000000000, 0.9510565162951535312, 1.000000000000000000, 0.9510565162951535312, 1.000000000000000000, 0.9510565162951535312, 1.000000000000000000 ) ) 
 REPRESENTATION_ITEM ( '' )  );
#105444=DIRECTION ( 'NONE',  ( -0.000000000000000000, -0.000000000000000000, 1.000000000000000000 ) ) ;
#105458=CARTESIAN_POINT ( 'NONE',  ( 30.74264578624800137, -22.33583958711395212, -7.200000000000001066 ) ) ;
#105484=DIRECTION ( 'NONE',  ( -0.000000000000000000, -0.000000000000000000, -1.000000000000000000 ) ) ;
#105488=EDGE_LOOP ( 'NONE', ( #11182, #59994, #56685, #20805 ) ) ;
#105517=CARTESIAN_POINT ( 'NONE',  ( -36.91746825000000598, 2.428612866367529932E-14, -10.62499999726881406 ) ) ;
#105590=DIRECTION ( 'NONE',  ( 0.000000000000000000, 0.000000000000000000, 1.000000000000000000 ) ) ;
#105598=CARTESIAN_POINT ( 'NONE',  ( 12.24802307403557577, -10.74802307403608737, -59.32879157176802920 ) ) ;
#105638=VERTEX_POINT ( 'NONE', #55034 ) ;
#105647=CARTESIAN_POINT ( 'NONE',  ( -24.50241233882722369, -28.74340065771546904, -20.80149134688043588 ) ) ;
#105653=EDGE_LOOP ( 'NONE', ( #110649, #141516, #70461, #162338 ) ) ;
#105686=ORIENTED_EDGE ( 'NONE', *, *, #131641, .T. ) ;
#105689=CARTESIAN_POINT ( 'NONE',  ( -36.91746825000000598, 2.428612866367529932E-14, -8.624999997268814056 ) ) ;
#105746=EDGE_CURVE ( 'NONE', #197536, #125394, #82720, .T. ) ;
#105812=AXIS2_PLACEMENT_3D ( 'NONE', #160641, #158640, #81776 ) ;
#105844=EDGE_CURVE ( 'NONE', #176035, #115704, #154292, .T. ) ;
#105868=ORIENTED_EDGE ( 'NONE', *, *, #156887, .T. ) ;
#105912=CARTESIAN_POINT ( 'NONE',  ( -0.5040881997803867698, -16.61636759701970689, -59.17093420172795248 ) ) ;
#105934=CARTESIAN_POINT ( 'NONE',  ( 29.86685920354754487, 21.69954338932564752, -5.924999997268813878 ) ) ;
#105985=CARTESIAN_POINT ( 'NONE',  ( 36.91746824999999177, 11.99521256947799230, -10.02499999726881086 ) ) ;
#106031=CARTESIAN_POINT ( 'NONE',  ( 8.788868155854864028, -0.9199430937698539479, -64.01178436185549003 ) ) ;
#106126=B_SPLINE_CURVE_WITH_KNOTS ( 'NONE', 3,
 ( #72352, #88504, #167352, #150200, #136015, #10688, #134026, #197688, #182523, #44004, #11698, #135037, #196713, #102686, #164373, #87510, #12683, #195719, #136993, #121817, #117859, #60149, #179550, #28850 ),
 .UNSPECIFIED., .F., .F.,
 ( 4, 2, 2, 2, 2, 2, 2, 2, 2, 2, 2, 4 ),
 ( 0.000000000000000000, 0.002210131452840893417, 0.004420262905681786834, 0.008840525811363580608, 0.01326078871704536657, 0.01768105162272715428, 0.02210131452840894198, 0.02652157743409072621, 0.02873170888693162006, 0.03094184033977251391, 0.03315197179261340776, 0.03536210324545430161 ),
 .UNSPECIFIED. ) ;
#106134=CARTESIAN_POINT ( 'NONE',  ( -20.63676584477901699, 20.25987216150948811, -49.65115959356506892 ) ) ;
#106141=B_SPLINE_CURVE_WITH_KNOTS ( 'NONE', 3,
 ( #103695, #71358, #166374, #74355, #135043, #163370, #27870, #12689 ),
 .UNSPECIFIED., .F., .F.,
 ( 4, 2, 2, 4 ),
 ( 2.784816081883512217E-07, 0.0003049387032676472830, 0.0006095989249271061916, 0.001218919368246023033 ),
 .UNSPECIFIED. ) ;
#106237=ORIENTED_EDGE ( 'NONE', *, *, #10139, .T. ) ;
#106258=DIRECTION ( 'NONE',  ( -1.000000000000000000, 0.000000000000000000, 0.000000000000000000 ) ) ;
#106305=AXIS2_PLACEMENT_3D ( 'NONE', #6188, #7186, #99196 ) ;
#106326=CARTESIAN_POINT ( 'NONE',  ( -6.941067294099585006, 1.351053078614677716, -64.37011660792191492 ) ) ;
#106382=VERTEX_POINT ( 'NONE', #173448 ) ;
#106409=CARTESIAN_POINT ( 'NONE',  ( 2.577820198429831642E-15, 9.100000000000001421, -65.00100000000003320 ) ) ;
#106415=CARTESIAN_POINT ( 'NONE',  ( 0.000000000000000000, 0.000000000000000000, -52.65483682830183199 ) ) ;
#106419=CARTESIAN_POINT ( 'NONE',  ( 14.30620887846970746, -1.220661533321876879, -60.18359034246770989 ) ) ;
#106438=CARTESIAN_POINT ( 'NONE',  ( 38.00000000000000711, -12.34694845685040754, -3.100000000000000533 ) ) ;
#106450=DIRECTION ( 'NONE',  ( 0.000000000000000000, -1.000000000000000000, 0.000000000000000000 ) ) ;
#106465=CARTESIAN_POINT ( 'NONE',  ( 18.60204571913743976, -35.35091242066980755, -18.26754506500548558 ) ) ;
#106584=CARTESIAN_POINT ( 'NONE',  ( -21.44208882751384593, -23.00296878542015477, -49.72123984779791783 ) ) ;
#106615=ADVANCED_FACE ( 'NONE', ( #58079 ), #134931, .T. ) ;
#106627=ORIENTED_EDGE ( 'NONE', *, *, #191742, .T. ) ;
#106638=CARTESIAN_POINT ( 'NONE',  ( -16.00769354339768924, -38.20109431699814451, -19.33483434993910066 ) ) ;
#106661=CARTESIAN_POINT ( 'NONE',  ( 22.36951698133467303, -20.26978297296616560, -48.08211468429932012 ) ) ;
#106679=CARTESIAN_POINT ( 'NONE',  ( -22.81625015709509441, -31.40387420917324590, -6.324999997268814234 ) ) ;
#106699=CARTESIAN_POINT ( 'NONE',  ( -9.670372969936114060, -11.80125700695215762, -61.97618590420869111 ) ) ;
#106715=ORIENTED_EDGE ( 'NONE', *, *, #15614, .T. ) ;
#106752=CARTESIAN_POINT ( 'NONE',  ( 23.48529157249599564, 32.32473071737754111, -2.700000000000000178 ) ) ;
#106780=CARTESIAN_POINT ( 'NONE',  ( 12.24802307403546386, -10.94100078822751776, -61.47356435416956799 ) ) ;
#106886=CARTESIAN_POINT ( 'NONE',  ( 1.500000000000124123, 15.01136863746049954, -59.87766023546532068 ) ) ;
#106908=FACE_OUTER_BOUND ( 'NONE', #105653, .T. ) ;
#106915=VERTEX_POINT ( 'NONE', #101210 ) ;
#106917=VERTEX_POINT ( 'NONE', #162899 ) ;
#106923=CARTESIAN_POINT ( 'NONE',  ( -36.91746825000000598, 2.428612866367529932E-14, -3.124999997268813168 ) ) ;
#106930=CARTESIAN_POINT ( 'NONE',  ( 193.3062444957835453, -155.7167183371837496, -15.00000000000000178 ) ) ;
#106935=CARTESIAN_POINT ( 'NONE',  ( 3.920341815485308690, 4.991179326919313652, -62.46637012391575183 ) ) ;
#106945=CARTESIAN_POINT ( 'NONE',  ( -23.50300173439379492, 1.337618122189927927, -57.33987540012260098 ) ) ;
#106971=FACE_OUTER_BOUND ( 'NONE', #68948, .T. ) ;
#106978=CARTESIAN_POINT ( 'NONE',  ( 31.67388030095421314, -20.99825235784043187, -23.44681632512342873 ) ) ;
#106986=ORIENTED_EDGE ( 'NONE', *, *, #188131, .T. ) ;
#107016=EDGE_CURVE ( 'NONE', #28823, #40299, #8580, .T. ) ;
#107053=LINE ( 'NONE', #105086, #96110 ) ;
#107055=CARTESIAN_POINT ( 'NONE',  ( -11.30153831258471442, -180.0000000000000000, -23.00000000000000000 ) ) ;
#107092=EDGE_CURVE ( 'NONE', #6179, #24124, #42256, .T. ) ;
#107157=CARTESIAN_POINT ( 'NONE',  ( -6.100000000000010303, 0.2002935562470000430, -62.50719930893271226 ) ) ;
#107198=ORIENTED_EDGE ( 'NONE', *, *, #154789, .T. ) ;
#107210=CARTESIAN_POINT ( 'NONE',  ( -5.576804854476224094, 3.874965782148136029, -64.41982836185007955 ) ) ;
#107241=B_SPLINE_CURVE_WITH_KNOTS ( 'NONE', 3,
 ( #152186, #45009, #167366, #168342, #13670, #121832, #14664, #95464, #96450, #33804, #77319, #31823, #49971, #186519, #174315, #141963, #142953, #173320, #48979, #110634, #111635, #63140 ),
 .UNSPECIFIED., .F., .F.,
 ( 4, 2, 2, 2, 2, 2, 2, 2, 2, 2, 4 ),
 ( 2.778238173728123515E-07, 0.0002956205979242803109, 0.0005909633720311878793, 0.0008863061461380952310, 0.001181648920245002799, 0.001772334468458817069, 0.002363020016672631556, 0.002953705564886446259, 0.003544391113100260095, 0.004135076661314075232, 0.004725762209527889501 ),
 .UNSPECIFIED. ) ;
#107277=ORIENTED_EDGE ( 'NONE', *, *, #197214, .F. ) ;
#107313=CARTESIAN_POINT ( 'NONE',  ( -9.100000000000003197, 0.1000365528947574634, -63.95112321872120731 ) ) ;
#107371=CARTESIAN_POINT ( 'NONE',  ( 23.48529157249599564, 32.32473071737754111, -8.449999994537627401 ) ) ;
#107396=FACE_OUTER_BOUND ( 'NONE', #198040, .T. ) ;
#107402=CARTESIAN_POINT ( 'NONE',  ( 25.83521962401025007, -30.44105770729786542, -17.07601944841966812 ) ) ;
#107424=CIRCLE ( 'NONE', #55779, 21.30000000000002913 ) ;
#107426=CARTESIAN_POINT ( 'NONE',  ( -23.48529157249599919, -32.32473071737750558, -3.699999999999999734 ) ) ;
#107451=CARTESIAN_POINT ( 'NONE',  ( 22.01160362600695564, -30.88790364210955275, -22.63296439182117581 ) ) ;
#107478=EDGE_LOOP ( 'NONE', ( #109473, #136816, #64481, #175049 ) ) ;
#107496=EDGE_CURVE ( 'NONE', #156506, #147808, #6041, .T. ) ;
#107558=DIRECTION ( 'NONE',  ( -0.000000000000000000, 0.000000000000000000, 1.000000000000000000 ) ) ;
#107567=CARTESIAN_POINT ( 'NONE',  ( -38.00000000000000711, 2.428612866367529932E-14, -9.749999994537626336 ) ) ;
#107603=VERTEX_POINT ( 'NONE', #15024 ) ;
#107616=CARTESIAN_POINT ( 'NONE',  ( -14.20416113189184593, -35.58439206127017229, -22.81347619872354215 ) ) ;
#107640=CARTESIAN_POINT ( 'NONE',  ( 22.97440419758976304, -21.21004173184712727, -46.59523340014560233 ) ) ;
#107648=DIRECTION ( 'NONE',  ( 1.000000000000000000, 0.000000000000000000, 0.000000000000000000 ) ) ;
#107694=ORIENTED_EDGE ( 'NONE', *, *, #83071, .T. ) ;
#107716=AXIS2_PLACEMENT_3D ( 'NONE', #92563, #187595, #49064 ) ;
#107753=CARTESIAN_POINT ( 'NONE',  ( 0.2046014141641599449, 16.68944534439192040, -61.35149151744828089 ) ) ;
#107807=ADVANCED_FACE ( 'NONE', ( #13049 ), #164740, .F. ) ;
#107866=CARTESIAN_POINT ( 'NONE',  ( -4.000000000000000888, -165.0000000000000000, 12.00000000000000355 ) ) ;
#107868=CARTESIAN_POINT ( 'NONE',  ( 20.43538597629129328, 20.43538597629121156, -49.67367017693150189 ) ) ;
#107887=CARTESIAN_POINT ( 'NONE',  ( -1.491100297015943488, -15.38830714838547919, -59.71292413584865244 ) ) ;
#107893=CARTESIAN_POINT ( 'NONE',  ( -21.41434933286226538, -23.00156705360894804, -46.36348427009351525 ) ) ;
#107902=ORIENTED_EDGE ( 'NONE', *, *, #21762, .F. ) ;
#107909=CARTESIAN_POINT ( 'NONE',  ( 11.40812507854754365, 35.11059874428196537, -3.724999997268813701 ) ) ;
#107923=CARTESIAN_POINT ( 'NONE',  ( 4.065169771515699360, 6.132035242901161531, -62.28151743970308729 ) ) ;
#107943=VECTOR ( 'NONE', #54512, 1000.000000000000000 ) ;
#107961=CARTESIAN_POINT ( 'NONE',  ( 0.000000000000000000, -165.0000000000000000, 12.00000000000000355 ) ) ;
#107962=CARTESIAN_POINT ( 'NONE',  ( 0.9971028448357464047, 8.724879486844042020, -64.02424906291095397 ) ) ;
#107969=CARTESIAN_POINT ( 'NONE',  ( -12.21717160642880451, 11.11254985580163357, -61.43205129781978258 ) ) ;
#107982=CARTESIAN_POINT ( 'NONE',  ( -37.24154831888154860, -19.83237144080716519, -19.76300508100580444 ) ) ;
#108006=AXIS2_PLACEMENT_3D ( 'NONE', #139580, #17252, #127396 ) ;
#108079=ORIENTED_EDGE ( 'NONE', *, *, #73257, .F. ) ;
#108085=AXIS2_PLACEMENT_3D ( 'NONE', #20611, #50962, #18643 ) ;
#108112=CARTESIAN_POINT ( 'NONE',  ( 0.6176563088794523315, 29.02844413588608319, -49.51499673148455827 ) ) ;
#108116=EDGE_CURVE ( 'NONE', #143210, #190550, #149562, .T. ) ;
#108147=ORIENTED_EDGE ( 'NONE', *, *, #139759, .F. ) ;
#108153=CARTESIAN_POINT ( 'NONE',  ( -6.139906835403841967, 0.3968392070110091097, -62.49911542708240120 ) ) ;
#108161=CARTESIAN_POINT ( 'NONE',  ( 0.000000000000000000, 0.000000000000000000, -64.53213882399991519 ) ) ;
#108163=CARTESIAN_POINT ( 'NONE',  ( 24.24152472029838634, -0.4285070731208356909, -56.81472536503797954 ) ) ;
#108167=VECTOR ( 'NONE', #5880, 1000.000000000000000 ) ;
#108188=ORIENTED_EDGE ( 'NONE', *, *, #67646, .F. ) ;
#108208=PRODUCT_DEFINITION_FORMATION_WITH_SPECIFIED_SOURCE ( 'ANY', '', #113205, .NOT_KNOWN. ) ;
#108211=CARTESIAN_POINT ( 'NONE',  ( -5.283393095647520354, 3.873560230149188488, -64.45999282322711110 ) ) ;
#108216=CARTESIAN_POINT ( 'NONE',  ( -24.26175155739904099, -32.05389003868044284, -17.42962289376371743 ) ) ;
#108223=EDGE_LOOP ( 'NONE', ( #115914, #137718, #99539, #41808 ) ) ;
#108232=VECTOR ( 'NONE', #81538, 1000.000000000000000 ) ;
#108256=CARTESIAN_POINT ( 'NONE',  ( -16.68945015508926843, 0.2045547421927693954, -61.35148950497488585 ) ) ;
#108276=DIRECTION ( 'NONE',  ( 1.000000000000000000, 0.000000000000000000, 0.000000000000000000 ) ) ;
#108308=CARTESIAN_POINT ( 'NONE',  ( -30.74264578624800492, 22.33583958711400186, -3.949999994537626957 ) ) ;
#108318=CARTESIAN_POINT ( 'NONE',  ( 19.24578484527059175, -180.9428398739492820, -15.00000000000000178 ) ) ;
#108352=DIRECTION ( 'NONE',  ( 1.000000000000000000, 0.000000000000000000, 0.000000000000000000 ) ) ;
#108367=ADVANCED_FACE ( 'NONE', ( #149078 ), #57068, .T. ) ;
#108372=ORIENTED_EDGE ( 'NONE', *, *, #5508, .T. ) ;
#108377=CARTESIAN_POINT ( 'NONE',  ( 38.00000000000008527, 12.34694845685035069, -8.649999994537628467 ) ) ;
#108411=CARTESIAN_POINT ( 'NONE',  ( 15.84196527238554353, -1.359015117358377323, -59.51370404797111036 ) ) ;
#108421=CARTESIAN_POINT ( 'NONE',  ( -17.44568526726164848, 16.83584321579681742, -56.81531555676559009 ) ) ;
#108430=CARTESIAN_POINT ( 'NONE',  ( -38.00000000000001421, -12.34694845685042708, -7.900000000000001243 ) ) ;
#108454=CARTESIAN_POINT ( 'NONE',  ( 20.92307141426025296, -31.70153649905323334, -23.60833562325456825 ) ) ;
#108485=CARTESIAN_POINT ( 'NONE',  ( 1.500000000000005329, 15.20000000000001883, -61.96904110198155280 ) ) ;
#108514=AXIS2_PLACEMENT_3D ( 'NONE', #114600, #51936, #176297 ) ;
#108524=CARTESIAN_POINT ( 'NONE',  ( 9.100000000000003197, -0.1001428631146442511, -61.89430850415823215 ) ) ;
#108555=ORIENTED_EDGE ( 'NONE', *, *, #44393, .F. ) ;
#108568=CIRCLE ( 'NONE', #140889, 40.00000000000000711 ) ;
#108573=CARTESIAN_POINT ( 'NONE',  ( -20.13687146691627561, -33.41269836094262047, -11.42148495485635529 ) ) ;
#108606=ORIENTED_EDGE ( 'NONE', *, *, #158775, .T. ) ;
#108611=CARTESIAN_POINT ( 'NONE',  ( 6.434671708797586653, 6.434671708797580436, -64.92279855667830191 ) ) ;
#108621=CARTESIAN_POINT ( 'NONE',  ( -20.12333042654506343, -32.04799867105109712, -20.24659421909778700 ) ) ;
#108644=CARTESIAN_POINT ( 'NONE',  ( 3.766062262543149401E-15, -39.95556452105413570, -9.500000000000000000 ) ) ;
#108663=VECTOR ( 'NONE', #44667, 1000.000000000000000 ) ;
#108681=CARTESIAN_POINT ( 'NONE',  ( 25.49187754477041779, -30.53313611124049487, -20.74730905734758224 ) ) ;
#108714=AXIS2_PLACEMENT_3D ( 'NONE', #20169, #78854, #127340 ) ;
#108728=CARTESIAN_POINT ( 'NONE',  ( -193.3062444957834884, -155.7167183371838064, 0.000000000000000000 ) ) ;
#108737=( BOUNDED_CURVE ( )  B_SPLINE_CURVE ( 2, ( #187024, #44753, #48495, #91219, #157652, #142470, #110149, #113116, #65627, #168090, #112135 ),
 .UNSPECIFIED., .F., .T. ) 
 B_SPLINE_CURVE_WITH_KNOTS ( ( 3, 2, 2, 2, 2, 3 ),
 ( 0.4000000000000000222, 0.4199999999999999845, 0.4400000000000000577, 0.4600000000000000755, 0.4800000000000000933, 0.5000000000000001110 ),
 .UNSPECIFIED. ) 
 CURVE ( )  GEOMETRIC_REPRESENTATION_ITEM ( )  RATIONAL_B_SPLINE_CURVE ( ( 1.000000000000000000, 0.9510565162951535312, 1.000000000000000000, 0.9510565162951535312, 1.000000000000000000, 0.9510565162951535312, 1.000000000000000000, 0.9510565162951535312, 1.000000000000000000, 0.9510565162951533091, 1.000000000000000222 ) ) 
 REPRESENTATION_ITEM ( '' )  );
#108797=EDGE_LOOP ( 'NONE', ( #101708, #70995, #154186, #62470 ) ) ;
#108813=AXIS2_PLACEMENT_3D ( 'NONE', #50132, #110796, #21778 ) ;
#108892=CARTESIAN_POINT ( 'NONE',  ( 17.62203461105333346, -16.21325560958408474, -54.50601694470664427 ) ) ;
#108901=CARTESIAN_POINT ( 'NONE',  ( 0.8180779778021126658, 21.52520729097319574, -58.70525297292005718 ) ) ;
#108912=CARTESIAN_POINT ( 'NONE',  ( 0.000000000000000000, 0.000000000000000000, -64.92279855667830191 ) ) ;
#108916=CARTESIAN_POINT ( 'NONE',  ( -29.86685920354755552, 21.69954338932564397, -3.324999997268813345 ) ) ;
#108929=DIRECTION ( 'NONE',  ( 0.000000000000000000, 0.000000000000000000, 1.000000000000000000 ) ) ;
#108945=CARTESIAN_POINT ( 'NONE',  ( -21.30000000000002913, 2.244099063931684814E-13, -56.46919128290398504 ) ) ;
#108949=VECTOR ( 'NONE', #179646, 1000.000000000000000 ) ;
#108964=CARTESIAN_POINT ( 'NONE',  ( 22.81625015709510151, -31.40387420917324590, -8.424999997268812990 ) ) ;
#108966=FACE_OUTER_BOUND ( 'NONE', #147751, .T. ) ;
#108968=VERTEX_POINT ( 'NONE', #143310 ) ;
#109000=ORIENTED_EDGE ( 'NONE', *, *, #49532, .T. ) ;
#109084=EDGE_LOOP ( 'NONE', ( #40622, #141025, #96405, #100488, #178900 ) ) ;
#109090=CIRCLE ( 'NONE', #34757, 10.00000000000000000 ) ;
#109112=CYLINDRICAL_SURFACE ( 'NONE', #61163, 216.0437394197456911 ) ;
#109116=CARTESIAN_POINT ( 'NONE',  ( -22.96531869715557761, 21.81714873624716233, -45.99103957044147961 ) ) ;
#109119=CARTESIAN_POINT ( 'NONE',  ( 6.874011537017776341, -5.570592230301131487, -61.95613518020381605 ) ) ;
#109146=ADVANCED_FACE ( 'NONE', ( #70235 ), #59098, .T. ) ;
#109155=DIRECTION ( 'NONE',  ( -0.000000000000000000, 0.000000000000000000, 1.000000000000000000 ) ) ;
#109163=CARTESIAN_POINT ( 'NONE',  ( -3.573655867282028392E-15, 2.428612866367529932E-14, -25.00000000000000000 ) ) ;
#109211=CARTESIAN_POINT ( 'NONE',  ( -27.99526582847389022, -28.30548820594175297, -16.92425894792109275 ) ) ;
#109216=CARTESIAN_POINT ( 'NONE',  ( 193.3062444957835453, -155.7167183371837496, -25.00000000000000000 ) ) ;
#109240=DIRECTION ( 'NONE',  ( 0.000000000000000000, 0.000000000000000000, -1.000000000000000000 ) ) ;
#109249=CARTESIAN_POINT ( 'NONE',  ( -16.61713888009425588, 0.5018587474794012904, -61.38171595447353468 ) ) ;
#109286=CARTESIAN_POINT ( 'NONE',  ( -69.65682714487590488, -71.74905178543390605, 0.000000000000000000 ) ) ;
#109361=ORIENTED_EDGE ( 'NONE', *, *, #43460, .T. ) ;
#109446=CARTESIAN_POINT ( 'NONE',  ( 20.00963169948072462, -33.79917020546515971, -17.75419178524472130 ) ) ;
#109473=ORIENTED_EDGE ( 'NONE', *, *, #171282, .F. ) ;
#109480=CIRCLE ( 'NONE', #22321, 61.99999999999998579 ) ;
#109517=CARTESIAN_POINT ( 'NONE',  ( 7.215019197202733992, -1.452998035947227873, -62.28058590214430978 ) ) ;
#109562=CARTESIAN_POINT ( 'NONE',  ( 11.74264578624800315, -36.14014761921581709, -7.400000000000000355 ) ) ;
#109564=CARTESIAN_POINT ( 'NONE',  ( 16.43460366218431901, 17.60430054815008205, -54.39459263522238786 ) ) ;
#109603=ORIENTED_EDGE ( 'NONE', *, *, #137192, .F. ) ;
#109615=CARTESIAN_POINT ( 'NONE',  ( -25.90290776672046746, -27.60635150542758254, -16.55190051048584010 ) ) ;
#109667=CARTESIAN_POINT ( 'NONE',  ( 11.40812507854754365, 35.11059874428196537, -3.224999997268813701 ) ) ;
#109677=CARTESIAN_POINT ( 'NONE',  ( 26.94323156051284229, -28.89364864972473868, -18.52709669219397526 ) ) ;
#109714=CARTESIAN_POINT ( 'NONE',  ( -0.5319302666793322976, -21.39352396646987842, -58.79417398750189960 ) ) ;
#109723=CARTESIAN_POINT ( 'NONE',  ( -15.59328001550075271, -17.53262387181210968, -54.89123680731869115 ) ) ;
#109791=ORIENTED_EDGE ( 'NONE', *, *, #78302, .F. ) ;
#109809=AXIS2_PLACEMENT_3D ( 'NONE', #49611, #99080, #97082 ) ;
#109866=CARTESIAN_POINT ( 'NONE',  ( 2.973862142520690366, -93.04182470242774627, -23.00000000000000000 ) ) ;
#109887=CARTESIAN_POINT ( 'NONE',  ( -1.464953661133971963, -14.82524568295235134, -59.95866808466630005 ) ) ;
#109900=ORIENTED_EDGE ( 'NONE', *, *, #157130, .T. ) ;
#109902=ORIENTED_EDGE ( 'NONE', *, *, #135559, .F. ) ;
#109908=CARTESIAN_POINT ( 'NONE',  ( -22.81625015709509441, -31.40387420917324590, -6.824999997268814234 ) ) ;
#109922=CARTESIAN_POINT ( 'NONE',  ( 4.978841623633263325, 6.824288631998587817, -62.04929096494494445 ) ) ;
#109943=AXIS2_PLACEMENT_3D ( 'NONE', #102535, #26708, #54032 ) ;
#109961=CARTESIAN_POINT ( 'NONE',  ( -29.86685920354755552, 21.69954338932564397, -7.324999997268814234 ) ) ;
#109984=ORIENTED_EDGE ( 'NONE', *, *, #188361, .F. ) ;
#110024=ADVANCED_FACE ( 'NONE', ( #192338 ), #38655, .F. ) ;
#110048=CARTESIAN_POINT ( 'NONE',  ( -9.248023074035629065, -10.74802307403544077, -64.92279855667830191 ) ) ;
#110114=CARTESIAN_POINT ( 'NONE',  ( 0.2641003901806721066, 28.91815444374861599, -49.65132406768935880 ) ) ;
#110116=CARTESIAN_POINT ( 'NONE',  ( -9.553307302758575759, -9.835630382207714462, -60.44015478763000715 ) ) ;
#110149=CARTESIAN_POINT ( 'NONE',  ( 11.74264578624799427, 36.14014761921585972, -6.349999994537625980 ) ) ;
#110158=CARTESIAN_POINT ( 'NONE',  ( 37.99999999999999289, 2.893978650043524126E-14, -7.000000000000000000 ) ) ;
#110160=CARTESIAN_POINT ( 'NONE',  ( 21.94104750614016552, -1.245073757423053484, -58.42286556281732857 ) ) ;
#110196=CARTESIAN_POINT ( 'NONE',  ( -0.3431728551240714742, -71.74905178543389184, -15.00000000000000178 ) ) ;
#110248=ADVANCED_FACE ( 'NONE', ( #134670 ), #60776, .T. ) ;
#110265=CARTESIAN_POINT ( 'NONE',  ( -3.573655867282028392E-15, 2.428612866367529932E-14, 0.000000000000000000 ) ) ;
#110281=CARTESIAN_POINT ( 'NONE',  ( -4.925740194183259923, -6.812954659138648061, -62.05864287809313851 ) ) ;
#110358=EDGE_LOOP ( 'NONE', ( #166285, #30540, #182860, #63478 ) ) ;
#110360=CARTESIAN_POINT ( 'NONE',  ( 1.734723475976807094E-15, -15.20000000000001883, -64.92279855667830191 ) ) ;
#110396=DIRECTION ( 'NONE',  ( 1.000000000000000000, 0.000000000000000000, 0.000000000000000000 ) ) ;
#110411=ORIENTED_EDGE ( 'NONE', *, *, #130059, .T. ) ;
#110412=EDGE_CURVE ( 'NONE', #101425, #125361, #31446, .T. ) ;
#110425=ORIENTED_EDGE ( 'NONE', *, *, #97036, .F. ) ;
#110440=CARTESIAN_POINT ( 'NONE',  ( 23.76806875052803747, -29.07479876791797579, -18.77372378130564456 ) ) ;
#110465=ORIENTED_EDGE ( 'NONE', *, *, #129852, .T. ) ;
#110488=EDGE_CURVE ( 'NONE', #173655, #173153, #166000, .T. ) ;
#110504=EDGE_CURVE ( 'NONE', #148642, #145210, #196611, .T. ) ;
#110553=FACE_OUTER_BOUND ( 'NONE', #90824, .T. ) ;
#110555=CARTESIAN_POINT ( 'NONE',  ( 17.18269478283316332, -17.18269478283309226, -56.77278709839600879 ) ) ;
#110602=CARTESIAN_POINT ( 'NONE',  ( -27.18398240159013568, -26.16474475602790406, -20.45985799058115262 ) ) ;
#110611=EDGE_CURVE ( 'NONE', #116458, #91244, #107424, .T. ) ;
#110629=CARTESIAN_POINT ( 'NONE',  ( 4.023676584314517690, 4.713425861958483232, -64.51712888360830789 ) ) ;
#110632=CARTESIAN_POINT ( 'NONE',  ( -31.90000000000003411, 3.219216299777112361E-13, -64.92279855667830191 ) ) ;
#110634=CARTESIAN_POINT ( 'NONE',  ( 22.97392636501382768, -21.20633172485417006, -49.95052365407170925 ) ) ;
#110649=ORIENTED_EDGE ( 'NONE', *, *, #11729, .T. ) ;
#110653=CARTESIAN_POINT ( 'NONE',  ( -36.91746825000001309, 11.99521256947798342, -2.724999997268813701 ) ) ;
#110663=CARTESIAN_POINT ( 'NONE',  ( 18.37518290866868398, -35.61898371402006802, -22.28534798803313777 ) ) ;
#110711=CARTESIAN_POINT ( 'NONE',  ( -15.02701145101215907, -17.15609852811352809, -55.39549205246427022 ) ) ;
#110715=CARTESIAN_POINT ( 'NONE',  ( -22.81625015709510507, 31.40387420917330275, -2.924999997268813434 ) ) ;
#110737=CARTESIAN_POINT ( 'NONE',  ( 30.74264578624800137, -22.33583958711395212, -10.94999999453762562 ) ) ;
#110751=CYLINDRICAL_SURFACE ( 'NONE', #95066, 4.000000000000000888 ) ;
#110757=AXIS2_PLACEMENT_3D ( 'NONE', #58796, #168945, #181177 ) ;
#110784=VERTEX_POINT ( 'NONE', #76942 ) ;
#110796=DIRECTION ( 'NONE',  ( 0.000000000000000000, 0.000000000000000000, 1.000000000000000000 ) ) ;
#110887=CARTESIAN_POINT ( 'NONE',  ( -22.55670631985108443, -22.55670631985069008, -45.64921306006598201 ) ) ;
#110900=CARTESIAN_POINT ( 'NONE',  ( 36.91746824999999177, 2.880721459617395097E-14, -8.124999997268814056 ) ) ;
#110912=CARTESIAN_POINT ( 'NONE',  ( 3.882744257519136433, 5.184702103851150490, -62.44399821614913293 ) ) ;
#110935=CARTESIAN_POINT ( 'NONE',  ( -38.00000000000000711, 12.34694845685046438, -8.099999999999997868 ) ) ;
#110948=CARTESIAN_POINT ( 'NONE',  ( 36.91746824999999177, 2.880721459617395097E-14, -6.124999997268813168 ) ) ;
#110957=CARTESIAN_POINT ( 'NONE',  ( 18.27284445343954289, -33.31360383038287409, -25.98075878691503959 ) ) ;
#110986=EDGE_CURVE ( 'NONE', #179364, #16960, #130072, .T. ) ;
#111025=VERTEX_POINT ( 'NONE', #141602 ) ;
#111035=CIRCLE ( 'NONE', #62535, 69.99999999999997158 ) ;
#111040=LINE ( 'NONE', #61546, #49871 ) ;
#111097=PLANE ( 'NONE',  #12851 ) ;
#111126=AXIS2_PLACEMENT_3D ( 'NONE', #163540, #183446, #194879 ) ;
#111137=LINE ( 'NONE', #106409, #160192 ) ;
#111149=CARTESIAN_POINT ( 'NONE',  ( 23.66491666289346085, -1.240847218223132487, -57.22545927231449525 ) ) ;
#111187=DIRECTION ( 'NONE',  ( 0.000000000000000000, 0.000000000000000000, -1.000000000000000000 ) ) ;
#111206=AXIS2_PLACEMENT_3D ( 'NONE', #41432, #136416, #44414 ) ;
#111207=VERTEX_POINT ( 'NONE', #5062 ) ;
#111223=EDGE_CURVE ( 'NONE', #171283, #181594, #7406, .T. ) ;
#111231=VECTOR ( 'NONE', #100560, 1000.000000000000000 ) ;
#111239=CARTESIAN_POINT ( 'NONE',  ( -1.490485923554860426, -7.405410116723224689, -62.24175268741321787 ) ) ;
#111274=CARTESIAN_POINT ( 'NONE',  ( -5.944577070221434667, -6.769145669310464797, -61.91697028796055235 ) ) ;
#111304=LINE ( 'NONE', #4111, #166480 ) ;
#111353=ORIENTED_EDGE ( 'NONE', *, *, #195701, .T. ) ;
#111377=CIRCLE ( 'NONE', #130715, 16.70000000000002061 ) ;
#111385=FACE_OUTER_BOUND ( 'NONE', #173580, .T. ) ;
#111396=CARTESIAN_POINT ( 'NONE',  ( 32.09281931051394565, -20.34824190692416934, -24.99999999999997868 ) ) ;
#111407=AXIS2_PLACEMENT_3D ( 'NONE', #63905, #54463, #155908 ) ;
#111438=CARTESIAN_POINT ( 'NONE',  ( 33.60028042027824569, -17.96933036163179764, -21.71044752825890711 ) ) ;
#111442=ORIENTED_EDGE ( 'NONE', *, *, #197557, .F. ) ;
#111451=AXIS2_PLACEMENT_3D ( 'NONE', #41756, #23585, #193437 ) ;
#111459=EDGE_CURVE ( 'NONE', #94189, #16723, #162432, .T. ) ;
#111468=ORIENTED_EDGE ( 'NONE', *, *, #66112, .F. ) ;
#111525=DIRECTION ( 'NONE',  ( 1.000000000000000000, 0.000000000000000000, 0.000000000000000000 ) ) ;
#111549=CARTESIAN_POINT ( 'NONE',  ( 11.66180171105669672, 11.95556478057400795, -59.13370768023890633 ) ) ;
#111594=VECTOR ( 'NONE', #92144, 1000.000000000000000 ) ;
#111598=EDGE_CURVE ( 'NONE', #93910, #150285, #97738, .T. ) ;
#111603=ORIENTED_EDGE ( 'NONE', *, *, #55067, .F. ) ;
#111605=CARTESIAN_POINT ( 'NONE',  ( -32.19332086309597685, -20.18834286810128376, -25.14458231473970073 ) ) ;
#111635=CARTESIAN_POINT ( 'NONE',  ( 22.99604614807110536, -21.34730593735726245, -49.80954046291019921 ) ) ;
#111653=FACE_OUTER_BOUND ( 'NONE', #173098, .T. ) ;
#111663=CARTESIAN_POINT ( 'NONE',  ( 19.77856019329516002, -34.75272400652957572, -21.53639161265285651 ) ) ;
#111699=AXIS2_PLACEMENT_3D ( 'NONE', #129274, #38286, #37279 ) ;
#111711=CARTESIAN_POINT ( 'NONE',  ( -16.91829712735633606, -17.40385595850962730, -54.23877452087121753 ) ) ;
#111715=CARTESIAN_POINT ( 'NONE',  ( 29.86685920354754487, 21.69954338932564752, -3.424999997268813434 ) ) ;
#111735=FACE_OUTER_BOUND ( 'NONE', #52161, .T. ) ;
#111749=CARTESIAN_POINT ( 'NONE',  ( -3.874011537017815421, -5.374011537017721274, -64.44758591613756948 ) ) ;
#111771=DIRECTION ( 'NONE',  ( 3.613946018757868503E-15, 0.000000000000000000, -1.000000000000000000 ) ) ;
#111780=VERTEX_POINT ( 'NONE', #112257 ) ;
#111827=ORIENTED_EDGE ( 'NONE', *, *, #139759, .T. ) ;
#111837=AXIS2_PLACEMENT_3D ( 'NONE', #158554, #112061, #1891 ) ;
#111846=ORIENTED_EDGE ( 'NONE', *, *, #32592, .F. ) ;
#111858=CARTESIAN_POINT ( 'NONE',  ( -11.74264578624799782, -36.14014761921581709, -5.599999999999999645 ) ) ;
#111887=AXIS2_PLACEMENT_3D ( 'NONE', #134599, #57754, #196285 ) ;
#111891=EDGE_LOOP ( 'NONE', ( #55534, #7211, #47251, #181873, #61855, #84841, #146022, #90463, #131370, #6577, #173272, #147351, #137977, #67261 ) ) ;
#111893=EDGE_CURVE ( 'NONE', #123757, #179471, #120431, .T. ) ;
#111894=EDGE_LOOP ( 'NONE', ( #48938, #20757, #132831, #94422, #130555, #71694, #57919, #173468, #178269, #162904, #152760, #141314, #96232, #185848, #102251 ) ) ;
#111900=CARTESIAN_POINT ( 'NONE',  ( 11.40812507854754365, 35.11059874428196537, -9.724999997268813701 ) ) ;
#111949=CARTESIAN_POINT ( 'NONE',  ( -36.91746825000001309, -11.99521256947794789, -7.024999997268812635 ) ) ;
#111956=CARTESIAN_POINT ( 'NONE',  ( 14.61778469963306470, -34.91027835867544837, -28.77367925216604050 ) ) ;
#112001=ADVANCED_FACE ( 'NONE', ( #47616 ), #170949, .F. ) ;
#112061=DIRECTION ( 'NONE',  ( 0.000000000000000000, 0.000000000000000000, 1.000000000000000000 ) ) ;
#112101=DIRECTION ( 'NONE',  ( -0.000000000000000000, 0.000000000000000000, 1.000000000000000000 ) ) ;
#112116=CARTESIAN_POINT ( 'NONE',  ( -38.00000000000000711, 12.34694845685046438, -0.09999999999999989453 ) ) ;
#112119=CARTESIAN_POINT ( 'NONE',  ( -30.09553654342099449, 1.478515647795847654, -51.30846887466858419 ) ) ;
#112132=VERTEX_POINT ( 'NONE', #172951 ) ;
#112135=CARTESIAN_POINT ( 'NONE',  ( 37.99999999999999289, 2.893978650043524126E-14, -6.749999994537627224 ) ) ;
#112149=ORIENTED_EDGE ( 'NONE', *, *, #102940, .F. ) ;
#112151=B_SPLINE_CURVE_WITH_KNOTS ( 'NONE', 3,
 ( #95909, #19085, #170772, #91912, #1912, #185952, #77756, #63591, #93919, #33258, #169772, #188944, #153605, #78745 ),
 .UNSPECIFIED., .F., .F.,
 ( 4, 2, 2, 2, 2, 2, 4 ),
 ( 0.002370014825004548333, 0.002666056695728372464, 0.002962098566452196595, 0.003258140437176020726, 0.003554182307899844857, 0.004146266049347488783, 0.004738349790795131841 ),
 .UNSPECIFIED. ) ;
#112206=DIRECTION ( 'NONE',  ( 0.000000000000000000, 0.000000000000000000, 1.000000000000000000 ) ) ;
#112238=DIRECTION ( 'NONE',  ( 1.000000000000000000, 0.000000000000000000, 0.000000000000000000 ) ) ;
#112257=CARTESIAN_POINT ( 'NONE',  ( 3.735172737399431091E-16, 6.100000000000006750, -64.53213882399991519 ) ) ;
#112277=ADVANCED_FACE ( 'NONE', ( #147598 ), #101067, .F. ) ;
#112299=CARTESIAN_POINT ( 'NONE',  ( -18.00321789565186847, -35.67122027912861171, -27.04300662093954344 ) ) ;
#112381=CYLINDRICAL_SURFACE ( 'NONE', #186507, 1.500000000000001332 ) ;
#112406=CARTESIAN_POINT ( 'NONE',  ( -38.00000000000000711, 2.428612866367529932E-14, -10.00000000000000000 ) ) ;
#112429=AXIS2_PLACEMENT_3D ( 'NONE', #194471, #164138, #117619 ) ;
#112431=CARTESIAN_POINT ( 'NONE',  ( 25.53334702086191754, -27.44079366658231578, -18.45201707416872239 ) ) ;
#112457=CARTESIAN_POINT ( 'NONE',  ( 11.45643923738960446, -4.999999999999992895, -15.00000000000000000 ) ) ;
#112489=CARTESIAN_POINT ( 'NONE',  ( 3.735172737399431091E-16, 6.100000000000006750, -62.50719930893269805 ) ) ;
#112581=ORIENTED_EDGE ( 'NONE', *, *, #115218, .F. ) ;
#112592=CARTESIAN_POINT ( 'NONE',  ( -26.89045226410910061, -26.45365283846046367, -20.38637362918493423 ) ) ;
#112637=EDGE_LOOP ( 'NONE', ( #41842, #129033, #196625, #116492, #186829 ) ) ;
#112639=CARTESIAN_POINT ( 'NONE',  ( -11.40812507854755609, 35.11059874428196537, -3.024999997268813523 ) ) ;
#112649=CARTESIAN_POINT ( 'NONE',  ( 27.99776551637609856, -28.30561827218008375, -16.93438536460889310 ) ) ;
#112651=AXIS2_PLACEMENT_3D ( 'NONE', #53708, #113366, #158873 ) ;
#112697=CARTESIAN_POINT ( 'NONE',  ( -14.62203461105304036, -16.12203461105356794, -56.14925526931841659 ) ) ;
#112701=CARTESIAN_POINT ( 'NONE',  ( -11.40812507854754720, -35.11059874428192273, -10.72499999726881548 ) ) ;
#112720=CARTESIAN_POINT ( 'NONE',  ( 0.000000000000000000, 0.000000000000000000, -63.95112321872120731 ) ) ;
#112726=DIRECTION ( 'NONE',  ( -0.000000000000000000, -0.000000000000000000, 1.000000000000000000 ) ) ;
#112732=CARTESIAN_POINT ( 'NONE',  ( 0.000000000000000000, 0.000000000000000000, -62.91767397929362460 ) ) ;
#112734=FACE_OUTER_BOUND ( 'NONE', #53997, .T. ) ;
#112753=ADVANCED_FACE ( 'NONE', ( #140087 ), #14780, .F. ) ;
#112765=ORIENTED_EDGE ( 'NONE', *, *, #30682, .T. ) ;
#112813=VERTEX_POINT ( 'NONE', #61265 ) ;
#112823=VECTOR ( 'NONE', #4843, 1000.000000000000000 ) ;
#112847=CARTESIAN_POINT ( 'NONE',  ( 20.03432139805449808, 21.88112277201184952, -48.74685162679677575 ) ) ;
#112856=LINE ( 'NONE', #8691, #124208 ) ;
#112865=FACE_OUTER_BOUND ( 'NONE', #46322, .T. ) ;
#112886=CARTESIAN_POINT ( 'NONE',  ( -11.40812507854754720, -35.11059874428192273, -6.724999997268813701 ) ) ;
#112933=CARTESIAN_POINT ( 'NONE',  ( -11.40812507854755609, 35.11059874428196537, -3.524999997268813523 ) ) ;
#112969=VECTOR ( 'NONE', #132334, 1000.000000000000000 ) ;
#113100=CARTESIAN_POINT ( 'NONE',  ( -28.91687668646899922, 0.2552802045325772706, -52.63629878241253124 ) ) ;
#113104=LINE ( 'NONE', #189969, #63000 ) ;
#113106=AXIS2_PLACEMENT_3D ( 'NONE', #172208, #70768, #53593 ) ;
#113116=CARTESIAN_POINT ( 'NONE',  ( 23.48529157249599564, 32.32473071737754111, -6.449999994537626513 ) ) ;
#113130=DIRECTION ( 'NONE',  ( 1.000000000000000000, 0.000000000000000000, 0.000000000000000000 ) ) ;
#113177=CARTESIAN_POINT ( 'NONE',  ( -1.408284774589554589, -29.87692619418718820, -48.43935853184043339 ) ) ;
#113190=CARTESIAN_POINT ( 'NONE',  ( -19.77856019328939396, -34.75272400654478844, -21.53639161264155533 ) ) ;
#113205=PRODUCT ( 'Rear Air Intake Grille & Cap', 'Rear Air Intake Grille & Cap', '', ( #3776 ) ) ;
#113217=CARTESIAN_POINT ( 'NONE',  ( 0.000000000000000000, 0.000000000000000000, -65.00100000000003320 ) ) ;
#113247=CARTESIAN_POINT ( 'NONE',  ( -4.295634330582060123, -37.01983766409437493, -32.60000000000000142 ) ) ;
#113256=LINE ( 'NONE', #141616, #45170 ) ;
#113318=CYLINDRICAL_SURFACE ( 'NONE', #93484, 8.000000000000000000 ) ;
#113340=FACE_OUTER_BOUND ( 'NONE', #40366, .T. ) ;
#113366=DIRECTION ( 'NONE',  ( -0.000000000000000000, -0.000000000000000000, 1.000000000000000000 ) ) ;
#113383=CARTESIAN_POINT ( 'NONE',  ( -15.01195240492205762, 1.500078752102993240, -59.87740586969341905 ) ) ;
#113414=CARTESIAN_POINT ( 'NONE',  ( 25.73110857337021784, -27.25168951599283673, -18.43918238434275736 ) ) ;
#113441=VERTEX_POINT ( 'NONE', #35896 ) ;
#113499=CARTESIAN_POINT ( 'NONE',  ( -193.3062444957834884, -155.7167183371838064, -15.00000000000000178 ) ) ;
#113512=ADVANCED_FACE ( 'NONE', ( #176427 ), #38902, .T. ) ;
#113525=CARTESIAN_POINT ( 'NONE',  ( 9.243954752495790572, 10.58667710475866564, -60.30599866924266905 ) ) ;
#113578=CARTESIAN_POINT ( 'NONE',  ( -25.73110857336972046, -27.25168951599382794, -18.43918238433846213 ) ) ;
#113583=VECTOR ( 'NONE', #31417, 1000.000000000000000 ) ;
#113594=ORIENTED_EDGE ( 'NONE', *, *, #183262, .F. ) ;
#113596=SPHERICAL_SURFACE ( 'NONE', #108514, 8.000000000000000000 ) ;
#113601=CARTESIAN_POINT ( 'NONE',  ( -28.91886483090992144, 0.2690448904511072437, -49.65045026909250936 ) ) ;
#113604=CARTESIAN_POINT ( 'NONE',  ( 5.759383325533893760, 6.837149423127133474, -63.98874707071207268 ) ) ;
#113623=ORIENTED_EDGE ( 'NONE', *, *, #48581, .T. ) ;
#113626=CARTESIAN_POINT ( 'NONE',  ( -22.81625015709509441, -31.40387420917324590, -2.324999997268813789 ) ) ;
#113636=CARTESIAN_POINT ( 'NONE',  ( 28.30573922537810816, -27.84595035627268800, -20.14355118860781957 ) ) ;
#113643=ADVANCED_FACE ( 'NONE', ( #146060 ), #162238, .F. ) ;
#113662=FACE_OUTER_BOUND ( 'NONE', #174361, .T. ) ;
#113685=CARTESIAN_POINT ( 'NONE',  ( -36.91746825000001309, -11.99521256947794789, -9.024999997268812635 ) ) ;
#113699=VERTEX_POINT ( 'NONE', #181419 ) ;
#113721=CARTESIAN_POINT ( 'NONE',  ( 29.32058373238547588, -1.046637022530830574, -52.18867397238361150 ) ) ;
#113724=CARTESIAN_POINT ( 'NONE',  ( 0.000000000000000000, -165.0000000000000000, 12.00000000000000355 ) ) ;
#113743=CARTESIAN_POINT ( 'NONE',  ( -21.49604614807110536, 21.49604614807103786, -65.00100000000003320 ) ) ;
#113804=DIRECTION ( 'NONE',  ( 1.000000000000000000, 0.000000000000000000, 0.000000000000000000 ) ) ;
#113837=FACE_OUTER_BOUND ( 'NONE', #14286, .T. ) ;
#113846=CARTESIAN_POINT ( 'NONE',  ( -27.98120534312124974, -28.16303873514637957, -20.10652275068721195 ) ) ;
#113858=CARTESIAN_POINT ( 'NONE',  ( -22.81625015709509441, -31.40387420917324590, -2.324999997268813345 ) ) ;
#113867=CARTESIAN_POINT ( 'NONE',  ( -32.09281931051391012, -20.34824190692417289, -24.99999999999999289 ) ) ;
#113918=CARTESIAN_POINT ( 'NONE',  ( 29.86685920354754487, 21.69954338932564752, -3.924999997268812990 ) ) ;
#113919=CARTESIAN_POINT ( 'NONE',  ( -20.43538597629128262, 20.43538597629122222, -52.65483682830182488 ) ) ;
#113929=CARTESIAN_POINT ( 'NONE',  ( 17.01743274722963051, 17.33027132694079242, -56.78176416808769034 ) ) ;
#113941=ORIENTED_EDGE ( 'NONE', *, *, #181196, .T. ) ;
#113957=ADVANCED_FACE ( 'NONE', ( #40900 ), #196595, .T. ) ;
#113988=ORIENTED_EDGE ( 'NONE', *, *, #161100, .F. ) ;
#114003=CARTESIAN_POINT ( 'NONE',  ( 0.000000000000000000, -105.0000000000000000, 12.00000000000000355 ) ) ;
#114007=CARTESIAN_POINT ( 'NONE',  ( -11.29706596393373985, -12.15234863546621646, -59.18655785247093348 ) ) ;
#114046=DIRECTION ( 'NONE',  ( -0.000000000000000000, -0.000000000000000000, -1.000000000000000000 ) ) ;
#114048=ORIENTED_EDGE ( 'NONE', *, *, #75628, .F. ) ;
#114071=CARTESIAN_POINT ( 'NONE',  ( 11.30153831258470731, -190.0000000000000000, -15.00000000000000178 ) ) ;
#114087=DIRECTION ( 'NONE',  ( 0.8571673007021135549, 0.000000000000000000, 0.5150380749100520461 ) ) ;
#114100=EDGE_LOOP ( 'NONE', ( #106627, #117828, #159806 ) ) ;
#114105=CARTESIAN_POINT ( 'NONE',  ( 3.766062262543149401E-15, -39.95556452105413570, -3.249999994537627224 ) ) ;
#114120=CARTESIAN_POINT ( 'NONE',  ( 20.53360937444653445, -31.96911244174550149, -23.96531494639225812 ) ) ;
#114164=DIRECTION ( 'NONE',  ( 1.000000000000000000, 0.000000000000000000, 0.000000000000000000 ) ) ;
#114176=CARTESIAN_POINT ( 'NONE',  ( -5.136056113502131204, -40.38396894447051721, -25.53196577691469926 ) ) ;
#114177=EDGE_LOOP ( 'NONE', ( #172361, #74196, #14923, #193552 ) ) ;
#114254=VECTOR ( 'NONE', #154178, 1000.000000000000000 ) ;
#114314=CARTESIAN_POINT ( 'NONE',  ( -38.00000000000000711, 2.428612866367529932E-14, -5.999999999999999112 ) ) ;
#114335=CARTESIAN_POINT ( 'NONE',  ( 17.36633513277089236, -35.95409897417799527, -27.53902325179317856 ) ) ;
#114352=ORIENTED_EDGE ( 'NONE', *, *, #70168, .T. ) ;
#114412=CARTESIAN_POINT ( 'NONE',  ( 31.84446081652115978, -20.74826690461661372, -24.63985244029811739 ) ) ;
#114479=DIRECTION ( 'NONE',  ( 0.8660254037844391517, -0.000000000000000000, -0.4999999999999991673 ) ) ;
#114483=AXIS2_PLACEMENT_3D ( 'NONE', #15264, #103304, #43620 ) ;
#114491=CARTESIAN_POINT ( 'NONE',  ( -6.856101608890801443E-16, -67.16067257189654072, -22.99988689144064580 ) ) ;
#114516=DIRECTION ( 'NONE',  ( -0.000000000000000000, -0.000000000000000000, -1.000000000000000000 ) ) ;
#114532=CIRCLE ( 'NONE', #11244, 37.23224409030433435 ) ;
#114595=DIRECTION ( 'NONE',  ( -0.000000000000000000, -0.000000000000000000, -1.000000000000000000 ) ) ;
#114600=CARTESIAN_POINT ( 'NONE',  ( -11.30153831258471975, -180.0000000000000000, -15.00000000000000178 ) ) ;
#114605=CARTESIAN_POINT ( 'NONE',  ( -31.88110949919180470, 0.2682394567897747883, -45.67705988491092484 ) ) ;
#114618=AXIS2_PLACEMENT_3D ( 'NONE', #118598, #145908, #101399 ) ;
#114627=UNCERTAINTY_MEASURE_WITH_UNIT (LENGTH_MEASURE( 1.000000000000000082E-05 ), #101239, 'distance_accuracy_value', 'NONE');
#114628=VERTEX_POINT ( 'NONE', #77186 ) ;
#114631=CARTESIAN_POINT ( 'NONE',  ( 38.00000000000000000, 12.34694845685046616, -0.9000000000000000222 ) ) ;
#114642=CARTESIAN_POINT ( 'NONE',  ( 32.63354670693964721, -22.83594557638339850, -20.39123836177202520 ) ) ;
#114684=CYLINDRICAL_SURFACE ( 'NONE', #102375, 1.500000000000001332 ) ;
#114692=ORIENTED_EDGE ( 'NONE', *, *, #24537, .T. ) ;
#114698=CARTESIAN_POINT ( 'NONE',  ( -36.91746825000001309, -11.99521256947794789, -2.524999997268813523 ) ) ;
#114734=CARTESIAN_POINT ( 'NONE',  ( 11.95117975717237080, -11.66618673445833920, -61.34707691135563579 ) ) ;
#114764=VERTEX_POINT ( 'NONE', #142823 ) ;
#114778=AXIS2_PLACEMENT_3D ( 'NONE', #5635, #6631, #113804 ) ;
#114807=ADVANCED_FACE ( 'NONE', ( #158985 ), #4303, .F. ) ;
#114815=ORIENTED_EDGE ( 'NONE', *, *, #53785, .T. ) ;
#114872=CARTESIAN_POINT ( 'NONE',  ( -29.86685920354755197, -21.69954338932560134, -4.424999997268812990 ) ) ;
#114947=CARTESIAN_POINT ( 'NONE',  ( 14.67883866103747970, 15.69994562750269473, -58.73507448357032246 ) ) ;
#115007=ORIENTED_EDGE ( 'NONE', *, *, #182492, .T. ) ;
#115027=CARTESIAN_POINT ( 'NONE',  ( 3.766062262543149401E-15, -39.95556452105413570, -11.24999999453762456 ) ) ;
#115083=CARTESIAN_POINT ( 'NONE',  ( -4.347827484049745728, -37.01609572856843045, -32.59999999897104317 ) ) ;
#115123=CARTESIAN_POINT ( 'NONE',  ( -38.00000000000001421, -12.34694845685042708, -7.649999994537626691 ) ) ;
#115131=CARTESIAN_POINT ( 'NONE',  ( 0.000000000000000000, 0.000000000000000000, -54.21489346206828230 ) ) ;
#115137=LINE ( 'NONE', #189012, #15305 ) ;
#115156=CIRCLE ( 'NONE', #179717, 8.000000000000000000 ) ;
#115183=CARTESIAN_POINT ( 'NONE',  ( -11.45643923738960446, -4.999999999999992895, -18.00000000000000000 ) ) ;
#115196=CARTESIAN_POINT ( 'NONE',  ( -8.400629636141269785, -38.44252190851295836, -32.19688134020307047 ) ) ;
#115208=CARTESIAN_POINT ( 'NONE',  ( 9.252314257645119611, 10.97407593764238598, -62.33638803020407693 ) ) ;
#115218=EDGE_CURVE ( 'NONE', #69935, #168486, #130215, .T. ) ;
#115279=EDGE_CURVE ( 'NONE', #170287, #150779, #115499, .T. ) ;
#115324=AXIS2_PLACEMENT_3D ( 'NONE', #166599, #43244, #149425 ) ;
#115333=FACE_OUTER_BOUND ( 'NONE', #174300, .T. ) ;
#115354=ORIENTED_EDGE ( 'NONE', *, *, #102120, .T. ) ;
#115357=CARTESIAN_POINT ( 'NONE',  ( 8.231229499107000080, -38.47007264976928553, -32.24440875978786636 ) ) ;
#115376=VERTEX_POINT ( 'NONE', #83142 ) ;
#115433=CARTESIAN_POINT ( 'NONE',  ( 31.20004872165405985, -21.37828431676117802, -20.08970689225314032 ) ) ;
#115437=ORIENTED_EDGE ( 'NONE', *, *, #134940, .F. ) ;
#115449=AXIS2_PLACEMENT_3D ( 'NONE', #84840, #112206, #116198 ) ;
#115458=EDGE_CURVE ( 'NONE', #52978, #55466, #158006, .T. ) ;
#115499=LINE ( 'NONE', #177186, #101219 ) ;
#115501=CARTESIAN_POINT ( 'NONE',  ( 0.2000162670639714646, 6.100000000000010303, -64.53213882399991519 ) ) ;
#115504=CYLINDRICAL_SURFACE ( 'NONE', #167811, 38.00000000000000000 ) ;
#115553=ADVANCED_FACE ( 'NONE', ( #49835 ), #36635, .T. ) ;
#115591=ORIENTED_EDGE ( 'NONE', *, *, #44038, .F. ) ;
#115592=CARTESIAN_POINT ( 'NONE',  ( 37.99999999999999289, 2.428612866367529932E-14, -18.00000000000000000 ) ) ;
#115620=CIRCLE ( 'NONE', #5764, 10.00000000000000000 ) ;
#115644=VERTEX_POINT ( 'NONE', #112489 ) ;
#115647=CARTESIAN_POINT ( 'NONE',  ( -29.86685920354755197, -21.69954338932560134, -8.424999997268812990 ) ) ;
#115666=EDGE_CURVE ( 'NONE', #120193, #182543, #146824, .T. ) ;
#115671=ORIENTED_EDGE ( 'NONE', *, *, #72464, .T. ) ;
#115703=EDGE_CURVE ( 'NONE', #99310, #100403, #148839, .T. ) ;
#115704=VERTEX_POINT ( 'NONE', #58801 ) ;
#115709=CARTESIAN_POINT ( 'NONE',  ( 36.91746824999999887, 11.99521256947799053, -9.524999997268812635 ) ) ;
#115745=DIRECTION ( 'NONE',  ( 0.000000000000000000, 0.000000000000000000, 1.000000000000000000 ) ) ;
#115748=CARTESIAN_POINT ( 'NONE',  ( 0.000000000000000000, 0.000000000000000000, -64.92279855667830191 ) ) ;
#115825=EDGE_CURVE ( 'NONE', #34604, #69503, #119501, .T. ) ;
#115833=EDGE_CURVE ( 'NONE', #41082, #42510, #62396, .T. ) ;
#115842=EDGE_LOOP ( 'NONE', ( #97573, #44722, #55523, #21766, #73700 ) ) ;
#115860=PLANE ( 'NONE',  #85310 ) ;
#115889=CARTESIAN_POINT ( 'NONE',  ( -31.67087737765754341, -20.99984420384768313, -23.45156215417600265 ) ) ;
#115914=ORIENTED_EDGE ( 'NONE', *, *, #147079, .T. ) ;
#115927=FACE_OUTER_BOUND ( 'NONE', #131754, .T. ) ;
#115938=CARTESIAN_POINT ( 'NONE',  ( -16.70000000000002061, 1.759457951533292443E-13, -64.92279855667830191 ) ) ;
#115942=B_SPLINE_CURVE_WITH_KNOTS ( 'NONE', 3,
 ( #133026, #194716, #56186, #117869, #44014, #119859, #165378, #25876 ),
 .UNSPECIFIED., .F., .F.,
 ( 4, 2, 2, 4 ),
 ( 2.784207231387392883E-07, 0.0003066998903876386857, 0.0006131213600521387115, 0.001225964299381153508 ),
 .UNSPECIFIED. ) ;
#115957=ORIENTED_EDGE ( 'NONE', *, *, #55329, .T. ) ;
#116024=DIRECTION ( 'NONE',  ( -0.000000000000000000, -0.000000000000000000, 1.000000000000000000 ) ) ;
#116087=CARTESIAN_POINT ( 'NONE',  ( 11.48731001631952253, -9.434891085173717329, -62.13554135533229328 ) ) ;
#116105=LINE ( 'NONE', #129257, #199362 ) ;
#116121=FACE_OUTER_BOUND ( 'NONE', #150689, .T. ) ;
#116124=CARTESIAN_POINT ( 'NONE',  ( 30.74264578624800137, -22.33583958711395212, -8.949999994537627401 ) ) ;
#116137=CYLINDRICAL_SURFACE ( 'NONE', #70315, 5.000000000000000000 ) ;
#116153=DIRECTION ( 'NONE',  ( -0.000000000000000000, -0.000000000000000000, 1.000000000000000000 ) ) ;
#116156=TOROIDAL_SURFACE ( 'NONE', #12984, 48.98979485566358250, 12.00000000000000000 ) ;
#116163=DIRECTION ( 'NONE',  ( 0.9930308165857338887, 0.1178549842436489581, 0.000000000000000000 ) ) ;
#116174=CARTESIAN_POINT ( 'NONE',  ( 22.81625015709510151, -31.40387420917324590, -2.424999997268812990 ) ) ;
#116175=CARTESIAN_POINT ( 'NONE',  ( -1.337618122189682346, -23.50300173439381624, -57.33987540012262230 ) ) ;
#116184=DIRECTION ( 'NONE',  ( -0.000000000000000000, -0.000000000000000000, 1.000000000000000000 ) ) ;
#116198=DIRECTION ( 'NONE',  ( 1.000000000000000000, 0.000000000000000000, 0.000000000000000000 ) ) ;
#116199=ORIENTED_EDGE ( 'NONE', *, *, #19937, .T. ) ;
#116208=CARTESIAN_POINT ( 'NONE',  ( 9.391041506135660910, 10.10090423873401733, -62.54717694538948791 ) ) ;
#116306=FACE_OUTER_BOUND ( 'NONE', #156346, .T. ) ;
#116324=DIRECTION ( 'NONE',  ( 1.000000000000000000, 0.000000000000000000, 0.000000000000000000 ) ) ;
#116327=CARTESIAN_POINT ( 'NONE',  ( -25.65937876999938894, -27.64914803190709591, -20.38451907593472612 ) ) ;
#116347=CARTESIAN_POINT ( 'NONE',  ( 19.82991159619255228, -34.74521775907860643, -25.51696690232491349 ) ) ;
#116365=EDGE_LOOP ( 'NONE', ( #192619, #8791, #132006, #10180 ) ) ;
#116374=CARTESIAN_POINT ( 'NONE',  ( 6.874011537017776341, -5.374011537017756801, -64.03675147074802965 ) ) ;
#116378=CARTESIAN_POINT ( 'NONE',  ( -10.27157327577100254, -12.17763598328338936, -59.49962702345104049 ) ) ;
#116384=CARTESIAN_POINT ( 'NONE',  ( 11.74264578624800315, -36.14014761921581709, -5.149999994537626691 ) ) ;
#116412=EDGE_LOOP ( 'NONE', ( #120884, #72621, #71140, #172517 ) ) ;
#116420=EDGE_CURVE ( 'NONE', #193461, #71928, #55924, .T. ) ;
#116432=EDGE_LOOP ( 'NONE', ( #187058, #192341, #165913, #160701, #53204, #116627, #3411, #128737, #58981, #87334 ) ) ;
#116458=VERTEX_POINT ( 'NONE', #70996 ) ;
#116492=ORIENTED_EDGE ( 'NONE', *, *, #121295, .F. ) ;
#116495=CARTESIAN_POINT ( 'NONE',  ( 1.424896265312427746, 7.121249343341831128, -64.33531891713909090 ) ) ;
#116496=EDGE_CURVE ( 'NONE', #19675, #141549, #134674, .T. ) ;
#116594=CARTESIAN_POINT ( 'NONE',  ( -4.647474457565486646E-15, 28.90000000000004476, -52.65483682830183199 ) ) ;
#116612=CARTESIAN_POINT ( 'NONE',  ( 0.000000000000000000, 0.000000000000000000, -64.53213882399991519 ) ) ;
#116620=CARTESIAN_POINT ( 'NONE',  ( 6.293193206003583562, 6.576150211591589745, -63.95112321872120731 ) ) ;
#116625=CARTESIAN_POINT ( 'NONE',  ( 31.05781409862806797, -25.21364184384349727, -18.17652835081984009 ) ) ;
#116627=ORIENTED_EDGE ( 'NONE', *, *, #36648, .F. ) ;
#116641=CARTESIAN_POINT ( 'NONE',  ( -23.48529157249600985, 32.32473071737754111, -0.2999999999999999334 ) ) ;
#116662=ORIENTED_EDGE ( 'NONE', *, *, #200059, .F. ) ;
#116665=FACE_BOUND ( 'NONE', #154639, .T. ) ;
#116672=EDGE_CURVE ( 'NONE', #86619, #124248, #138614, .T. ) ;
#116695=VERTEX_POINT ( 'NONE', #29475 ) ;
#116699=CARTESIAN_POINT ( 'NONE',  ( -36.91746825000001309, -11.99521256947794789, -6.524999997268810858 ) ) ;
#116714=VERTEX_POINT ( 'NONE', #43645 ) ;
#116867=ORIENTED_EDGE ( 'NONE', *, *, #62255, .F. ) ;
#116871=CARTESIAN_POINT ( 'NONE',  ( -36.91746825000000598, 11.99521256947798520, -4.724999997268811924 ) ) ;
#117002=VERTEX_POINT ( 'NONE', #97 ) ;
#117057=CARTESIAN_POINT ( 'NONE',  ( -17.31327599691207197, 15.19344129729072712, -55.22348155082431020 ) ) ;
#117119=CARTESIAN_POINT ( 'NONE',  ( -30.74264578624800492, 22.33583958711400186, -7.949999994537626513 ) ) ;
#117126=CARTESIAN_POINT ( 'NONE',  ( 4.944490673674106773, -3.929198865016385156, -62.47179825203327397 ) ) ;
#117132=CARTESIAN_POINT ( 'NONE',  ( -11.16651649332244212, 9.304348965730380172, -60.11051939825532031 ) ) ;
#117136=EDGE_LOOP ( 'NONE', ( #76331, #192859, #167739, #28068 ) ) ;
#117171=CARTESIAN_POINT ( 'NONE',  ( 36.91746824999999887, -11.99521256947793546, -4.224999997268813701 ) ) ;
#117181=CARTESIAN_POINT ( 'NONE',  ( -40.00000000000000711, 2.918471586026471156E-14, 0.000000000000000000 ) ) ;
#117184=B_SPLINE_CURVE_WITH_KNOTS ( 'NONE', 3,
 ( #46596, #157756, #108256, #155754, #109249, #154764, #33415, #65727, #31427, #78905, #19247, #173928, #34409, #35397, #125425, #18256, #81868, #93080, #48593, #140582, #3068, #95074 ),
 .UNSPECIFIED., .F., .F.,
 ( 4, 2, 2, 2, 2, 2, 2, 2, 2, 2, 4 ),
 ( 1.970604705270169680E-07, 0.0003054521314110711003, 0.0006107072023516151114, 0.001221217344232706928, 0.001831727486113798962, 0.002136982557054344870, 0.002442237627994890779, 0.003052747769875995172, 0.003663257911757099566, 0.004273768053638204827, 0.004884278195519306184 ),
 .UNSPECIFIED. ) ;
#117195=CARTESIAN_POINT ( 'NONE',  ( -24.80109738229592509, -30.87060611836150059, -19.02242571537068017 ) ) ;
#117211=CARTESIAN_POINT ( 'NONE',  ( 21.36119649488921013, -0.4379334789936405459, -56.42482690868973094 ) ) ;
#117223=CARTESIAN_POINT ( 'NONE',  ( 0.000000000000000000, 0.000000000000000000, -65.00100000000003320 ) ) ;
#117230=CIRCLE ( 'NONE', #62360, 9.100000000000001421 ) ;
#117232=CARTESIAN_POINT ( 'NONE',  ( -0.3968392070109439951, -6.139906835403845520, -62.49911542708239409 ) ) ;
#117324=CARTESIAN_POINT ( 'NONE',  ( -16.92372544712134541, -17.40010620954080522, -56.79388978676514910 ) ) ;
#117327=CARTESIAN_POINT ( 'NONE',  ( -27.48145228890726699, -25.86941904439673223, -20.55877432051689624 ) ) ;
#117405=VECTOR ( 'NONE', #197338, 1000.000000000000000 ) ;
#117432=VERTEX_POINT ( 'NONE', #31449 ) ;
#117455=EDGE_LOOP ( 'NONE', ( #24467, #166152, #161623, #109603 ) ) ;
#117464=CIRCLE ( 'NONE', #188477, 38.00000000000000000 ) ;
#117491=EDGE_LOOP ( 'NONE', ( #167510, #159675, #168298, #135754, #128823 ) ) ;
#117497=LINE ( 'NONE', #52812, #135502 ) ;
#117619=DIRECTION ( 'NONE',  ( -1.000000000000000000, 0.000000000000000000, 0.000000000000000000 ) ) ;
#117645=CARTESIAN_POINT ( 'NONE',  ( -29.86685920354755552, 21.69954338932564397, -6.824999997268814234 ) ) ;
#117654=CARTESIAN_POINT ( 'NONE',  ( 27.83073679762881980, -28.30972371524019948, -20.09501658340476737 ) ) ;
#117668=ORIENTED_EDGE ( 'NONE', *, *, #143629, .F. ) ;
#117704=CARTESIAN_POINT ( 'NONE',  ( -11.40812507854754720, -35.11059874428192273, -8.224999997268813701 ) ) ;
#117741=CARTESIAN_POINT ( 'NONE',  ( 5.000000000000000000, 0.000000000000000000, -18.00000000000000000 ) ) ;
#117745=DIRECTION ( 'NONE',  ( 1.000000000000000000, 0.000000000000000000, 0.000000000000000000 ) ) ;
#117749=EDGE_CURVE ( 'NONE', #181556, #42534, #12955, .T. ) ;
#117777=VERTEX_POINT ( 'NONE', #99070 ) ;
#117828=ORIENTED_EDGE ( 'NONE', *, *, #127970, .T. ) ;
#117840=EDGE_CURVE ( 'NONE', #19028, #89236, #129079, .T. ) ;
#117859=CARTESIAN_POINT ( 'NONE',  ( -6.017829804060265353, -47.35862344248571532, -22.79591852006818087 ) ) ;
#117869=CARTESIAN_POINT ( 'NONE',  ( -14.81258577508671515, -15.38338031094985325, -56.43166240502930719 ) ) ;
#117884=CARTESIAN_POINT ( 'NONE',  ( -36.91746825000000598, 2.428612866367529932E-14, -10.62499999726881406 ) ) ;
#117886=VECTOR ( 'NONE', #37027, 1000.000000000000000 ) ;
#117929=AXIS2_PLACEMENT_3D ( 'NONE', #106930, #140249, #185780 ) ;
#117944=LINE ( 'NONE', #115938, #144746 ) ;
#117961=VERTEX_POINT ( 'NONE', #175941 ) ;
#118027=VECTOR ( 'NONE', #57489, 1000.000000000000000 ) ;
#118034=FACE_OUTER_BOUND ( 'NONE', #121551, .T. ) ;
#118042=VECTOR ( 'NONE', #157176, 1000.000000000000000 ) ;
#118095=CARTESIAN_POINT ( 'NONE',  ( 11.09110223580025689, -9.259486913381270057, -62.30073625427280604 ) ) ;
#118097=CARTESIAN_POINT ( 'NONE',  ( -0.2045547421925955622, -16.68945015508927199, -61.35148950497489295 ) ) ;
#118115=CIRCLE ( 'NONE', #114778, 16.70000000000002061 ) ;
#118119=CARTESIAN_POINT ( 'NONE',  ( 12.22610943951276319, -10.45445179612737086, -59.42747105264538732 ) ) ;
#118127=VERTEX_POINT ( 'NONE', #108945 ) ;
#118130=CARTESIAN_POINT ( 'NONE',  ( -17.18269478283327345, -17.18269478283298568, -54.21489346206828230 ) ) ;
#118134=CARTESIAN_POINT ( 'NONE',  ( 30.74264578624800137, -22.33583958711395212, -4.949999994537626513 ) ) ;
#118145=CARTESIAN_POINT ( 'NONE',  ( -10.10305183197212742, 9.389996629557172625, -60.40856999928715254 ) ) ;
#118149=ORIENTED_EDGE ( 'NONE', *, *, #150015, .T. ) ;
#118183=CARTESIAN_POINT ( 'NONE',  ( -22.81625015709509441, -31.40387420917324590, -6.824999997268814234 ) ) ;
#118184=CYLINDRICAL_SURFACE ( 'NONE', #79704, 214.0437394197456342 ) ;
#118207=CARTESIAN_POINT ( 'NONE',  ( -27.53771902582940001, -28.32105632907237691, -18.50180672658962777 ) ) ;
#118208=ORIENTED_EDGE ( 'NONE', *, *, #130640, .F. ) ;
#118222=DIRECTION ( 'NONE',  ( -0.000000000000000000, -0.000000000000000000, 1.000000000000000000 ) ) ;
#118235=CARTESIAN_POINT ( 'NONE',  ( 6.404328268737250696, -0.9271017399331602515, -64.47359807031668311 ) ) ;
#118340=CARTESIAN_POINT ( 'NONE',  ( 1.370007243092780325, 31.03250612061568248, -46.89016925620975229 ) ) ;
#118359=EDGE_LOOP ( 'NONE', ( #48758, #167613 ) ) ;
#118362=CARTESIAN_POINT ( 'NONE',  ( 0.000000000000000000, 0.000000000000000000, -64.92279855667830191 ) ) ;
#118386=CARTESIAN_POINT ( 'NONE',  ( 20.33413869251837980, 22.45862007004985728, -51.11888769873470295 ) ) ;
#118403=CARTESIAN_POINT ( 'NONE',  ( 31.90000000000003411, 0.000000000000000000, -49.13275782002545355 ) ) ;
#118408=CARTESIAN_POINT ( 'NONE',  ( 18.36170132746700645, -35.61590944478783172, -18.35554273634629752 ) ) ;
#118414=ORIENTED_EDGE ( 'NONE', *, *, #48810, .F. ) ;
#118443=( BOUNDED_CURVE ( )  B_SPLINE_CURVE ( 2, ( #85269, #146960, #128773, #71122, #193472, #190472, #38788, #147970, #21613, #51945, #84265 ),
 .UNSPECIFIED., .F., .T. ) 
 B_SPLINE_CURVE_WITH_KNOTS ( ( 3, 2, 2, 2, 2, 3 ),
 ( 0.5000000000000001110, 0.5200000000000001288, 0.5400000000000001465, 0.5600000000000001643, 0.5800000000000000711, 0.6000000000000000888 ),
 .UNSPECIFIED. ) 
 CURVE ( )  GEOMETRIC_REPRESENTATION_ITEM ( )  RATIONAL_B_SPLINE_CURVE ( ( 0.9999999999999997780, 0.9510565162951537532, 1.000000000000000000, 0.9510565162951535312, 1.000000000000000000, 0.9510565162951535312, 1.000000000000000000, 0.9510565162951535312, 1.000000000000000000, 0.9510565162951533091, 1.000000000000000222 ) ) 
 REPRESENTATION_ITEM ( '' )  );
#118469=ORIENTED_EDGE ( 'NONE', *, *, #54562, .F. ) ;
#118505=DIRECTION ( 'NONE',  ( 1.000000000000000000, 0.000000000000000000, 0.000000000000000000 ) ) ;
#118527=LINE ( 'NONE', #41686, #163021 ) ;
#118537=CARTESIAN_POINT ( 'NONE',  ( -11.30153831258470731, -188.0000000000000000, 0.000000000000000000 ) ) ;
#118598=CARTESIAN_POINT ( 'NONE',  ( 0.000000000000000000, 0.000000000000000000, -18.00000000000000000 ) ) ;
#118619=CARTESIAN_POINT ( 'NONE',  ( -69.65682714487590488, -71.74905178543390605, -15.00000000000000178 ) ) ;
#118621=ORIENTED_EDGE ( 'NONE', *, *, #58626, .F. ) ;
#118637=CARTESIAN_POINT ( 'NONE',  ( -3.573655867282028392E-15, 2.428612866367529932E-14, 0.000000000000000000 ) ) ;
#118652=CARTESIAN_POINT ( 'NONE',  ( 29.86685920354754842, -21.69954338932559068, -9.824999997268813345 ) ) ;
#118682=ORIENTED_EDGE ( 'NONE', *, *, #177665, .T. ) ;
#118712=CARTESIAN_POINT ( 'NONE',  ( 22.81625015709509441, 31.40387420917330275, -9.324999997268813345 ) ) ;
#118793=CARTESIAN_POINT ( 'NONE',  ( -19.99999999999998224, -180.0000000000000000, -15.00000000000000178 ) ) ;
#118802=AXIS2_PLACEMENT_3D ( 'NONE', #178882, #11022, #130331 ) ;
#118830=VECTOR ( 'NONE', #46268, 1000.000000000000000 ) ;
#118839=ORIENTED_EDGE ( 'NONE', *, *, #145712, .F. ) ;
#118877=DIRECTION ( 'NONE',  ( 0.000000000000000000, 0.000000000000000000, 1.000000000000000000 ) ) ;
#118891=CARTESIAN_POINT ( 'NONE',  ( 29.86685920354754842, -21.69954338932559068, -9.824999997268813345 ) ) ;
#118898=EDGE_LOOP ( 'NONE', ( #86612, #150986, #182251, #130855, #9476 ) ) ;
#118949=DIRECTION ( 'NONE',  ( 1.000000000000000000, 0.000000000000000000, 0.000000000000000000 ) ) ;
#119028=FILL_AREA_STYLE_COLOUR ( '', #137220 ) ;
#119036=EDGE_CURVE ( 'NONE', #156928, #150928, #148611, .T. ) ;
#119099=CARTESIAN_POINT ( 'NONE',  ( 12.08042635477516846, -10.04444949571651158, -61.78581196890001337 ) ) ;
#119136=CARTESIAN_POINT ( 'NONE',  ( -38.00000000000001421, 12.34694845685046438, -5.849999994537627757 ) ) ;
#119142=CARTESIAN_POINT ( 'NONE',  ( 4.539240849104785980, -4.118817879080736155, -62.50270742379689182 ) ) ;
#119148=CARTESIAN_POINT ( 'NONE',  ( -11.25730316407969234, 9.333912919581832668, -60.07366171483953110 ) ) ;
#119183=CARTESIAN_POINT ( 'NONE',  ( 29.86685920354754487, 21.69954338932564752, -1.924999997268813212 ) ) ;
#119199=ORIENTED_EDGE ( 'NONE', *, *, #981, .F. ) ;
#119205=CARTESIAN_POINT ( 'NONE',  ( -25.17999522921142841, -30.53243704067310560, -18.89073929087953374 ) ) ;
#119219=CARTESIAN_POINT ( 'NONE',  ( 22.62812085840269560, -1.500606516337551044, -55.49205433527804843 ) ) ;
#119223=EDGE_CURVE ( 'NONE', #87857, #69935, #38772, .T. ) ;
#119233=DIRECTION ( 'NONE',  ( -0.000000000000000000, -0.000000000000000000, 1.000000000000000000 ) ) ;
#119338=CARTESIAN_POINT ( 'NONE',  ( -1.221313414957698099E-14, 31.90000000000003411, -45.64921306006598201 ) ) ;
#119342=LINE ( 'NONE', #123280, #183443 ) ;
#119352=VERTEX_POINT ( 'NONE', #160371 ) ;
#119367=CIRCLE ( 'NONE', #70861, 38.00000000000000000 ) ;
#119385=CARTESIAN_POINT ( 'NONE',  ( 21.53952979013940094, 22.99870628207707668, -49.63989001790915978 ) ) ;
#119387=DIRECTION ( 'NONE',  ( 1.000000000000000000, 0.000000000000000000, 0.000000000000000000 ) ) ;
#119406=CARTESIAN_POINT ( 'NONE',  ( -6.328346318964374717, -6.540997098630797701, -63.95112321872120731 ) ) ;
#119411=ORIENTED_EDGE ( 'NONE', *, *, #150161, .T. ) ;
#119429=CARTESIAN_POINT ( 'NONE',  ( -6.565813341170984252, 4.458020396767564009, -64.20492216656604967 ) ) ;
#119454=EDGE_CURVE ( 'NONE', #1233, #171664, #10577, .T. ) ;
#119463=CARTESIAN_POINT ( 'NONE',  ( 5.000000000000003553, -4.999999999999996447, -15.00000000000000000 ) ) ;
#119464=VERTEX_POINT ( 'NONE', #99687 ) ;
#119482=EDGE_CURVE ( 'NONE', #48307, #127799, #191702, .T. ) ;
#119501=LINE ( 'NONE', #89147, #30224 ) ;
#119586=ORIENTED_EDGE ( 'NONE', *, *, #140816, .F. ) ;
#119592=LINE ( 'NONE', #60870, #156644 ) ;
#119618=DIRECTION ( 'NONE',  ( -0.000000000000000000, -0.000000000000000000, 1.000000000000000000 ) ) ;
#119626=CARTESIAN_POINT ( 'NONE',  ( 5.000000000000003553, -4.999999999999996447, -18.00000000000000000 ) ) ;
#119631=DIRECTION ( 'NONE',  ( 1.000000000000000000, 0.000000000000000000, 0.000000000000000000 ) ) ;
#119633=CARTESIAN_POINT ( 'NONE',  ( 4.000000000000000888, -165.0000000000000000, -23.00000000000000000 ) ) ;
#119639=CARTESIAN_POINT ( 'NONE',  ( -19.99999999999998224, -180.0000000000000000, -15.00000000000000178 ) ) ;
#119641=AXIS2_PLACEMENT_3D ( 'NONE', #25777, #54092, #134944 ) ;
#119648=CARTESIAN_POINT ( 'NONE',  ( 38.00000000000000000, 12.34694845685046616, -6.899999999999999467 ) ) ;
#119653=CARTESIAN_POINT ( 'NONE',  ( 1.500000000000000888, 15.20000000000002061, -59.79525829764741474 ) ) ;
#119703=CARTESIAN_POINT ( 'NONE',  ( -36.91746825000000598, 2.428612866367529932E-14, -4.624999997268814056 ) ) ;
#119715=LINE ( 'NONE', #89367, #79129 ) ;
#119761=DIRECTION ( 'NONE',  ( 0.000000000000000000, 0.000000000000000000, 1.000000000000000000 ) ) ;
#119822=EDGE_LOOP ( 'NONE', ( #125172, #195052, #122968, #65273 ) ) ;
#119825=ORIENTED_EDGE ( 'NONE', *, *, #107496, .T. ) ;
#119859=CARTESIAN_POINT ( 'NONE',  ( -14.65603373305124357, -15.74840231007434355, -56.32459802048661857 ) ) ;
#119874=CARTESIAN_POINT ( 'NONE',  ( 22.81625015709509441, 31.40387420917330275, -7.324999997268812457 ) ) ;
#119891=CARTESIAN_POINT ( 'NONE',  ( 10.44694540016481099, -45.05842955090996327, -23.63933302999445729 ) ) ;
#119908=EDGE_LOOP ( 'NONE', ( #18841, #183153, #159102, #85566 ) ) ;
#119942=CARTESIAN_POINT ( 'NONE',  ( 6.651581668633990515E-13, -67.16384485484805111, -24.99989890117360503 ) ) ;
#120044=ORIENTED_EDGE ( 'NONE', *, *, #158416, .T. ) ;
#120055=CARTESIAN_POINT ( 'NONE',  ( -17.18269478283316332, 17.18269478283309226, -54.21489346206828230 ) ) ;
#120103=ORIENTED_EDGE ( 'NONE', *, *, #155138, .T. ) ;
#120110=CARTESIAN_POINT ( 'NONE',  ( 36.91746825000000598, -11.99521256947793546, -2.224999997268813701 ) ) ;
#120134=LINE ( 'NONE', #75613, #118027 ) ;
#120140=CARTESIAN_POINT ( 'NONE',  ( 4.999999999999996447, 5.000000000000003553, -18.00000000000000000 ) ) ;
#120148=EDGE_CURVE ( 'NONE', #185073, #38805, #96907, .T. ) ;
#120160=CARTESIAN_POINT ( 'NONE',  ( -22.81625015709509441, -31.40387420917324590, -2.824999997268812901 ) ) ;
#120169=CARTESIAN_POINT ( 'NONE',  ( 32.09281931051394565, -20.34824190692416934, -24.99999999999997868 ) ) ;
#120176=VERTEX_POINT ( 'NONE', #74363 ) ;
#120182=CARTESIAN_POINT ( 'NONE',  ( -24.61032826407718233, -31.32210114170946724, -21.33226357149971619 ) ) ;
#120193=VERTEX_POINT ( 'NONE', #29838 ) ;
#120209=DIRECTION ( 'NONE',  ( 0.000000000000000000, 0.000000000000000000, 1.000000000000000000 ) ) ;
#120277=ORIENTED_EDGE ( 'NONE', *, *, #47276, .F. ) ;
#120307=CARTESIAN_POINT ( 'NONE',  ( -4.897001621108284297, 3.948440707545709749, -62.47584611210317007 ) ) ;
#120311=CARTESIAN_POINT ( 'NONE',  ( -23.87356034986281728, -29.32389248808953397, -21.14071813158723856 ) ) ;
#120340=EDGE_CURVE ( 'NONE', #89770, #196867, #184513, .T. ) ;
#120354=CARTESIAN_POINT ( 'NONE',  ( 20.25409705915565794, 20.61667489342684689, -52.65483682830181777 ) ) ;
#120376=CARTESIAN_POINT ( 'NONE',  ( 26.33511944008831307, -27.18111610334192463, -16.53814760372662107 ) ) ;
#120381=VERTEX_POINT ( 'NONE', #137007 ) ;
#120397=AXIS2_PLACEMENT_3D ( 'NONE', #72388, #91495, #183545 ) ;
#120431=CIRCLE ( 'NONE', #68748, 10.00000000000000000 ) ;
#120434=DIRECTION ( 'NONE',  ( -0.000000000000000000, -0.000000000000000000, -1.000000000000000000 ) ) ;
#120468=ORIENTED_EDGE ( 'NONE', *, *, #98300, .T. ) ;
#120469=CARTESIAN_POINT ( 'NONE',  ( 26.46959431505284499, -27.26463967846488146, -25.00000000000000000 ) ) ;
#120559=ORIENTED_EDGE ( 'NONE', *, *, #20458, .F. ) ;
#120597=CARTESIAN_POINT ( 'NONE',  ( 17.59990718697208223, -15.82923402486897579, -57.24447373837836039 ) ) ;
#120601=CARTESIAN_POINT ( 'NONE',  ( -0.2247805922399719325, -21.31291730435233234, -56.45983593933051026 ) ) ;
#120605=CARTESIAN_POINT ( 'NONE',  ( 0.000000000000000000, -165.0000000000000000, 12.00000000000000355 ) ) ;
#120619=CARTESIAN_POINT ( 'NONE',  ( -38.00000000000001421, 12.34694845685046438, -6.099999999999999645 ) ) ;
#120629=DIRECTION ( 'NONE',  ( 1.000000000000000000, 0.000000000000000000, 0.000000000000000000 ) ) ;
#120673=EDGE_CURVE ( 'NONE', #51008, #19818, #177633, .T. ) ;
#120715=AXIS2_PLACEMENT_3D ( 'NONE', #71659, #151499, #103995 ) ;
#120796=VERTEX_POINT ( 'NONE', #199686 ) ;
#120807=CARTESIAN_POINT ( 'NONE',  ( -21.18879603622789531, -31.24179269222070587, -19.75583340878099037 ) ) ;
#120823=DIRECTION ( 'NONE',  ( 1.000000000000000000, 0.000000000000000000, 0.000000000000000000 ) ) ;
#120847=CARTESIAN_POINT ( 'NONE',  ( 11.40812507854755253, -35.11059874428192273, -8.024999997268814411 ) ) ;
#120857=CARTESIAN_POINT ( 'NONE',  ( 1.500000000000003553, 30.40000000000004476, -47.75060438757614634 ) ) ;
#120884=ORIENTED_EDGE ( 'NONE', *, *, #138817, .T. ) ;
#120905=ORIENTED_EDGE ( 'NONE', *, *, #157130, .F. ) ;
#121020=VECTOR ( 'NONE', #158030, 1000.000000000000000 ) ;
#121027=EDGE_LOOP ( 'NONE', ( #165708, #68677, #126745 ) ) ;
#121095=CARTESIAN_POINT ( 'NONE',  ( 1.040834085586084257E-14, -30.40000000000003766, -64.92279855667830191 ) ) ;
#121099=CARTESIAN_POINT ( 'NONE',  ( -5.950531402560715689E-15, 38.81732327939063509, -5.624999997268812280 ) ) ;
#121128=AXIS2_PLACEMENT_3D ( 'NONE', #84994, #39504, #22348 ) ;
#121150=CARTESIAN_POINT ( 'NONE',  ( 22.81625015709509441, 31.40387420917330275, -9.824999997268811569 ) ) ;
#121152=DIRECTION ( 'NONE',  ( 1.000000000000000000, 0.000000000000000000, 0.000000000000000000 ) ) ;
#121172=CARTESIAN_POINT ( 'NONE',  ( -27.19415581439709939, -28.92630772671082084, -20.12198987529475147 ) ) ;
#121187=CARTESIAN_POINT ( 'NONE',  ( 38.00000000000000000, -12.34694845685040754, -10.84999999453762598 ) ) ;
#121194=LINE ( 'NONE', #182887, #191950 ) ;
#121268=ORIENTED_EDGE ( 'NONE', *, *, #48904, .T. ) ;
#121295=EDGE_CURVE ( 'NONE', #114764, #148642, #107241, .T. ) ;
#121300=CARTESIAN_POINT ( 'NONE',  ( -4.313351365237961588, 4.313351365237934054, -62.50719930893269805 ) ) ;
#121304=CARTESIAN_POINT ( 'NONE',  ( 0.1328615419017731281, 28.90000000000004476, -49.67367017693149478 ) ) ;
#121316=ORIENTED_EDGE ( 'NONE', *, *, #82044, .T. ) ;
#121340=CARTESIAN_POINT ( 'NONE',  ( -8.348819774032568475, 1.314123079931817317, -62.04874212273342948 ) ) ;
#121368=AXIS2_PLACEMENT_3D ( 'NONE', #121095, #74610, #122088 ) ;
#121369=CARTESIAN_POINT ( 'NONE',  ( 20.28159948851302374, -33.49867931359608519, -17.64937754809732695 ) ) ;
#121411=VECTOR ( 'NONE', #197014, 1000.000000000000000 ) ;
#121441=EDGE_CURVE ( 'NONE', #125394, #66168, #186777, .T. ) ;
#121460=ORIENTED_EDGE ( 'NONE', *, *, #110488, .F. ) ;
#121467=FACE_BOUND ( 'NONE', #29639, .T. ) ;
#121491=CARTESIAN_POINT ( 'NONE',  ( 30.74264578624799782, 22.33583958711400541, -4.549999994537627046 ) ) ;
#121497=CARTESIAN_POINT ( 'NONE',  ( -7.794767548047328631, 1.499903966022481994, -64.20498622968419511 ) ) ;
#121546=ORIENTED_EDGE ( 'NONE', *, *, #120673, .F. ) ;
#121549=ORIENTED_EDGE ( 'NONE', *, *, #181196, .F. ) ;
#121551=EDGE_LOOP ( 'NONE', ( #66074, #144518, #196558, #39732 ) ) ;
#121577=DIRECTION ( 'NONE',  ( -0.000000000000000000, -0.000000000000000000, -1.000000000000000000 ) ) ;
#121608=CARTESIAN_POINT ( 'NONE',  ( 30.74264578624800137, -22.33583958711395212, -5.200000000000001066 ) ) ;
#121632=VERTEX_POINT ( 'NONE', #171329 ) ;
#121661=ORIENTED_EDGE ( 'NONE', *, *, #87165, .F. ) ;
#121662=ORIENTED_EDGE ( 'NONE', *, *, #26122, .F. ) ;
#121740=DIRECTION ( 'NONE',  ( 0.000000000000000000, 0.000000000000000000, 1.000000000000000000 ) ) ;
#121743=CARTESIAN_POINT ( 'NONE',  ( -193.3062444957834884, -155.7167183371838064, -15.00000000000000178 ) ) ;
#121751=DIRECTION ( 'NONE',  ( 1.000000000000000000, 1.776356839400250465E-15, 0.000000000000000000 ) ) ;
#121788=ORIENTED_EDGE ( 'NONE', *, *, #50162, .T. ) ;
#121801=CARTESIAN_POINT ( 'NONE',  ( -12.97112549081923660, -41.39484261838730816, -20.61933656601500076 ) ) ;
#121810=EDGE_CURVE ( 'NONE', #99783, #113699, #65, .T. ) ;
#121817=CARTESIAN_POINT ( 'NONE',  ( -6.613545406318515951, -46.94410406412049497, -22.68594355512400540 ) ) ;
#121819=AXIS2_PLACEMENT_3D ( 'NONE', #69876, #158875, #66869 ) ;
#121827=CARTESIAN_POINT ( 'NONE',  ( 37.99999999999999289, 2.428612866367529932E-14, -25.00000000000000000 ) ) ;
#121832=CARTESIAN_POINT ( 'NONE',  ( 20.99598008017551365, -20.07891204798916007, -52.49574298665344685 ) ) ;
#121841=CARTESIAN_POINT ( 'NONE',  ( -29.86685920354755552, 21.69954338932564397, -6.824999997268814234 ) ) ;
#121863=CARTESIAN_POINT ( 'NONE',  ( -11.80868324581545714, -11.80868324581525997, -61.34707691135562868 ) ) ;
#121940=EDGE_CURVE ( 'NONE', #76043, #84310, #103441, .T. ) ;
#121976=EDGE_CURVE ( 'NONE', #116714, #51008, #87908, .T. ) ;
#121980=ORIENTED_EDGE ( 'NONE', *, *, #108116, .T. ) ;
#122070=CARTESIAN_POINT ( 'NONE',  ( -1.455916144794658473, -15.57302527691883576, -59.63194581529845806 ) ) ;
#122088=DIRECTION ( 'NONE',  ( 1.000000000000000000, 0.000000000000000000, 0.000000000000000000 ) ) ;
#122092=CARTESIAN_POINT ( 'NONE',  ( 22.81625015709510151, -31.40387420917324590, -2.424999997268812546 ) ) ;
#122105=CARTESIAN_POINT ( 'NONE',  ( 4.619076279717888589, 6.673813065215385087, -62.12322917040970083 ) ) ;
#122109=VECTOR ( 'NONE', #90802, 1000.000000000000000 ) ;
#122129=LINE ( 'NONE', #44312, #121411 ) ;
#122144=CARTESIAN_POINT ( 'NONE',  ( 0.3917941432913279454, 9.051283227799057585, -63.96062768057055337 ) ) ;
#122185=DIRECTION ( 'NONE',  ( 0.000000000000000000, 0.000000000000000000, 1.000000000000000000 ) ) ;
#122286=CARTESIAN_POINT ( 'NONE',  ( -6.873421141834968218, 5.266531018137379228, -62.00040165901305755 ) ) ;
#122290=CARTESIAN_POINT ( 'NONE',  ( -22.85886502250330210, 22.13519047554786567, -45.77314885760244323 ) ) ;
#122293=DIRECTION ( 'NONE',  ( 0.000000000000000000, 0.000000000000000000, 1.000000000000000000 ) ) ;
#122308=CARTESIAN_POINT ( 'NONE',  ( -3.883653825558159411, -5.178020654986570825, -62.44482655153596795 ) ) ;
#122324=ORIENTED_EDGE ( 'NONE', *, *, #15986, .T. ) ;
#122328=CARTESIAN_POINT ( 'NONE',  ( -8.945340038113732462, 0.6707077324888295333, -61.92615459704094150 ) ) ;
#122335=TOROIDAL_SURFACE ( 'NONE', #12679, 48.98979485566358250, 10.00000000000000000 ) ;
#122339=DIRECTION ( 'NONE',  ( 1.000000000000000000, 0.000000000000000000, 0.000000000000000000 ) ) ;
#122342=ADVANCED_FACE ( 'NONE', ( #75099 ), #58934, .F. ) ;
#122343=ADVANCED_FACE ( 'NONE', ( #196490 ), #135797, .F. ) ;
#122389=CARTESIAN_POINT ( 'NONE',  ( -15.64208950468055193, -40.81369178264755959, -21.33727593494802477 ) ) ;
#122419=VERTEX_POINT ( 'NONE', #90263 ) ;
#122429=DIRECTION ( 'NONE',  ( 1.000000000000000000, 0.000000000000000000, 0.000000000000000000 ) ) ;
#122502=AXIS2_PLACEMENT_3D ( 'NONE', #62598, #124276, #185972 ) ;
#122539=CARTESIAN_POINT ( 'NONE',  ( 0.000000000000000000, 0.000000000000000000, -45.64921306006598201 ) ) ;
#122579=CARTESIAN_POINT ( 'NONE',  ( 24.26175155739902323, -32.05389003868042863, -17.42962289376370677 ) ) ;
#122584=CARTESIAN_POINT ( 'NONE',  ( 15.66521691804239502, -1.429200727443413088, -59.59145728475414217 ) ) ;
#122602=CARTESIAN_POINT ( 'NONE',  ( -30.74264578624800492, 22.33583958711400186, -6.200000000000001066 ) ) ;
#122607=FACE_OUTER_BOUND ( 'NONE', #30602, .T. ) ;
#122628=CARTESIAN_POINT ( 'NONE',  ( 9.524678007105494615, -44.64363251549367106, -21.91146642400599021 ) ) ;
#122715=DIRECTION ( 'NONE',  ( 1.000000000000000000, 0.000000000000000000, 0.000000000000000000 ) ) ;
#122741=CARTESIAN_POINT ( 'NONE',  ( 14.79648886421078124, 15.41147372653644787, -56.42550976940269436 ) ) ;
#122743=CARTESIAN_POINT ( 'NONE',  ( -9.100000000000001421, 9.789526074884739315E-14, -61.89430850415821794 ) ) ;
#122793=CARTESIAN_POINT ( 'NONE',  ( -22.55660001725368247, -30.45235066354263509, -22.16622550485435994 ) ) ;
#122844=CARTESIAN_POINT ( 'NONE',  ( 39.99999999999999289, 2.428612866367529932E-14, -25.00000000000000000 ) ) ;
#122852=CARTESIAN_POINT ( 'NONE',  ( 6.300487686722097358, -38.77208804323581859, -32.75369354554603518 ) ) ;
#122909=CARTESIAN_POINT ( 'NONE',  ( -11.74264578624800670, 36.14014761921585972, -2.400000000000000355 ) ) ;
#122929=CARTESIAN_POINT ( 'NONE',  ( 1.428746744957154258, 15.66666519715284522, -61.77668719748695736 ) ) ;
#122958=DIRECTION ( 'NONE',  ( 1.000000000000000000, 0.000000000000000000, 0.000000000000000000 ) ) ;
#122968=ORIENTED_EDGE ( 'NONE', *, *, #111223, .F. ) ;
#122973=DIRECTION ( 'NONE',  ( -0.000000000000000000, -0.000000000000000000, 1.000000000000000000 ) ) ;
#123083=CARTESIAN_POINT ( 'NONE',  ( 38.00000000000000711, -12.34694845685040754, -10.84999999453762598 ) ) ;
#123096=CARTESIAN_POINT ( 'NONE',  ( 4.179973224035756552, 4.460769206500171613, -62.50518786092069945 ) ) ;
#123119=CARTESIAN_POINT ( 'NONE',  ( 11.74264578624799427, 36.14014761921585972, -8.599999999999999645 ) ) ;
#123131=LINE ( 'NONE', #139299, #122109 ) ;
#123132=CARTESIAN_POINT ( 'NONE',  ( -29.86685920354755197, -21.69954338932560134, -10.92499999726881299 ) ) ;
#123149=ORIENTED_EDGE ( 'NONE', *, *, #183499, .F. ) ;
#123155=CARTESIAN_POINT ( 'NONE',  ( -34.17105881114489563, -20.77207671795436639, -21.54825371331532935 ) ) ;
#123215=LINE ( 'NONE', #187908, #62705 ) ;
#123277=CARTESIAN_POINT ( 'NONE',  ( 0.9142611263790301201, 29.18971664064655513, -49.31446279634770491 ) ) ;
#123280=CARTESIAN_POINT ( 'NONE',  ( -26.46959431505283789, -27.26463967846487435, -25.00000000000000000 ) ) ;
#123314=CARTESIAN_POINT ( 'NONE',  ( -9.099999999999999645, 0.1001428631147401743, -61.89430850415823215 ) ) ;
#123368=CARTESIAN_POINT ( 'NONE',  ( -4.460609718571558524, 4.180103257450054066, -64.53023439669115646 ) ) ;
#123374=CARTESIAN_POINT ( 'NONE',  ( -16.67568593663830256, -39.83563513005474732, -20.80532163689326097 ) ) ;
#123413=CARTESIAN_POINT ( 'NONE',  ( -1.305043071815281008, -6.854124442542008033, -62.35408385982739077 ) ) ;
#123431=DIRECTION ( 'NONE',  ( 0.000000000000000000, 0.000000000000000000, 1.000000000000000000 ) ) ;
#123434=CARTESIAN_POINT ( 'NONE',  ( 9.687362902255726382, 9.687362902255699737, -64.92279855667830191 ) ) ;
#123473=CARTESIAN_POINT ( 'NONE',  ( -6.691186640346280967, 1.197302953328974739, -64.41832325557876970 ) ) ;
#123507=DIRECTION ( 'NONE',  ( 0.000000000000000000, 0.000000000000000000, 1.000000000000000000 ) ) ;
#123527=ORIENTED_EDGE ( 'NONE', *, *, #5609, .T. ) ;
#123529=CARTESIAN_POINT ( 'NONE',  ( -30.74264578624800492, 22.33583958711400186, -7.949999994537626513 ) ) ;
#123557=DIRECTION ( 'NONE',  ( 1.000000000000000000, 0.000000000000000000, 0.000000000000000000 ) ) ;
#123565=CARTESIAN_POINT ( 'NONE',  ( 16.70000000000002061, 0.000000000000000000, -59.13370768023891344 ) ) ;
#123575=CARTESIAN_POINT ( 'NONE',  ( -17.56609036915072153, 15.67660317299526085, -57.33766855040060051 ) ) ;
#123585=CARTESIAN_POINT ( 'NONE',  ( -6.020228577223754586E-15, 39.95556452105416412, -4.500000000000000888 ) ) ;
#123609=CARTESIAN_POINT ( 'NONE',  ( 8.139631411198177346, -37.86970803904774385, -24.01681473739955663 ) ) ;
#123757=VERTEX_POINT ( 'NONE', #46741 ) ;
#123761=VERTEX_POINT ( 'NONE', #29587 ) ;
#123773=CARTESIAN_POINT ( 'NONE',  ( -12.11826072628013584, -36.49684537641458348, -23.43927118308474178 ) ) ;
#123791=VECTOR ( 'NONE', #109155, 1000.000000000000000 ) ;
#123820=ORIENTED_EDGE ( 'NONE', *, *, #190234, .F. ) ;
#123823=FACE_OUTER_BOUND ( 'NONE', #198260, .T. ) ;
#123832=CARTESIAN_POINT ( 'NONE',  ( 9.816778487193307257, -45.49549017958584329, -23.86159105743385211 ) ) ;
#123875=ORIENTED_EDGE ( 'NONE', *, *, #136297, .T. ) ;
#123909=ADVANCED_FACE ( 'NONE', ( #172069 ), #122335, .F. ) ;
#123965=AXIS2_PLACEMENT_3D ( 'NONE', #126551, #64890, #66873 ) ;
#124028=CARTESIAN_POINT ( 'NONE',  ( -13.70000000000001528, 1.443387660838688656E-13, -64.92279855667830191 ) ) ;
#124046=CARTESIAN_POINT ( 'NONE',  ( 17.61379574983714846, -16.30506298781205743, -54.46030667112336232 ) ) ;
#124071=CARTESIAN_POINT ( 'NONE',  ( -29.86685920354755552, 21.69954338932564397, -1.324999997268813345 ) ) ;
#124084=STYLED_ITEM ( 'NONE', ( #129568 ), #100331 ) ;
#124085=CARTESIAN_POINT ( 'NONE',  ( 3.948440707545728845, 4.897001621108269198, -62.47584611210316297 ) ) ;
#124106=AXIS2_PLACEMENT_3D ( 'NONE', #189095, #186104, #50568 ) ;
#124120=ADVANCED_FACE ( 'NONE', ( #107396 ), #169069, .F. ) ;
#124123=CARTESIAN_POINT ( 'NONE',  ( 29.86685920354754842, -21.69954338932559068, -10.32499999726881335 ) ) ;
#124126=CARTESIAN_POINT ( 'NONE',  ( 0.1000683901517948615, 9.099999999999999645, -63.95112321872117889 ) ) ;
#124134=CARTESIAN_POINT ( 'NONE',  ( -10.58303160951406419, 9.244353370540759229, -62.45107349144919340 ) ) ;
#124208=VECTOR ( 'NONE', #144188, 1000.000000000000000 ) ;
#124248=VERTEX_POINT ( 'NONE', #174071 ) ;
#124276=DIRECTION ( 'NONE',  ( 0.000000000000000000, 0.000000000000000000, 1.000000000000000000 ) ) ;
#124333=CIRCLE ( 'NONE', #95181, 2.500000000000000000 ) ;
#124348=AXIS2_PLACEMENT_3D ( 'NONE', #170580, #79558, #169580 ) ;
#124365=STYLED_ITEM ( 'NONE', ( #87666 ), #9086 ) ;
#124381=CARTESIAN_POINT ( 'NONE',  ( -13.50000934768029026, -42.70547949999481574, -22.37447973961943504 ) ) ;
#124420=CARTESIAN_POINT ( 'NONE',  ( -0.7571601631681732503, -8.898623008803074441, -61.93576936796790022 ) ) ;
#124433=CARTESIAN_POINT ( 'NONE',  ( -20.43538597629143538, -20.43538597629106945, -64.92279855667830191 ) ) ;
#124434=CIRCLE ( 'NONE', #114618, 12.50000000000000000 ) ;
#124449=DIRECTION ( 'NONE',  ( -0.000000000000000000, 0.000000000000000000, 1.000000000000000000 ) ) ;
#124474=CYLINDRICAL_SURFACE ( 'NONE', #47346, 1.500000000000001332 ) ;
#124477=ADVANCED_FACE ( 'NONE', ( #111385 ), #192227, .F. ) ;
#124485=CARTESIAN_POINT ( 'NONE',  ( -19.23457310888357341, -35.06695140040310577, -26.03237767043702533 ) ) ;
#124515=AXIS2_PLACEMENT_3D ( 'NONE', #39300, #162643, #49006 ) ;
#124575=CARTESIAN_POINT ( 'NONE',  ( -1.470710558936382917, -22.45286902209804580, -55.62279185774873724 ) ) ;
#124580=CARTESIAN_POINT ( 'NONE',  ( 17.47810363111204879, -16.77070589658688604, -56.83189886071843944 ) ) ;
#124586=CARTESIAN_POINT ( 'NONE',  ( -17.62966412709571529, 16.24235425892366891, -57.02231465076383188 ) ) ;
#124605=CARTESIAN_POINT ( 'NONE',  ( 0.000000000000000000, 0.000000000000000000, -62.58071313852362039 ) ) ;
#124619=CARTESIAN_POINT ( 'NONE',  ( 20.12333042654781678, -32.04799867105307953, -20.24659421909878532 ) ) ;
#124623=ORIENTED_EDGE ( 'NONE', *, *, #76459, .F. ) ;
#124645=FACE_OUTER_BOUND ( 'NONE', #81817, .T. ) ;
#124650=CARTESIAN_POINT ( 'NONE',  ( -11.40812507854754720, -35.11059874428192273, -10.22499999726881548 ) ) ;
#124684=EDGE_CURVE ( 'NONE', #197049, #28823, #9489, .T. ) ;
#124687=DIRECTION ( 'NONE',  ( 1.000000000000000000, 0.000000000000000000, 0.000000000000000000 ) ) ;
#124690=CARTESIAN_POINT ( 'NONE',  ( 7.405410116723220249, -1.490485923554886405, -62.24175268741320366 ) ) ;
#124708=CARTESIAN_POINT ( 'NONE',  ( -20.43538597629128262, 20.43538597629122222, -52.65483682830182488 ) ) ;
#124735=CARTESIAN_POINT ( 'NONE',  ( 9.437681514439660191, 10.01085954718715598, -60.42207423661103860 ) ) ;
#124773=ORIENTED_EDGE ( 'NONE', *, *, #155029, .F. ) ;
#124788=CARTESIAN_POINT ( 'NONE',  ( -20.37447694477751980, -32.07477979233467380, -24.11443027215549506 ) ) ;
#124811=CARTESIAN_POINT ( 'NONE',  ( 22.85092056426274354, -20.84023149160054089, -47.08084238880162076 ) ) ;
#124828=CARTESIAN_POINT ( 'NONE',  ( 0.000000000000000000, 0.000000000000000000, -49.13275782002545355 ) ) ;
#124838=CARTESIAN_POINT ( 'NONE',  ( 29.86685920354754842, -21.69954338932559068, -1.824999997268813345 ) ) ;
#124848=CARTESIAN_POINT ( 'NONE',  ( 26.35664240927018653, -29.91691629194446378, -17.00538226201184600 ) ) ;
#124850=CARTESIAN_POINT ( 'NONE',  ( -10.70657341253913231, -12.25455453777589554, -61.54064628990102648 ) ) ;
#125018=EDGE_LOOP ( 'NONE', ( #87768, #87302, #101949 ) ) ;
#125071=CARTESIAN_POINT ( 'NONE',  ( 1.468936857220423775, 22.44461420004035901, -58.07763101479264378 ) ) ;
#125086=CARTESIAN_POINT ( 'NONE',  ( 3.556970738554033499E-15, -38.81732327939057825, -8.624999997268814056 ) ) ;
#125094=CARTESIAN_POINT ( 'NONE',  ( 0.000000000000000000, -105.0000000000000000, 7.000000000000003553 ) ) ;
#125124=CARTESIAN_POINT ( 'NONE',  ( 2.500000000000000000, -165.0000000000000000, 12.00000000000000355 ) ) ;
#125126=EDGE_CURVE ( 'NONE', #93910, #140935, #11214, .T. ) ;
#125138=CARTESIAN_POINT ( 'NONE',  ( 3.556970738554033499E-15, -38.81732327939057825, -6.624999997268814056 ) ) ;
#125139=CARTESIAN_POINT ( 'NONE',  ( 0.4292098674014996895, 24.24132924781739362, -56.81486547910376572 ) ) ;
#125146=CARTESIAN_POINT ( 'NONE',  ( 11.19179774862115018, -35.88147526272302912, -30.64906824478838843 ) ) ;
#125160=CARTESIAN_POINT ( 'NONE',  ( -35.08666314276963760, -21.80769648729559407, -18.77091308352783017 ) ) ;
#125161=ORIENTED_EDGE ( 'NONE', *, *, #5777, .F. ) ;
#125172=ORIENTED_EDGE ( 'NONE', *, *, #43025, .T. ) ;
#125174=CIRCLE ( 'NONE', #37993, 48.98979485566358250 ) ;
#125223=LINE ( 'NONE', #67516, #151157 ) ;
#125225=CARTESIAN_POINT ( 'NONE',  ( -6.100000000000006750, 6.426762577456935076E-14, -64.53213882399991519 ) ) ;
#125272=EDGE_CURVE ( 'NONE', #156405, #164148, #181747, .T. ) ;
#125327=CARTESIAN_POINT ( 'NONE',  ( 193.3062444957835453, -155.7167183371837496, -15.00000000000000178 ) ) ;
#125347=EDGE_CURVE ( 'NONE', #143210, #56919, #151514, .T. ) ;
#125361=VERTEX_POINT ( 'NONE', #26388 ) ;
#125382=CARTESIAN_POINT ( 'NONE',  ( -1.054302444749779077, -31.48176515315803670, -46.25693415911323569 ) ) ;
#125394=VERTEX_POINT ( 'NONE', #116374 ) ;
#125425=CARTESIAN_POINT ( 'NONE',  ( -14.82342540975555600, 1.464556741314251731, -62.12362001602809869 ) ) ;
#125471=EDGE_CURVE ( 'NONE', #42510, #171133, #70879, .T. ) ;
#125573=CARTESIAN_POINT ( 'NONE',  ( 0.000000000000000000, 0.000000000000000000, -63.95112321872120731 ) ) ;
#125575=DIRECTION ( 'NONE',  ( -1.000000000000000000, -8.921435019309295657E-15, 0.000000000000000000 ) ) ;
#125579=SPHERICAL_SURFACE ( 'NONE', #85699, 38.00000000000002132 ) ;
#125593=CARTESIAN_POINT ( 'NONE',  ( -38.00000000000001421, -12.34694845685042708, -9.899999999999998579 ) ) ;
#125617=CARTESIAN_POINT ( 'NONE',  ( 10.65591991699549368, -43.63381331854910172, -21.52219975116264195 ) ) ;
#125621=ORIENTED_EDGE ( 'NONE', *, *, #65973, .F. ) ;
#125649=AXIS2_PLACEMENT_3D ( 'NONE', #25396, #131543, #165887 ) ;
#125729=CARTESIAN_POINT ( 'NONE',  ( 9.822817408787017257, 11.94368209565400640, -59.71171441009363434 ) ) ;
#125731=DIRECTION ( 'NONE',  ( -0.000000000000000000, -0.000000000000000000, -1.000000000000000000 ) ) ;
#125765=ORIENTED_EDGE ( 'NONE', *, *, #68000, .F. ) ;
#125769=EDGE_LOOP ( 'NONE', ( #34746, #64908, #70959, #118208 ) ) ;
#125802=CARTESIAN_POINT ( 'NONE',  ( 11.74264578624800315, -36.14014761921581709, -9.400000000000000355 ) ) ;
#125805=CARTESIAN_POINT ( 'NONE',  ( 4.180103257450070942, 4.460609718571543425, -64.53023439669115646 ) ) ;
#125819=LINE ( 'NONE', #172324, #114254 ) ;
#125826=ORIENTED_EDGE ( 'NONE', *, *, #197214, .T. ) ;
#125829=CARTESIAN_POINT ( 'NONE',  ( -11.40812507854754720, -35.11059874428192273, -6.224999997268812812 ) ) ;
#125839=CARTESIAN_POINT ( 'NONE',  ( 27.28412861566094350, -28.99984389462593271, -16.93987563810616592 ) ) ;
#125853=EDGE_CURVE ( 'NONE', #140780, #196237, #190175, .T. ) ;
#125891=CARTESIAN_POINT ( 'NONE',  ( 29.86685920354754487, 21.69954338932564752, -9.924999997268812990 ) ) ;
#125895=CYLINDRICAL_SURFACE ( 'NONE', #107716, 1.500000000000001332 ) ;
#125907=EDGE_LOOP ( 'NONE', ( #82607, #195535, #8163, #118621 ) ) ;
#125975=AXIS2_PLACEMENT_3D ( 'NONE', #54922, #145918, #55918 ) ;
#126003=B_SPLINE_CURVE_WITH_KNOTS ( 'NONE', 3,
 ( #137488, #199168, #196221, #105172, #151680, #60635, #103187 ),
 .UNSPECIFIED., .F., .F.,
 ( 4, 3, 4 ),
 ( 0.006882574723720362095, 0.01376514944744072419, 0.01380547055123299352 ),
 .UNSPECIFIED. ) ;
#126053=CARTESIAN_POINT ( 'NONE',  ( 0.8267425368004359676, 21.53050622130930591, -56.30180790818311465 ) ) ;
#126056=FACE_OUTER_BOUND ( 'NONE', #134794, .T. ) ;
#126062=CARTESIAN_POINT ( 'NONE',  ( -22.22593230296001465, -22.81042121942878609, -45.72930070417675097 ) ) ;
#126066=ADVANCED_FACE ( 'NONE', ( #13199 ), #136524, .F. ) ;
#126073=CYLINDRICAL_SURFACE ( 'NONE', #198014, 28.90000000000004476 ) ;
#126076=CARTESIAN_POINT ( 'NONE',  ( -2.500000000000000000, -105.0000000000000000, 7.000000000000003553 ) ) ;
#126088=CARTESIAN_POINT ( 'NONE',  ( 12.24802307403548518, -10.94040653594595724, -59.26855811195190427 ) ) ;
#126097=( BOUNDED_CURVE ( )  B_SPLINE_CURVE ( 2, ( #97833, #159521, #21018, #115027, #45914, #108573, #132194 ),
 .UNSPECIFIED., .F., .F. ) 
 B_SPLINE_CURVE_WITH_KNOTS ( ( 3, 2, 2, 3 ),
 ( 0.9255006513465138251, 0.9399999999999999467, 0.9599999999999999645, 0.9744993486534860860 ),
 .UNSPECIFIED. ) 
 CURVE ( )  GEOMETRIC_REPRESENTATION_ITEM ( )  RATIONAL_B_SPLINE_CURVE ( ( 0.9804823514139773266, 0.9645175682723605703, 1.000000000000000000, 0.9510565162951535312, 1.000000000000000000, 0.9645175682723607924, 0.9804823514139775487 ) ) 
 REPRESENTATION_ITEM ( '' )  );
#126109=CIRCLE ( 'NONE', #84091, 12.50000000000000000 ) ;
#126126=CARTESIAN_POINT ( 'NONE',  ( -22.81625015709509441, -31.40387420917324590, -6.824999997268814234 ) ) ;
#126147=CARTESIAN_POINT ( 'NONE',  ( -33.12942481080120416, -22.41379292486517016, -24.08540372093838045 ) ) ;
#126159=VERTEX_POINT ( 'NONE', #93987 ) ;
#126212=CARTESIAN_POINT ( 'NONE',  ( -4.313351365237979351, -4.313351365237916291, -64.92279855667830191 ) ) ;
#126269=DIRECTION ( 'NONE',  ( -0.000000000000000000, -0.000000000000000000, -1.000000000000000000 ) ) ;
#126308=DIRECTION ( 'NONE',  ( -0.000000000000000000, -0.000000000000000000, 1.000000000000000000 ) ) ;
#126310=FACE_OUTER_BOUND ( 'NONE', #111894, .T. ) ;
#126321=CARTESIAN_POINT ( 'NONE',  ( 25.96435248595184220, -27.35529834266878524, -20.33897993952045979 ) ) ;
#126341=ORIENTED_EDGE ( 'NONE', *, *, #107092, .T. ) ;
#126376=VERTEX_POINT ( 'NONE', #98947 ) ;
#126397=CARTESIAN_POINT ( 'NONE',  ( -30.74264578624800492, -22.33583958711396278, -9.549999994537627046 ) ) ;
#126399=CARTESIAN_POINT ( 'NONE',  ( 1.227931366032057224E-14, 24.30000000000003268, -65.00100000000003320 ) ) ;
#126428=DIRECTION ( 'NONE',  ( -0.3041824702427683436, -0.9526137857479322069, 2.960637879548173518E-15 ) ) ;
#126431=CARTESIAN_POINT ( 'NONE',  ( -17.10305700086924929, -33.88765926517217508, -26.94085628989254033 ) ) ;
#126470=DIRECTION ( 'NONE',  ( 0.000000000000000000, -1.000000000000000000, 0.000000000000000000 ) ) ;
#126521=CARTESIAN_POINT ( 'NONE',  ( -11.30153831258471975, -180.0000000000000000, -15.00000000000000178 ) ) ;
#126530=CARTESIAN_POINT ( 'NONE',  ( 14.82342540975558443, -1.464556741314153587, -62.12362001602809869 ) ) ;
#126551=CARTESIAN_POINT ( 'NONE',  ( -1.734723475976807094E-15, 15.20000000000001883, -65.00100000000003320 ) ) ;
#126569=VERTEX_POINT ( 'NONE', #110158 ) ;
#126594=CARTESIAN_POINT ( 'NONE',  ( 28.03896471500612719, -25.30868469084780870, -20.82118626250830573 ) ) ;
#126630=CARTESIAN_POINT ( 'NONE',  ( -11.30153831258471975, -180.0000000000000000, -15.00000000000000178 ) ) ;
#126659=CARTESIAN_POINT ( 'NONE',  ( 7.122238460089383771, -1.425225664899866684, -62.29949481927938137 ) ) ;
#126702=CARTESIAN_POINT ( 'NONE',  ( 10.91206588261563759, 12.25194888441100716, -59.27621954310798458 ) ) ;
#126741=ORIENTED_EDGE ( 'NONE', *, *, #74517, .T. ) ;
#126745=ORIENTED_EDGE ( 'NONE', *, *, #99054, .T. ) ;
#126746=CARTESIAN_POINT ( 'NONE',  ( 17.18269478283314911, 17.18269478283310647, -54.21489346206828230 ) ) ;
#126756=CARTESIAN_POINT ( 'NONE',  ( -26.43919995774735554, -26.89423752947756441, -20.34026575423078853 ) ) ;
#126784=DIRECTION ( 'NONE',  ( -0.000000000000000000, -0.000000000000000000, 1.000000000000000000 ) ) ;
#126803=CARTESIAN_POINT ( 'NONE',  ( 22.81625015709509441, 31.40387420917330275, -3.324999997268812901 ) ) ;
#126809=EDGE_CURVE ( 'NONE', #117002, #17032, #109480, .T. ) ;
#126815=CARTESIAN_POINT ( 'NONE',  ( 23.69010019207190965, -31.82897765506827881, -19.48018210901874525 ) ) ;
#126866=CARTESIAN_POINT ( 'NONE',  ( -36.91746825000001309, 11.99521256947798342, -0.7249999972688133676 ) ) ;
#126867=DIRECTION ( 'NONE',  ( -0.000000000000000000, 0.000000000000000000, 1.000000000000000000 ) ) ;
#126900=DIRECTION ( 'NONE',  ( -0.000000000000000000, -0.000000000000000000, -1.000000000000000000 ) ) ;
#126901=DIRECTION ( 'NONE',  ( 1.000000000000000000, 0.000000000000000000, 0.000000000000000000 ) ) ;
#126902=CARTESIAN_POINT ( 'NONE',  ( 38.00000000000000000, -12.34694845685040754, -1.099999999999999645 ) ) ;
#126933=VERTEX_POINT ( 'NONE', #146453 ) ;
#127028=CARTESIAN_POINT ( 'NONE',  ( -193.3062444957834884, -155.7167183371838064, 0.000000000000000000 ) ) ;
#127029=CARTESIAN_POINT ( 'NONE',  ( 0.4883415225378692215, 9.021730311186841433, -61.91042889546767469 ) ) ;
#127032=CARTESIAN_POINT ( 'NONE',  ( 12.50000000000001066, -90.00000000000005684, 0.000000000000000000 ) ) ;
#127053=CARTESIAN_POINT ( 'NONE',  ( 11.40812507854755253, -35.11059874428192273, -8.524999997268814411 ) ) ;
#127093=EDGE_LOOP ( 'NONE', ( #99187, #162199, #33074, #81522, #141916, #76278, #100027, #21575, #24206, #162642 ) ) ;
#127097=CARTESIAN_POINT ( 'NONE',  ( 37.66961640367472341, 5.000000000000023981, -25.00000000000000000 ) ) ;
#127100=CARTESIAN_POINT ( 'NONE',  ( 11.40812507854754365, 35.11059874428196537, -7.724999997268813701 ) ) ;
#127105=AXIS2_PLACEMENT_3D ( 'NONE', #24162, #116153, #88810 ) ;
#127187=FACE_OUTER_BOUND ( 'NONE', #101947, .T. ) ;
#127209=DIRECTION ( 'NONE',  ( 0.000000000000000000, 0.000000000000000000, 1.000000000000000000 ) ) ;
#127287=LINE ( 'NONE', #152910, #43880 ) ;
#127299=DIRECTION ( 'NONE',  ( 1.000000000000000000, 0.000000000000000000, 0.000000000000000000 ) ) ;
#127301=VERTEX_POINT ( 'NONE', #176675 ) ;
#127303=CIRCLE ( 'NONE', #49816, 6.100000000000006750 ) ;
#127324=EDGE_LOOP ( 'NONE', ( #182512, #77573, #140750, #32963 ) ) ;
#127340=DIRECTION ( 'NONE',  ( 1.000000000000000000, 0.000000000000000000, 0.000000000000000000 ) ) ;
#127347=CARTESIAN_POINT ( 'NONE',  ( -2.577820198429831642E-15, -9.100000000000001421, -63.95112321872120731 ) ) ;
#127360=CARTESIAN_POINT ( 'NONE',  ( -3.964304649048260742, -40.57928608015912175, -25.32305239478594672 ) ) ;
#127362=EDGE_LOOP ( 'NONE', ( #181793, #121980, #138796, #124773 ) ) ;
#127387=VECTOR ( 'NONE', #16764, 1000.000000000000000 ) ;
#127396=DIRECTION ( 'NONE',  ( 1.000000000000000000, 0.000000000000000000, 0.000000000000000000 ) ) ;
#127416=CIRCLE ( 'NONE', #56297, 16.70000000000002061 ) ;
#127417=DIRECTION ( 'NONE',  ( -0.000000000000000000, -0.000000000000000000, 1.000000000000000000 ) ) ;
#127459=CARTESIAN_POINT ( 'NONE',  ( -9.841528761215647236, -38.18405872352760611, -31.73089324721045656 ) ) ;
#127503=CIRCLE ( 'NONE', #66159, 8.000000000000000000 ) ;
#127545=DIRECTION ( 'NONE',  ( 0.000000000000000000, 0.000000000000000000, 1.000000000000000000 ) ) ;
#127556=FACE_BOUND ( 'NONE', #117491, .T. ) ;
#127561=CARTESIAN_POINT ( 'NONE',  ( 37.66961640367472341, 5.000000000000023981, -15.00000000000000000 ) ) ;
#127563=CIRCLE ( 'NONE', #172766, 5.000000000000000000 ) ;
#127568=VERTEX_POINT ( 'NONE', #189603 ) ;
#127591=SURFACE_STYLE_FILL_AREA ( #7232 ) ;
#127595=CARTESIAN_POINT ( 'NONE',  ( 26.91739389984235942, -26.09363094301860642, -18.46721497145071211 ) ) ;
#127660=CARTESIAN_POINT ( 'NONE',  ( 8.898623008803079770, -0.7571601631681817990, -61.93576936796788601 ) ) ;
#127703=FACE_OUTER_BOUND ( 'NONE', #32865, .T. ) ;
#127753=ORIENTED_EDGE ( 'NONE', *, *, #145835, .T. ) ;
#127755=CARTESIAN_POINT ( 'NONE',  ( -28.83006054357406711, -24.83490584245891597, -16.72457388843617920 ) ) ;
#127759=EDGE_CURVE ( 'NONE', #101645, #188707, #80606, .T. ) ;
#127771=EDGE_LOOP ( 'NONE', ( #112149, #9789, #103025, #183596 ) ) ;
#127773=DIRECTION ( 'NONE',  ( -0.000000000000000000, -0.000000000000000000, 1.000000000000000000 ) ) ;
#127778=CARTESIAN_POINT ( 'NONE',  ( -29.41559601785653655, 1.135674102528529295, -49.03020479230152517 ) ) ;
#127799=VERTEX_POINT ( 'NONE', #129880 ) ;
#127801=CARTESIAN_POINT ( 'NONE',  ( 36.91746825000000598, -11.99521256947793546, -3.724999997268812812 ) ) ;
#127811=CARTESIAN_POINT ( 'NONE',  ( 27.05031264677070979, -29.22974442244436588, -16.95124367203838744 ) ) ;
#127850=CYLINDRICAL_SURFACE ( 'NONE', #5499, 24.30000000000003268 ) ;
#127863=CARTESIAN_POINT ( 'NONE',  ( -22.81625015709510507, 31.40387420917330275, -9.424999997268812990 ) ) ;
#127864=LINE ( 'NONE', #189568, #160480 ) ;
#127898=CARTESIAN_POINT ( 'NONE',  ( 31.90000000000004476, -0.1282610754044114509, -49.13275782002542513 ) ) ;
#127956=ADVANCED_FACE ( 'NONE', ( #102578 ), #191579, .T. ) ;
#127970=EDGE_CURVE ( 'NONE', #76158, #182346, #38625, .T. ) ;
#127987=AXIS2_PLACEMENT_3D ( 'NONE', #57691, #166858, #136498 ) ;
#128011=CARTESIAN_POINT ( 'NONE',  ( 21.81714873624722628, 22.96531869715549234, -45.99103957044146540 ) ) ;
#128016=CARTESIAN_POINT ( 'NONE',  ( -3.573655867282028392E-15, 2.428612866367529932E-14, -25.00000000000000000 ) ) ;
#128042=ORIENTED_EDGE ( 'NONE', *, *, #150161, .F. ) ;
#128045=VERTEX_POINT ( 'NONE', #178429 ) ;
#128051=CARTESIAN_POINT ( 'NONE',  ( 29.86685920354754487, 21.69954338932564752, -9.924999997268812990 ) ) ;
#128097=CARTESIAN_POINT ( 'NONE',  ( -36.91746825000001309, 11.99521256947798342, -3.224999997268813257 ) ) ;
#128121=ADVANCED_FACE ( 'NONE', ( #149088 ), #99564, .T. ) ;
#128132=ADVANCED_FACE ( 'NONE', ( #8570 ), #70245, .F. ) ;
#128135=VECTOR ( 'NONE', #83354, 1000.000000000000000 ) ;
#128148=AXIS2_PLACEMENT_3D ( 'NONE', #129240, #82739, #101919 ) ;
#128181=VECTOR ( 'NONE', #67185, 1000.000000000000000 ) ;
#128220=ORIENTED_EDGE ( 'NONE', *, *, #73153, .F. ) ;
#128251=CARTESIAN_POINT ( 'NONE',  ( -26.46959431505279525, -27.26463967846491698, -11.49588912907431393 ) ) ;
#128273=CIRCLE ( 'NONE', #28312, 4.000000000000000888 ) ;
#128283=CARTESIAN_POINT ( 'NONE',  ( 27.98120534312134922, -28.16303873514628364, -20.10652275068718708 ) ) ;
#128285=CARTESIAN_POINT ( 'NONE',  ( 11.74264578624799427, 36.14014761921585972, -2.349999994537626868 ) ) ;
#128295=CARTESIAN_POINT ( 'NONE',  ( 21.23184647844207618, -181.1785498424364675, -15.00000000000000178 ) ) ;
#128354=CARTESIAN_POINT ( 'NONE',  ( -15.71981542752435423, -36.60361700297588072, -28.71911170261294899 ) ) ;
#128356=ORIENTED_EDGE ( 'NONE', *, *, #85361, .F. ) ;
#128407=AXIS2_PLACEMENT_3D ( 'NONE', #23427, #36574, #97237 ) ;
#128420=CARTESIAN_POINT ( 'NONE',  ( -5.374011537017778117, 5.374011537017756801, -65.00100000000003320 ) ) ;
#128444=CARTESIAN_POINT ( 'NONE',  ( 69.65682714487590488, -71.74905178543389184, -25.00000000000000000 ) ) ;
#128478=B_SPLINE_CURVE_WITH_KNOTS ( 'NONE', 3,
 ( #185265, #172082, #1222, #65882, #46757, #124580, #174083, #141733, #232, #78065 ),
 .UNSPECIFIED., .F., .F.,
 ( 4, 2, 2, 2, 4 ),
 ( 0.003992163664268632249, 0.004297753711354872219, 0.004603343758441113057, 0.004908933805527353894, 0.005214523852613593864 ),
 .UNSPECIFIED. ) ;
#128483=CARTESIAN_POINT ( 'NONE',  ( -15.03002592745795774, -17.15945613581673257, -57.85847139087537983 ) ) ;
#128546=CARTESIAN_POINT ( 'NONE',  ( -16.49581645235992156, 0.7820921006974912437, -59.22453004090982631 ) ) ;
#128552=EDGE_CURVE ( 'NONE', #46712, #45827, #183972, .T. ) ;
#128559=CARTESIAN_POINT ( 'NONE',  ( 37.99999999999999289, 2.893978650043524126E-14, -9.000000000000001776 ) ) ;
#128574=CIRCLE ( 'NONE', #80238, 6.100000000000006750 ) ;
#128579=( NAMED_UNIT ( * ) SI_UNIT ( $, .STERADIAN. ) SOLID_ANGLE_UNIT ( ) );
#128583=CARTESIAN_POINT ( 'NONE',  ( 25.90290776672146222, -27.60635150542609750, -16.55190051048762001 ) ) ;
#128693=CARTESIAN_POINT ( 'NONE',  ( 9.389996629557208152, 10.10305183197209544, -60.40856999928715254 ) ) ;
#128732=ORIENTED_EDGE ( 'NONE', *, *, #42790, .T. ) ;
#128737=ORIENTED_EDGE ( 'NONE', *, *, #182320, .F. ) ;
#128747=CARTESIAN_POINT ( 'NONE',  ( -30.24683373042578083, -22.89668476416583687, -22.64123003232879228 ) ) ;
#128769=CARTESIAN_POINT ( 'NONE',  ( -28.98522958361496293, 0.5143648618589782284, -49.56847006845431025 ) ) ;
#128772=DIRECTION ( 'NONE',  ( -0.000000000000000000, -0.000000000000000000, 1.000000000000000000 ) ) ;
#128773=CARTESIAN_POINT ( 'NONE',  ( 30.74264578624800137, -22.33583958711395212, -6.949999994537627401 ) ) ;
#128778=CARTESIAN_POINT ( 'NONE',  ( 33.78191506369888941, -21.41920200728860380, -24.99999999999997868 ) ) ;
#128795=CARTESIAN_POINT ( 'NONE',  ( -29.86685920354755552, 21.69954338932564397, -0.8249999972688133454 ) ) ;
#128819=DIRECTION ( 'NONE',  ( -1.000000000000000000, 0.000000000000000000, 0.000000000000000000 ) ) ;
#128823=ORIENTED_EDGE ( 'NONE', *, *, #55964, .T. ) ;
#128842=CARTESIAN_POINT ( 'NONE',  ( -16.12203461105333702, 16.12203461105326951, -65.00100000000003320 ) ) ;
#128854=CARTESIAN_POINT ( 'NONE',  ( -36.91746825000000598, 2.428612866367529932E-14, -11.12499999726881228 ) ) ;
#128862=CARTESIAN_POINT ( 'NONE',  ( 37.99999999999999289, 2.893978650043524126E-14, -2.749999994537626780 ) ) ;
#128888=CARTESIAN_POINT ( 'NONE',  ( 3.766062262543149401E-15, -39.95556452105413570, -1.499999999999999778 ) ) ;
#129016=CARTESIAN_POINT ( 'NONE',  ( 0.1121086616460852114, 21.30000000000003268, -56.46919128290400636 ) ) ;
#129033=ORIENTED_EDGE ( 'NONE', *, *, #195501, .F. ) ;
#129046=LINE ( 'NONE', #6705, #108232 ) ;
#129079=B_SPLINE_CURVE_WITH_KNOTS ( 'NONE', 3,
 ( #174937, #113247, #49599, #51582, #142594, #191101, #81890, #3092, #160759, #157781, #6068, #64769, #126431, #129404, #143583, #36400 ),
 .UNSPECIFIED., .F., .F.,
 ( 4, 2, 2, 2, 2, 2, 2, 4 ),
 ( 0.000000000000000000, 0.004834299366836557893, 0.006042874208545700836, 0.007251449050254843778, 0.009668598733673129664, 0.01450289810050969970, 0.01692004778392798212, 0.01933719746734626627 ),
 .UNSPECIFIED. ) ;
#129082=EDGE_CURVE ( 'NONE', #74887, #22341, #159472, .T. ) ;
#129086=CARTESIAN_POINT ( 'NONE',  ( -5.950531402560715689E-15, 38.81732327939063509, -5.624999997268812280 ) ) ;
#129102=EDGE_LOOP ( 'NONE', ( #3786, #76045, #184345, #10075, #92816 ) ) ;
#129110=ORIENTED_EDGE ( 'NONE', *, *, #116420, .T. ) ;
#129173=CYLINDRICAL_SURFACE ( 'NONE', #18779, 16.70000000000002061 ) ;
#129175=CARTESIAN_POINT ( 'NONE',  ( -36.91746825000000598, 2.428612866367529932E-14, -0.6249999972688132788 ) ) ;
#129238=FACE_OUTER_BOUND ( 'NONE', #141123, .T. ) ;
#129240=CARTESIAN_POINT ( 'NONE',  ( -11.30153831258470731, -180.0000000000000000, 0.000000000000000000 ) ) ;
#129257=CARTESIAN_POINT ( 'NONE',  ( 26.46959431505284499, -27.26463967846488146, -25.00000000000000000 ) ) ;
#129271=ORIENTED_EDGE ( 'NONE', *, *, #20851, .T. ) ;
#129274=CARTESIAN_POINT ( 'NONE',  ( 193.3062444957835453, -155.7167183371837496, 0.000000000000000000 ) ) ;
#129287=DIRECTION ( 'NONE',  ( 0.000000000000000000, 0.000000000000000000, 1.000000000000000000 ) ) ;
#129290=CARTESIAN_POINT ( 'NONE',  ( 1.221313414957698099E-14, -31.90000000000003411, -49.13275782002545355 ) ) ;
#129327=CARTESIAN_POINT ( 'NONE',  ( -38.00000000000000711, 2.893978650043524126E-14, -24.99999999999997868 ) ) ;
#129334=CARTESIAN_POINT ( 'NONE',  ( -0.8274645171313256276, -29.14368513529649007, -49.37167794572891921 ) ) ;
#129347=CARTESIAN_POINT ( 'NONE',  ( -11.26676076909002155, -37.89014424912453904, -31.17854569212617832 ) ) ;
#129404=CARTESIAN_POINT ( 'NONE',  ( -18.27284445343937236, -33.31360383038296646, -25.98075878691516039 ) ) ;
#129491=EDGE_CURVE ( 'NONE', #196218, #158096, #51464, .T. ) ;
#129532=CARTESIAN_POINT ( 'NONE',  ( 3.766062262543149401E-15, -39.95556452105413570, -5.249999994537625447 ) ) ;
#129539=CARTESIAN_POINT ( 'NONE',  ( -16.70000000000002061, 0.1037895044724580218, -59.13370768023892055 ) ) ;
#129568=PRESENTATION_STYLE_ASSIGNMENT (( #67915 ) ) ;
#129569=CARTESIAN_POINT ( 'NONE',  ( 23.48529157249599564, 32.32473071737754111, -10.44999999453762562 ) ) ;
#129572=CARTESIAN_POINT ( 'NONE',  ( 35.57212018829687139, -18.96864681236966277, -18.54270186059541814 ) ) ;
#129580=EDGE_LOOP ( 'NONE', ( #120468, #28203, #32357, #15676 ) ) ;
#129633=DIRECTION ( 'NONE',  ( 0.000000000000000000, 0.000000000000000000, 1.000000000000000000 ) ) ;
#129674=CARTESIAN_POINT ( 'NONE',  ( -27.86273085795036408, -28.69962071417357663, -15.00000000000000178 ) ) ;
#129681=CARTESIAN_POINT ( 'NONE',  ( 69.65682714487590488, -71.74905178543389184, -15.00000000000000178 ) ) ;
#129746=CARTESIAN_POINT ( 'NONE',  ( 28.90000000000004476, 0.000000000000000000, -49.67367017693150189 ) ) ;
#129777=ORIENTED_EDGE ( 'NONE', *, *, #117749, .F. ) ;
#129780=CARTESIAN_POINT ( 'NONE',  ( -22.81625015709509441, -31.40387420917324590, -10.32499999726881157 ) ) ;
#129837=ORIENTED_EDGE ( 'NONE', *, *, #46651, .F. ) ;
#129842=CARTESIAN_POINT ( 'NONE',  ( -36.91746825000000598, 2.428612866367529932E-14, -0.6249999972688132788 ) ) ;
#129852=EDGE_CURVE ( 'NONE', #196867, #69099, #177498, .T. ) ;
#129880=CARTESIAN_POINT ( 'NONE',  ( -2.577820198429831642E-15, -9.100000000000001421, -61.89430850415821794 ) ) ;
#129898=LINE ( 'NONE', #37922, #177800 ) ;
#129987=CARTESIAN_POINT ( 'NONE',  ( 20.33951628977429849, 20.53125566280822056, -49.67367017693150189 ) ) ;
#129992=DIRECTION ( 'NONE',  ( 1.000000000000000000, 0.000000000000000000, -0.000000000000000000 ) ) ;
#130002=CARTESIAN_POINT ( 'NONE',  ( -25.13006352617138006, -30.86725525062055553, -20.93759803324971713 ) ) ;
#130012=CARTESIAN_POINT ( 'NONE',  ( 0.000000000000000000, 0.000000000000000000, -58.85720012050612837 ) ) ;
#130014=CARTESIAN_POINT ( 'NONE',  ( -29.86685920354755552, 21.69954338932564397, -0.8249999972688133454 ) ) ;
#130021=ORIENTED_EDGE ( 'NONE', *, *, #82833, .T. ) ;
#130023=ADVANCED_FACE ( 'NONE', ( #192347 ), #115504, .T. ) ;
#130059=EDGE_CURVE ( 'NONE', #130796, #137721, #117497, .T. ) ;
#130072=CIRCLE ( 'NONE', #155926, 4.000000000000000888 ) ;
#130078=B_SPLINE_CURVE_WITH_KNOTS ( 'NONE', 3,
 ( #45232, #106886, #164602, #165599, #196940, #198913, #60382, #72594, #30057, #134268 ),
 .UNSPECIFIED., .F., .F.,
 ( 4, 2, 2, 2, 4 ),
 ( 0.002455067421798150240, 0.003068445128277203469, 0.003681822834756256699, 0.004295200541235309928, 0.004908578247714363157 ),
 .UNSPECIFIED. ) ;
#130079=CARTESIAN_POINT ( 'NONE',  ( -22.72511982729796287, 22.36433501015060799, -49.15411784021379304 ) ) ;
#130103=ORIENTED_EDGE ( 'NONE', *, *, #68244, .F. ) ;
#130215=CIRCLE ( 'NONE', #188417, 59.99999999999998579 ) ;
#130230=CARTESIAN_POINT ( 'NONE',  ( 0.000000000000000000, -78.67194367458512261, -25.00000000000000000 ) ) ;
#130248=CARTESIAN_POINT ( 'NONE',  ( 15.77906466954398113, -14.65353482790562012, -56.31012573826036771 ) ) ;
#130265=DIRECTION ( 'NONE',  ( 1.000000000000000000, 0.000000000000000000, 0.000000000000000000 ) ) ;
#130279=AXIS2_PLACEMENT_3D ( 'NONE', #171588, #80552, #174576 ) ;
#130331=DIRECTION ( 'NONE',  ( -1.000000000000000000, 0.000000000000000000, 0.000000000000000000 ) ) ;
#130332=ORIENTED_EDGE ( 'NONE', *, *, #29329, .F. ) ;
#130338=CARTESIAN_POINT ( 'NONE',  ( -14.22875182907677072, -42.06737590810060112, -22.02417070750285788 ) ) ;
#130374=DIRECTION ( 'NONE',  ( 1.000000000000000000, 0.000000000000000000, 0.000000000000000000 ) ) ;
#130418=AXIS2_PLACEMENT_3D ( 'NONE', #64155, #78309, #139982 ) ;
#130443=ORIENTED_EDGE ( 'NONE', *, *, #63444, .F. ) ;
#130448=AXIS2_PLACEMENT_3D ( 'NONE', #25, #137559, #75884 ) ;
#130478=CARTESIAN_POINT ( 'NONE',  ( -14.62203461105063873, -16.12203461105573865, -58.56003730381080175 ) ) ;
#130499=VERTEX_POINT ( 'NONE', #152800 ) ;
#130555=ORIENTED_EDGE ( 'NONE', *, *, #2746, .T. ) ;
#130580=CARTESIAN_POINT ( 'NONE',  ( 37.99999999999999289, 12.34694845685046793, -10.64999999453762669 ) ) ;
#130583=CARTESIAN_POINT ( 'NONE',  ( 27.29882810768421919, -25.71095057349885948, -18.52182797988482221 ) ) ;
#130602=EDGE_CURVE ( 'NONE', #166806, #126933, #67622, .T. ) ;
#130640=EDGE_CURVE ( 'NONE', #12139, #197947, #149834, .T. ) ;
#130657=AXIS2_PLACEMENT_3D ( 'NONE', #105058, #167724, #103066 ) ;
#130705=B_SPLINE_CURVE_WITH_KNOTS ( 'NONE', 3,
 ( #130478, #191176, #98131, #176016, #128483, #178013, #7136, #131490, #66820, #52650, #192175, #175010, #177024, #117324, #36474, #39480 ),
 .UNSPECIFIED., .F., .F.,
 ( 4, 2, 2, 2, 2, 2, 2, 4 ),
 ( 0.001218919368246023033, 0.002217820489337911892, 0.002717271049883857731, 0.003216721610429803570, 0.003716172170975749409, 0.004215622731521694380, 0.004715073292067640219, 0.005214523852613586058 ),
 .UNSPECIFIED. ) ;
#130715=AXIS2_PLACEMENT_3D ( 'NONE', #60072, #2371, #48888 ) ;
#130737=EDGE_LOOP ( 'NONE', ( #165681, #38569, #71952, #45156 ) ) ;
#130747=CIRCLE ( 'NONE', #108085, 4.000000000000000888 ) ;
#130773=CARTESIAN_POINT ( 'NONE',  ( -31.90000000000003411, 3.219216299777112361E-13, -45.64921306006598201 ) ) ;
#130776=DIRECTION ( 'NONE',  ( 1.000000000000000000, 0.000000000000000000, 0.000000000000000000 ) ) ;
#130796=VERTEX_POINT ( 'NONE', #196364 ) ;
#130800=CARTESIAN_POINT ( 'NONE',  ( -38.00000000000000711, 2.428612866367529932E-14, -2.000000000000000000 ) ) ;
#130809=CARTESIAN_POINT ( 'NONE',  ( 29.21837264310193305, -26.94013878454481414, -20.44914777673364981 ) ) ;
#130830=ORIENTED_EDGE ( 'NONE', *, *, #131641, .F. ) ;
#130855=ORIENTED_EDGE ( 'NONE', *, *, #37807, .T. ) ;
#130861=CARTESIAN_POINT ( 'NONE',  ( -29.86685920354755197, -21.69954338932560134, -8.424999997268812990 ) ) ;
#130880=ADVANCED_FACE ( 'NONE', ( #121467, #148844 ), #103333, .T. ) ;
#130898=CARTESIAN_POINT ( 'NONE',  ( 31.49504140153652898, -1.029908246020218687, -49.63772645510939441 ) ) ;
#131014=DIRECTION ( 'NONE',  ( 1.000000000000000000, 0.000000000000000000, 0.000000000000000000 ) ) ;
#131036=CARTESIAN_POINT ( 'NONE',  ( 11.40812507854755253, -35.11059874428192273, -2.024999997268813079 ) ) ;
#131048=CARTESIAN_POINT ( 'NONE',  ( 0.000000000000000000, 0.000000000000000000, -61.89430850415821794 ) ) ;
#131057=CARTESIAN_POINT ( 'NONE',  ( 21.30000000000002913, -7.567280135845077329E-14, -58.85720012050612837 ) ) ;
#131095=CARTESIAN_POINT ( 'NONE',  ( -4.000000000000000888, -165.0000000000000000, -23.00000000000000000 ) ) ;
#131114=ORIENTED_EDGE ( 'NONE', *, *, #40503, .T. ) ;
#131188=CARTESIAN_POINT ( 'NONE',  ( -11.69745301899430956, -11.91991347263640222, -59.13370768023892055 ) ) ;
#131209=CARTESIAN_POINT ( 'NONE',  ( -11.74264578624800670, 36.14014761921585972, -2.149999994537626691 ) ) ;
#131226=CIRCLE ( 'NONE', #2054, 10.00000000000000000 ) ;
#131277=ADVANCED_FACE ( 'NONE', ( #154791 ), #16289, .T. ) ;
#131287=CARTESIAN_POINT ( 'NONE',  ( -30.74264578624800492, -22.33583958711396278, -7.549999994537627934 ) ) ;
#131300=CARTESIAN_POINT ( 'NONE',  ( 11.45643923738960446, -4.999999999999992895, -18.00000000000000000 ) ) ;
#131303=ORIENTED_EDGE ( 'NONE', *, *, #126809, .T. ) ;
#131319=AXIS2_PLACEMENT_3D ( 'NONE', #134490, #165822, #24318 ) ;
#131324=EDGE_CURVE ( 'NONE', #16960, #99783, #120134, .T. ) ;
#131337=CARTESIAN_POINT ( 'NONE',  ( -36.91746825000000598, 2.428612866367529932E-14, -5.124999997268813168 ) ) ;
#131338=CARTESIAN_POINT ( 'NONE',  ( -1.500431131851305500, -22.62413958104530920, -57.95367621771161737 ) ) ;
#131347=CARTESIAN_POINT ( 'NONE',  ( -28.47622644277399928, -25.16156846422451920, -16.68312038616162951 ) ) ;
#131359=CARTESIAN_POINT ( 'NONE',  ( -8.543935154431821388, -46.31530851242288804, -24.25021605108518941 ) ) ;
#131370=ORIENTED_EDGE ( 'NONE', *, *, #42762, .T. ) ;
#131372=CIRCLE ( 'NONE', #199217, 61.99999999999998579 ) ;
#131375=CARTESIAN_POINT ( 'NONE',  ( 21.31291730435230747, -0.2247805922399771505, -56.45983593933052447 ) ) ;
#131490=CARTESIAN_POINT ( 'NONE',  ( -15.60300394477387265, -17.53633401217249954, -57.38906433430459231 ) ) ;
#131493=CARTESIAN_POINT ( 'NONE',  ( -27.77250826529492755, -25.57832283906995130, -20.68473525701014992 ) ) ;
#131543=DIRECTION ( 'NONE',  ( 0.000000000000000000, 0.000000000000000000, -1.000000000000000000 ) ) ;
#131548=CARTESIAN_POINT ( 'NONE',  ( -9.248023074035629065, -10.74802307403544077, -60.25555373585994090 ) ) ;
#131562=CARTESIAN_POINT ( 'NONE',  ( -14.30620887846971279, 1.220661533321985903, -60.18359034246770989 ) ) ;
#131582=EDGE_LOOP ( 'NONE', ( #68840, #67801 ) ) ;
#131592=CARTESIAN_POINT ( 'NONE',  ( 37.99999999999999289, 2.893978650043524126E-14, -10.74999999453762811 ) ) ;
#131625=ORIENTED_EDGE ( 'NONE', *, *, #192484, .F. ) ;
#131641=EDGE_CURVE ( 'NONE', #150038, #140047, #24508, .T. ) ;
#131661=ORIENTED_EDGE ( 'NONE', *, *, #76859, .T. ) ;
#131670=EDGE_CURVE ( 'NONE', #93910, #194492, #46561, .T. ) ;
#131704=CARTESIAN_POINT ( 'NONE',  ( -30.20036327792369235, -26.22857331006468229, -17.18026671435357500 ) ) ;
#131754=EDGE_LOOP ( 'NONE', ( #176701, #114815, #82996 ) ) ;
#131764=CARTESIAN_POINT ( 'NONE',  ( -9.248023074035627289, -10.55727144485873126, -62.45740887555399468 ) ) ;
#131788=CARTESIAN_POINT ( 'NONE',  ( -29.87692619418718110, 1.408284774589867894, -48.43935853184042628 ) ) ;
#131795=CARTESIAN_POINT ( 'NONE',  ( 16.64782025964803225, -0.4052355915353793581, -59.15693706287429876 ) ) ;
#131797=DIRECTION ( 'NONE',  ( 0.000000000000000000, 0.000000000000000000, 1.000000000000000000 ) ) ;
#131799=DIRECTION ( 'NONE',  ( -5.204170427930421283E-16, 0.000000000000000000, -1.000000000000000000 ) ) ;
#131805=DIRECTION ( 'NONE',  ( -0.000000000000000000, -0.000000000000000000, 1.000000000000000000 ) ) ;
#131810=EDGE_LOOP ( 'NONE', ( #17474, #141367, #104940, #158105 ) ) ;
#131813=CARTESIAN_POINT ( 'NONE',  ( 37.99999999999999289, 2.893978650043524126E-14, -1.000000000000000000 ) ) ;
#131818=DIRECTION ( 'NONE',  ( 1.000000000000000000, 0.000000000000000000, 0.000000000000000000 ) ) ;
#131822=CARTESIAN_POINT ( 'NONE',  ( 29.51469970000643883, -26.64072072720820472, -20.60124869737700948 ) ) ;
#131842=ORIENTED_EDGE ( 'NONE', *, *, #172113, .T. ) ;
#131872=CARTESIAN_POINT ( 'NONE',  ( -22.81625015709509441, -31.40387420917324590, -6.324999997268815122 ) ) ;
#131929=AXIS2_PLACEMENT_3D ( 'NONE', #108728, #74430, #136097 ) ;
#132006=ORIENTED_EDGE ( 'NONE', *, *, #199554, .F. ) ;
#132024=CARTESIAN_POINT ( 'NONE',  ( 0.000000000000000000, 0.000000000000000000, -10.00000000000000000 ) ) ;
#132034=CARTESIAN_POINT ( 'NONE',  ( -33.40031027765337512, -22.02106105253704982, -24.45416078184958764 ) ) ;
#132045=CARTESIAN_POINT ( 'NONE',  ( 11.40812507854755253, -35.11059874428192273, -4.024999997268814411 ) ) ;
#132052=ORIENTED_EDGE ( 'NONE', *, *, #165213, .T. ) ;
#132056=FACE_OUTER_BOUND ( 'NONE', #93194, .T. ) ;
#132101=CARTESIAN_POINT ( 'NONE',  ( 28.90000000000002700, -0.1353689087803565394, -49.67367017693150189 ) ) ;
#132115=CARTESIAN_POINT ( 'NONE',  ( 15.85590801997753552, 17.61085972261885502, -57.22569728324523197 ) ) ;
#132194=CARTESIAN_POINT ( 'NONE',  ( -26.46959431505279881, -27.26463967846491698, -11.49588912907431393 ) ) ;
#132290=DIRECTION ( 'NONE',  ( 0.000000000000000000, 0.000000000000000000, 1.000000000000000000 ) ) ;
#132294=CARTESIAN_POINT ( 'NONE',  ( 38.00000000000000000, 12.34694845685046616, -8.649999994537624914 ) ) ;
#132307=CARTESIAN_POINT ( 'NONE',  ( -9.687362902255733488, 9.687362902255692632, -60.44446360152740993 ) ) ;
#132334=DIRECTION ( 'NONE',  ( -0.000000000000000000, -0.000000000000000000, 1.000000000000000000 ) ) ;
#132345=CARTESIAN_POINT ( 'NONE',  ( 36.91746824999999177, 2.880721459617395097E-14, -6.124999997268813168 ) ) ;
#132358=EDGE_CURVE ( 'NONE', #19818, #31363, #82020, .T. ) ;
#132368=CARTESIAN_POINT ( 'NONE',  ( -23.77862661291642610, -32.55609251395267734, -17.57696395782127752 ) ) ;
#132378=CARTESIAN_POINT ( 'NONE',  ( 9.455153793104345894, 11.51446144058595422, -62.12179458070791327 ) ) ;
#132383=CARTESIAN_POINT ( 'NONE',  ( -1.203296689329353519, -8.516692751257727068, -64.06477955746662190 ) ) ;
#132395=CARTESIAN_POINT ( 'NONE',  ( 0.000000000000000000, -105.0000000000000000, 5.497848452431111532 ) ) ;
#132498=DIRECTION ( 'NONE',  ( 0.000000000000000000, 0.000000000000000000, 1.000000000000000000 ) ) ;
#132501=CARTESIAN_POINT ( 'NONE',  ( -26.42731554605150635, -26.90581007260913537, -20.33945912742373707 ) ) ;
#132541=DIRECTION ( 'NONE',  ( -0.000000000000000000, -0.000000000000000000, -1.000000000000000000 ) ) ;
#132547=B_SPLINE_CURVE_WITH_KNOTS ( 'NONE', 3,
 ( #71604, #90738, #43264, #167604, #74597, #70611, #133270, #194961, #56438, #118119, #164623, #78550 ),
 .UNSPECIFIED., .F., .F.,
 ( 4, 2, 2, 2, 2, 4 ),
 ( 2.787091001330594030E-07, 0.0009290869694426631643, 0.001857895229785193293, 0.002786703490127723313, 0.003251107620298992334, 0.003715511750470261790 ),
 .UNSPECIFIED. ) ;
#132572=VERTEX_POINT ( 'NONE', #99026 ) ;
#132574=EDGE_CURVE ( 'NONE', #31363, #171664, #134200, .T. ) ;
#132586=ORIENTED_EDGE ( 'NONE', *, *, #13873, .F. ) ;
#132602=( BOUNDED_CURVE ( )  B_SPLINE_CURVE ( 2, ( #83749, #112116, #96928, #19122, #68589, #97907, #52426, #81744, #22099, #143431, #65608 ),
 .UNSPECIFIED., .F., .F. ) 
 B_SPLINE_CURVE_WITH_KNOTS ( ( 3, 2, 2, 2, 2, 3 ),
 ( 0.000000000000000000, 0.02000000000000000042, 0.04000000000000000083, 0.05999999999999999778, 0.08000000000000000167, 0.1000000000000000194 ),
 .UNSPECIFIED. ) 
 CURVE ( )  GEOMETRIC_REPRESENTATION_ITEM ( )  RATIONAL_B_SPLINE_CURVE ( ( 1.000000000000000000, 0.9510565162951535312, 1.000000000000000000, 0.9510565162951535312, 1.000000000000000000, 0.9510565162951535312, 1.000000000000000000, 0.9510565162951535312, 1.000000000000000000, 0.9510565162951535312, 1.000000000000000000 ) ) 
 REPRESENTATION_ITEM ( '' )  );
#132627=LINE ( 'NONE', #119463, #184630 ) ;
#132659=DIRECTION ( 'NONE',  ( 0.000000000000000000, 0.000000000000000000, 1.000000000000000000 ) ) ;
#132667=ADVANCED_FACE ( 'NONE', ( #145538 ), #174895, .F. ) ;
#132669=DIRECTION ( 'NONE',  ( 1.000000000000000000, 0.000000000000000000, 0.000000000000000000 ) ) ;
#132700=CARTESIAN_POINT ( 'NONE',  ( -23.48529157249599919, -32.32473071737749848, -3.449999994537626957 ) ) ;
#132706=CARTESIAN_POINT ( 'NONE',  ( -1.022580077288041090E-15, -16.70000000000002061, -64.92279855667830191 ) ) ;
#132751=EDGE_LOOP ( 'NONE', ( #174095, #152500, #43611, #69328, #13189, #24677 ) ) ;
#132760=CARTESIAN_POINT ( 'NONE',  ( 0.1264748200299367631, 28.90000000000004832, -52.65483682830182488 ) ) ;
#132778=DIRECTION ( 'NONE',  ( -0.000000000000000000, -0.000000000000000000, -1.000000000000000000 ) ) ;
#132780=CARTESIAN_POINT ( 'NONE',  ( 0.9976825729257744468, 8.724364686941823877, -61.97160884975856732 ) ) ;
#132809=CARTESIAN_POINT ( 'NONE',  ( -11.40812507854755609, 35.11059874428196537, -7.024999997268813523 ) ) ;
#132831=ORIENTED_EDGE ( 'NONE', *, *, #11291, .T. ) ;
#132834=LINE ( 'NONE', #103507, #76758 ) ;
#132867=CARTESIAN_POINT ( 'NONE',  ( -29.86685920354755552, 21.69954338932564397, -8.824999997268815122 ) ) ;
#132938=ORIENTED_EDGE ( 'NONE', *, *, #19810, .T. ) ;
#132949=DIRECTION ( 'NONE',  ( 1.000000000000000000, 0.000000000000000000, 0.000000000000000000 ) ) ;
#133011=EDGE_CURVE ( 'NONE', #100403, #116458, #29523, .T. ) ;
#133017=CARTESIAN_POINT ( 'NONE',  ( 0.000000000000000000, 0.000000000000000000, -64.92279855667830191 ) ) ;
#133026=CARTESIAN_POINT ( 'NONE',  ( -15.06137443927361019, -15.06137443927335440, -56.46919128290398504 ) ) ;
#133042=CARTESIAN_POINT ( 'NONE',  ( -22.81625015709510507, 31.40387420917330275, -2.924999997268813434 ) ) ;
#133052=CARTESIAN_POINT ( 'NONE',  ( 2.973862142520697471, -93.04182470242776049, -15.00000000000000178 ) ) ;
#133097=ORIENTED_EDGE ( 'NONE', *, *, #133150, .F. ) ;
#133112=CARTESIAN_POINT ( 'NONE',  ( 27.86273085795036408, -28.69962071417356242, -25.00000000000000000 ) ) ;
#133150=EDGE_CURVE ( 'NONE', #112132, #86619, #143815, .T. ) ;
#133174=SURFACE_STYLE_FILL_AREA ( #90650 ) ;
#133225=CYLINDRICAL_SURFACE ( 'NONE', #18142, 1.500000000000001332 ) ;
#133243=CARTESIAN_POINT ( 'NONE',  ( -21.74014569710914202, -31.09693755439675300, -22.87366378656648536 ) ) ;
#133262=DIRECTION ( 'NONE',  ( 1.000000000000000000, 0.000000000000000000, 0.000000000000000000 ) ) ;
#133270=CARTESIAN_POINT ( 'NONE',  ( 11.84747491945383224, -9.688819730466811109, -59.78303737067794543 ) ) ;
#133276=ORIENTED_EDGE ( 'NONE', *, *, #73153, .T. ) ;
#133282=CARTESIAN_POINT ( 'NONE',  ( 23.36741966814239646, -32.36690354120208468, -22.32433735814155540 ) ) ;
#133286=CARTESIAN_POINT ( 'NONE',  ( 3.766062262543149401E-15, -39.95556452105413570, -9.249999994537628112 ) ) ;
#133293=CARTESIAN_POINT ( 'NONE',  ( 6.874011537017776341, -5.374011537017756801, -61.98469907122333922 ) ) ;
#133337=CARTESIAN_POINT ( 'NONE',  ( 29.86685920354754842, -21.69954338932559068, -2.324999997268813345 ) ) ;
#133347=CARTESIAN_POINT ( 'NONE',  ( -9.687362902255733488, 9.687362902255692632, -65.00100000000003320 ) ) ;
#133360=CARTESIAN_POINT ( 'NONE',  ( -29.18329815487601664, -27.17471096552342402, -17.01306446741856249 ) ) ;
#133371=EDGE_LOOP ( 'NONE', ( #59937, #141744, #8522, #10295 ) ) ;
#133387=FACE_OUTER_BOUND ( 'NONE', #119908, .T. ) ;
#133388=DIRECTION ( 'NONE',  ( 1.000000000000000000, 0.000000000000000000, 0.000000000000000000 ) ) ;
#133491=CARTESIAN_POINT ( 'NONE',  ( -4.625078002628085549, 4.070616889113791714, -62.49731305256337066 ) ) ;
#133494=CARTESIAN_POINT ( 'NONE',  ( -19.96964676835922248, -32.33678545050552344, -24.48363814647542114 ) ) ;
#133496=CIRCLE ( 'NONE', #72154, 16.70000000000002061 ) ;
#133509=VERTEX_POINT ( 'NONE', #85871 ) ;
#133516=CARTESIAN_POINT ( 'NONE',  ( 13.99740082693655019, -37.19577201402442057, -29.83961662117126323 ) ) ;
#133563=CARTESIAN_POINT ( 'NONE',  ( 8.898962301217535398, -0.7565710328820663966, -63.99033069988504963 ) ) ;
#133615=EDGE_CURVE ( 'NONE', #48307, #106382, #171681, .T. ) ;
#133623=EDGE_CURVE ( 'NONE', #77704, #156506, #195550, .T. ) ;
#133626=ADVANCED_FACE ( 'NONE', ( #111735 ), #163194, .F. ) ;
#133633=AXIS2_PLACEMENT_3D ( 'NONE', #70133, #131805, #193484 ) ;
#133662=CARTESIAN_POINT ( 'NONE',  ( 1.490379145827383622, 7.404560491896994279, -64.28054250939490544 ) ) ;
#133681=DIRECTION ( 'NONE',  ( -0.000000000000000000, -0.000000000000000000, 1.000000000000000000 ) ) ;
#133698=CARTESIAN_POINT ( 'NONE',  ( 38.00000000000000000, -12.34694845685040754, -2.849999994537626424 ) ) ;
#133704=DIRECTION ( 'NONE',  ( -0.000000000000000000, -0.000000000000000000, 1.000000000000000000 ) ) ;
#133747=CARTESIAN_POINT ( 'NONE',  ( 9.100000000000001421, 0.000000000000000000, -63.95112321872120731 ) ) ;
#133754=CARTESIAN_POINT ( 'NONE',  ( -38.00000000000000711, 2.428612866367529932E-14, -4.000000000000000000 ) ) ;
#133772=AXIS2_PLACEMENT_3D ( 'NONE', #120605, #105444, #13437 ) ;
#133778=ORIENTED_EDGE ( 'NONE', *, *, #103351, .T. ) ;
#133785=EDGE_CURVE ( 'NONE', #29612, #120193, #7751, .T. ) ;
#133790=CARTESIAN_POINT ( 'NONE',  ( 17.51956405198879807, -15.55922825390971731, -57.41917273836692459 ) ) ;
#133793=CARTESIAN_POINT ( 'NONE',  ( 15.92681084339661268, -1.315686079477300874, -59.47631410104522587 ) ) ;
#133804=CARTESIAN_POINT ( 'NONE',  ( -3.503282210674349528, -48.86437366581481001, -23.00000000000000000 ) ) ;
#133814=CARTESIAN_POINT ( 'NONE',  ( 36.91746824999999177, 2.880721459617395097E-14, -9.624999997268814056 ) ) ;
#133819=FACE_OUTER_BOUND ( 'NONE', #25478, .T. ) ;
#133837=ORIENTED_EDGE ( 'NONE', *, *, #110611, .T. ) ;
#133869=AXIS2_PLACEMENT_3D ( 'NONE', #165978, #167952, #122429 ) ;
#133875=CARTESIAN_POINT ( 'NONE',  ( 29.86685920354754487, 21.69954338932564752, -7.424999997268813878 ) ) ;
#133964=AXIS2_PLACEMENT_3D ( 'NONE', #177822, #38297, #125575 ) ;
#133998=ORIENTED_EDGE ( 'NONE', *, *, #72679, .T. ) ;
#134026=CARTESIAN_POINT ( 'NONE',  ( -23.23284429171610910, -30.31406682163553867, -16.83429831496585649 ) ) ;
#134051=CARTESIAN_POINT ( 'NONE',  ( -11.40812507854754720, -35.11059874428192273, -10.22499999726881548 ) ) ;
#134074=DIRECTION ( 'NONE',  ( -0.000000000000000000, -0.000000000000000000, 1.000000000000000000 ) ) ;
#134099=VECTOR ( 'NONE', #41067, 1000.000000000000000 ) ;
#134114=CARTESIAN_POINT ( 'NONE',  ( 30.59399807301411656, -1.495846735942621297, -47.49088840515945265 ) ) ;
#134200=CIRCLE ( 'NONE', #34012, 40.00000000000000000 ) ;
#134268=CARTESIAN_POINT ( 'NONE',  ( 8.388830574159379737E-16, 13.70000000000001528, -60.44446360152740283 ) ) ;
#134296=ORIENTED_EDGE ( 'NONE', *, *, #80939, .F. ) ;
#134305=CARTESIAN_POINT ( 'NONE',  ( -30.74264578624800492, 22.33583958711400186, -5.949999994537626513 ) ) ;
#134311=CARTESIAN_POINT ( 'NONE',  ( 6.218960876731467913, -4.126125163602036849, -62.26018854728523166 ) ) ;
#134317=CARTESIAN_POINT ( 'NONE',  ( -12.24338688535747721, 10.51869806896807802, -59.40202214942380721 ) ) ;
#134321=CARTESIAN_POINT ( 'NONE',  ( -1.366177905283608052, -29.77433414031402137, -51.67655205196554391 ) ) ;
#134329=CARTESIAN_POINT ( 'NONE',  ( -24.24152472029835792, 0.4285070731210879891, -56.81472536503801507 ) ) ;
#134335=DIRECTION ( 'NONE',  ( -0.8660254037844391517, -0.000000000000000000, -0.4999999999999991673 ) ) ;
#134356=CARTESIAN_POINT ( 'NONE',  ( -22.81625015709510507, 31.40387420917330275, -3.424999997268813434 ) ) ;
#134365=CARTESIAN_POINT ( 'NONE',  ( 30.57569798415968876, -22.56501773984572168, -20.05394705607442063 ) ) ;
#134377=CARTESIAN_POINT ( 'NONE',  ( -30.85002141292116917, -24.92539791875024946, -19.32025355658407761 ) ) ;
#134378=ORIENTED_EDGE ( 'NONE', *, *, #130602, .T. ) ;
#134388=ORIENTED_EDGE ( 'NONE', *, *, #95674, .F. ) ;
#134393=CARTESIAN_POINT ( 'NONE',  ( -0.3916721525565259876, -9.051314012904525086, -63.96062167512636876 ) ) ;
#134408=B_SPLINE_CURVE_WITH_KNOTS ( 'NONE', 3,
 ( #179575, #41045, #102710, #195743, #42050, #103714, #27888, #89530, #165394, #26887, #88530, #151218 ),
 .UNSPECIFIED., .F., .F.,
 ( 4, 2, 2, 2, 2, 4 ),
 ( -6.183812803946990913E-05, 0.002421080454147832121, 0.004903999036335133718, 0.006145458327428788420, 0.007386917618522443121, 0.009869836200709747320 ),
 .UNSPECIFIED. ) ;
#134446=DIRECTION ( 'NONE',  ( -0.000000000000000000, -0.000000000000000000, 1.000000000000000000 ) ) ;
#134490=CARTESIAN_POINT ( 'NONE',  ( -3.573655867282028392E-15, 2.428612866367529932E-14, -23.00000000000000000 ) ) ;
#134509=CARTESIAN_POINT ( 'NONE',  ( 38.00000000000002842, 12.34694845685041109, -6.899999999999999467 ) ) ;
#134517=FACE_OUTER_BOUND ( 'NONE', #129580, .T. ) ;
#134548=ORIENTED_EDGE ( 'NONE', *, *, #139988, .F. ) ;
#134550=DIRECTION ( 'NONE',  ( -1.000000000000000000, -5.267352820763006950E-15, 0.000000000000000000 ) ) ;
#134558=CARTESIAN_POINT ( 'NONE',  ( 20.56805782000754590, 22.68575836265089762, -50.73663675503807013 ) ) ;
#134563=CARTESIAN_POINT ( 'NONE',  ( -10.00792592295668548, -12.06067447007310101, -59.61799893849534016 ) ) ;
#134580=CARTESIAN_POINT ( 'NONE',  ( 8.343164238912780917, -45.63112023308525522, -22.26988597240829293 ) ) ;
#134586=EDGE_LOOP ( 'NONE', ( #170526, #66616, #157534, #121661 ) ) ;
#134599=CARTESIAN_POINT ( 'NONE',  ( -69.65682714487590488, -71.74905178543390605, -15.00000000000000178 ) ) ;
#134603=CARTESIAN_POINT ( 'NONE',  ( -6.875025434611812258, 5.563988007711742512, -64.01045944195826110 ) ) ;
#134639=CYLINDRICAL_SURFACE ( 'NONE', #584, 1.500000000000001332 ) ;
#134670=FACE_OUTER_BOUND ( 'NONE', #181969, .T. ) ;
#134673=EDGE_LOOP ( 'NONE', ( #148696, #138619, #128220, #189824 ) ) ;
#134674=LINE ( 'NONE', #57828, #26944 ) ;
#134687=AXIS2_PLACEMENT_3D ( 'NONE', #24861, #39014, #161356 ) ;
#134692=ADVANCED_FACE ( 'NONE', ( #75853 ), #137529, .T. ) ;
#134694=EDGE_CURVE ( 'NONE', #42057, #120796, #102228, .T. ) ;
#134763=DIRECTION ( 'NONE',  ( -0.000000000000000000, -0.000000000000000000, 1.000000000000000000 ) ) ;
#134766=ORIENTED_EDGE ( 'NONE', *, *, #177434, .T. ) ;
#134791=DIRECTION ( 'NONE',  ( 1.000000000000000000, 0.000000000000000000, 0.000000000000000000 ) ) ;
#134794=EDGE_LOOP ( 'NONE', ( #119411, #144739, #188824, #33527, #121546, #132586, #196744, #129110 ) ) ;
#134827=CARTESIAN_POINT ( 'NONE',  ( -23.48529157249600985, 32.32473071737754111, -8.300000000000000711 ) ) ;
#134832=CARTESIAN_POINT ( 'NONE',  ( 1.151390856322186851, 16.16634691005189595, -59.37054012757567278 ) ) ;
#134886=CARTESIAN_POINT ( 'NONE',  ( -5.950531402560715689E-15, 38.81732327939063509, -7.124999997268814944 ) ) ;
#134890=CARTESIAN_POINT ( 'NONE',  ( 6.874011537017777229, -5.225174246120010579, -64.05724122177205970 ) ) ;
#134923=CARTESIAN_POINT ( 'NONE',  ( 0.000000000000000000, 0.000000000000000000, -61.89430850415821794 ) ) ;
#134931=CYLINDRICAL_SURFACE ( 'NONE', #172389, 40.00000000000000711 ) ;
#134940=EDGE_CURVE ( 'NONE', #60353, #185073, #40559, .T. ) ;
#134944=DIRECTION ( 'NONE',  ( -1.000000000000000000, 0.000000000000000000, -0.000000000000000000 ) ) ;
#134955=ORIENTED_EDGE ( 'NONE', *, *, #115825, .F. ) ;
#134972=AXIS2_PLACEMENT_3D ( 'NONE', #8493, #191505, #128819 ) ;
#134998=AXIS2_PLACEMENT_3D ( 'NONE', #22132, #84780, #113130 ) ;
#135011=EDGE_LOOP ( 'NONE', ( #11961, #22607, #130103, #104738 ) ) ;
#135024=VERTEX_POINT ( 'NONE', #118403 ) ;
#135037=CARTESIAN_POINT ( 'NONE',  ( -15.49673173449292563, -38.75597260390001964, -19.54956558032594671 ) ) ;
#135043=CARTESIAN_POINT ( 'NONE',  ( -14.76659222988139675, -15.47206428619941398, -58.80197253718059613 ) ) ;
#135062=CARTESIAN_POINT ( 'NONE',  ( 36.91746824999999887, -11.99521256947793546, -7.724999997268813701 ) ) ;
#135120=CARTESIAN_POINT ( 'NONE',  ( 31.88110949919180470, -0.2682394567895525772, -45.67705988491094615 ) ) ;
#135131=LINE ( 'NONE', #57286, #108949 ) ;
#135133=AXIS2_PLACEMENT_3D ( 'NONE', #27949, #155236, #540 ) ;
#135193=ORIENTED_EDGE ( 'NONE', *, *, #38432, .F. ) ;
#135199=EDGE_CURVE ( 'NONE', #42057, #76374, #176171, .T. ) ;
#135268=CARTESIAN_POINT ( 'NONE',  ( 37.99999999999999289, 2.428612866367529932E-14, -24.99999999999997868 ) ) ;
#135303=CARTESIAN_POINT ( 'NONE',  ( 37.99999999999999289, 2.893978650043524126E-14, -6.749999994537627224 ) ) ;
#135320=EDGE_CURVE ( 'NONE', #15137, #114628, #171850, .T. ) ;
#135328=CARTESIAN_POINT ( 'NONE',  ( -24.28797299941338039, 0.2180554607495331365, -56.78142080721297447 ) ) ;
#135355=CARTESIAN_POINT ( 'NONE',  ( -36.91746825000000598, -11.99521256947794789, -5.024999997268813523 ) ) ;
#135378=CARTESIAN_POINT ( 'NONE',  ( -26.35664240927071944, -29.91691629194321322, -17.00538226201434711 ) ) ;
#135379=EDGE_LOOP ( 'NONE', ( #169124, #165287 ) ) ;
#135393=CARTESIAN_POINT ( 'NONE',  ( -1.351053078614605107, -6.941067294099600105, -64.37011660792194334 ) ) ;
#135502=VECTOR ( 'NONE', #114479, 999.9999999999998863 ) ;
#135506=CARTESIAN_POINT ( 'NONE',  ( -6.875118674992797274, 5.563226388833924396, -61.95704554880759218 ) ) ;
#135559=EDGE_CURVE ( 'NONE', #164346, #138197, #53036, .T. ) ;
#135568=DIRECTION ( 'NONE',  ( 1.000000000000000000, 0.000000000000000000, 0.000000000000000000 ) ) ;
#135573=CARTESIAN_POINT ( 'NONE',  ( 21.25171708481321176, -32.43382446246057071, -17.33145006470355654 ) ) ;
#135578=ORIENTED_EDGE ( 'NONE', *, *, #184713, .F. ) ;
#135596=CARTESIAN_POINT ( 'NONE',  ( 0.000000000000000000, 0.000000000000000000, -10.00000000000000000 ) ) ;
#135661=DIRECTION ( 'NONE',  ( -0.000000000000000000, -0.000000000000000000, 1.000000000000000000 ) ) ;
#135664=ORIENTED_EDGE ( 'NONE', *, *, #95255, .T. ) ;
#135665=EDGE_LOOP ( 'NONE', ( #171162, #131625, #152428, #28022 ) ) ;
#135670=DIRECTION ( 'NONE',  ( 0.000000000000000000, 0.000000000000000000, 1.000000000000000000 ) ) ;
#135754=ORIENTED_EDGE ( 'NONE', *, *, #41891, .T. ) ;
#135790=CARTESIAN_POINT ( 'NONE',  ( -10.74802307403555268, 10.74802307403551715, -65.00100000000003320 ) ) ;
#135792=CARTESIAN_POINT ( 'NONE',  ( 16.22700747346227246, -14.59405422056926938, -58.52327065384329075 ) ) ;
#135795=CARTESIAN_POINT ( 'NONE',  ( -0.9928668394654698304, -21.65895526037597563, -56.20821996642036567 ) ) ;
#135797=CYLINDRICAL_SURFACE ( 'NONE', #77156, 2.500000000000000000 ) ;
#135805=DIRECTION ( 'NONE',  ( 0.000000000000000000, 0.000000000000000000, -1.000000000000000000 ) ) ;
#135814=CARTESIAN_POINT ( 'NONE',  ( 23.48529157249599919, 32.32473071737754111, -4.699999999999999289 ) ) ;
#135873=CARTESIAN_POINT ( 'NONE',  ( 5.686924398124309832, -3.878244659966709307, -64.40439148883940845 ) ) ;
#135992=ORIENTED_EDGE ( 'NONE', *, *, #20851, .F. ) ;
#136015=CARTESIAN_POINT ( 'NONE',  ( -25.80819889657188781, -27.69677943096050043, -16.54815200935615493 ) ) ;
#136038=CARTESIAN_POINT ( 'NONE',  ( -22.81625015709509441, -31.40387420917324590, -10.32499999726881157 ) ) ;
#136044=EDGE_LOOP ( 'NONE', ( #151224, #164713, #1807, #91019, #104598, #5394, #131842, #123527 ) ) ;
#136047=CYLINDRICAL_SURFACE ( 'NONE', #17061, 1.499999999999997780 ) ;
#136074=ORIENTED_EDGE ( 'NONE', *, *, #96295, .T. ) ;
#136097=DIRECTION ( 'NONE',  ( -1.000000000000000000, 0.000000000000000000, 0.000000000000000000 ) ) ;
#136280=CARTESIAN_POINT ( 'NONE',  ( 22.81625015709510151, -31.40387420917324590, -4.424999997268812990 ) ) ;
#136297=EDGE_CURVE ( 'NONE', #186567, #24637, #180996, .T. ) ;
#136298=LINE ( 'NONE', #78327, #118042 ) ;
#136305=DIRECTION ( 'NONE',  ( 1.000000000000000000, 0.000000000000000000, 0.000000000000000000 ) ) ;
#136321=CARTESIAN_POINT ( 'NONE',  ( -1.221313414957698099E-14, 31.90000000000003411, -49.13275782002545355 ) ) ;
#136353=CARTESIAN_POINT ( 'NONE',  ( -31.83877234781512655, -24.10177343596587107, -22.51708424455619451 ) ) ;
#136374=DIRECTION ( 'NONE',  ( -1.000000000000000000, 6.391086490440866478E-16, 0.000000000000000000 ) ) ;
#136416=DIRECTION ( 'NONE',  ( 0.000000000000000000, 0.000000000000000000, -1.000000000000000000 ) ) ;
#136436=CARTESIAN_POINT ( 'NONE',  ( -2.500000000000000000, 3.061616997868383141E-16, -65.00100000000003320 ) ) ;
#136461=EDGE_CURVE ( 'NONE', #89236, #140310, #147320, .T. ) ;
#136480=CARTESIAN_POINT ( 'NONE',  ( -20.85937581585705658, 20.13181022538182674, -49.56857446948050949 ) ) ;
#136498=DIRECTION ( 'NONE',  ( -1.000000000000000000, 0.000000000000000000, 0.000000000000000000 ) ) ;
#136524=CYLINDRICAL_SURFACE ( 'NONE', #170841, 38.00000000000000000 ) ;
#136566=VECTOR ( 'NONE', #160960, 1000.000000000000000 ) ;
#136629=DIRECTION ( 'NONE',  ( 1.000000000000000000, 0.000000000000000000, 0.000000000000000000 ) ) ;
#136645=DIRECTION ( 'NONE',  ( -1.000000000000000000, 0.000000000000000000, 0.000000000000000000 ) ) ;
#136647=EDGE_CURVE ( 'NONE', #24637, #44838, #166674, .T. ) ;
#136665=CARTESIAN_POINT ( 'NONE',  ( -3.573655867282028392E-15, 2.428612866367529932E-14, 0.000000000000000000 ) ) ;
#136671=CARTESIAN_POINT ( 'NONE',  ( -6.615299585309108110, 1.135848680322218751, -64.43295106733367561 ) ) ;
#136692=EDGE_CURVE ( 'NONE', #69503, #42366, #84623, .T. ) ;
#136721=EDGE_LOOP ( 'NONE', ( #71273, #131661, #94857, #121268 ) ) ;
#136722=CARTESIAN_POINT ( 'NONE',  ( 0.000000000000000000, 0.000000000000000000, -62.50719930893269805 ) ) ;
#136759=CARTESIAN_POINT ( 'NONE',  ( 18.70878831527338093, -37.83292004501380035, -19.76830273372893387 ) ) ;
#136761=DIRECTION ( 'NONE',  ( 0.000000000000000000, 0.000000000000000000, -1.000000000000000000 ) ) ;
#136764=CARTESIAN_POINT ( 'NONE',  ( -0.4379334789936237260, -21.36119649488922789, -56.42482690868973094 ) ) ;
#136783=CARTESIAN_POINT ( 'NONE',  ( 37.99999999999999289, 2.893978650043524126E-14, -5.000000000000000000 ) ) ;
#136799=VECTOR ( 'NONE', #48988, 1000.000000000000000 ) ;
#136801=DIRECTION ( 'NONE',  ( 1.000000000000000000, 0.000000000000000000, 0.000000000000000000 ) ) ;
#136810=ORIENTED_EDGE ( 'NONE', *, *, #53259, .T. ) ;
#136812=CARTESIAN_POINT ( 'NONE',  ( 2.662494480112517437, -37.13692398601924793, -32.60000000000000142 ) ) ;
#136816=ORIENTED_EDGE ( 'NONE', *, *, #131324, .T. ) ;
#136886=AXIS2_PLACEMENT_3D ( 'NONE', #182833, #44315, #56493 ) ;
#136902=CARTESIAN_POINT ( 'NONE',  ( 0.7993202289070840960, 31.67416946171545433, -49.41566550377648070 ) ) ;
#136977=CARTESIAN_POINT ( 'NONE',  ( -14.93382465614873666, -34.77343615282673994, -28.53315611748318759 ) ) ;
#136993=CARTESIAN_POINT ( 'NONE',  ( -7.776400214313161641, -46.08030136692367051, -22.42299576004354833 ) ) ;
#136999=AXIS2_PLACEMENT_3D ( 'NONE', #145946, #8448, #163128 ) ;
#137007=CARTESIAN_POINT ( 'NONE',  ( 6.874011537017776341, -5.374011537017756801, -61.98469907122333922 ) ) ;
#137015=CARTESIAN_POINT ( 'NONE',  ( 36.91746824999999177, 11.99521256947799230, -5.524999997268812635 ) ) ;
#137018=EDGE_CURVE ( 'NONE', #171133, #130796, #159583, .T. ) ;
#137034=CARTESIAN_POINT ( 'NONE',  ( 13.59403193627403539, -42.61206874333516481, -22.32444481402548675 ) ) ;
#137074=AXIS2_PLACEMENT_3D ( 'NONE', #128444, #99107, #4108 ) ;
#137080=VECTOR ( 'NONE', #90589, 1000.000000000000000 ) ;
#137152=ORIENTED_EDGE ( 'NONE', *, *, #188131, .F. ) ;
#137192=EDGE_CURVE ( 'NONE', #93735, #145198, #188966, .T. ) ;
#137220=COLOUR_RGB ( '', 0.31764706, 0.68627451, 0.89019608) ;
#137227=FACE_OUTER_BOUND ( 'NONE', #25368, .T. ) ;
#137229=DIRECTION ( 'NONE',  ( -0.000000000000000000, -0.000000000000000000, 1.000000000000000000 ) ) ;
#137245=FACE_BOUND ( 'NONE', #53676, .T. ) ;
#137251=CARTESIAN_POINT ( 'NONE',  ( -19.99604614807126524, -21.49604614807087799, -49.12629558063592583 ) ) ;
#137253=AXIS2_PLACEMENT_3D ( 'NONE', #162127, #179323, #23623 ) ;
#137263=ORIENTED_EDGE ( 'NONE', *, *, #110504, .T. ) ;
#137269=CARTESIAN_POINT ( 'NONE',  ( 36.91746825000000598, -11.99521256947793546, -4.224999997268812812 ) ) ;
#137318=CARTESIAN_POINT ( 'NONE',  ( 36.91746824999999177, 11.99521256947799230, -8.024999997268814411 ) ) ;
#137321=CARTESIAN_POINT ( 'NONE',  ( 1.242190437790102076, 23.66305621013599136, -57.22677643647746493 ) ) ;
#137351=AXIS2_PLACEMENT_3D ( 'NONE', #72654, #149485, #103979 ) ;
#137365=CARTESIAN_POINT ( 'NONE',  ( 7.405238625847253786, -1.490470117976223863, -64.28041130758167299 ) ) ;
#137370=AXIS2_PLACEMENT_3D ( 'NONE', #172896, #96035, #157722 ) ;
#137402=CARTESIAN_POINT ( 'NONE',  ( 1.022580077288041090E-15, 16.70000000000002061, -65.00100000000003320 ) ) ;
#137415=ADVANCED_FACE ( 'NONE', ( #129238 ), #144417, .F. ) ;
#137469=CARTESIAN_POINT ( 'NONE',  ( 1.285635531079530436, 29.62244251375079784, -48.76710130854527137 ) ) ;
#137487=CARTESIAN_POINT ( 'NONE',  ( -3.874011537017815421, -5.374011537017722162, -62.41807096325323556 ) ) ;
#137488=CARTESIAN_POINT ( 'NONE',  ( -6.856101608890801443E-16, -71.74905178543389184, -22.99263613531268291 ) ) ;
#137517=CARTESIAN_POINT ( 'NONE',  ( 9.100000000000001421, 0.000000000000000000, -61.89430850415821794 ) ) ;
#137529=CYLINDRICAL_SURFACE ( 'NONE', #4965, 28.90000000000004476 ) ;
#137534=AXIS2_PLACEMENT_3D ( 'NONE', #88262, #132778, #194465 ) ;
#137535=CARTESIAN_POINT ( 'NONE',  ( -5.362406601429247743, -6.881127002625603062, -64.03737582163388709 ) ) ;
#137559=DIRECTION ( 'NONE',  ( 0.000000000000000000, 0.000000000000000000, 1.000000000000000000 ) ) ;
#137572=VERTEX_POINT ( 'NONE', #130230 ) ;
#137625=CARTESIAN_POINT ( 'NONE',  ( 22.71484980649369945, -22.39856283320808217, -49.13275782002545355 ) ) ;
#137628=ORIENTED_EDGE ( 'NONE', *, *, #1893, .T. ) ;
#137633=DIRECTION ( 'NONE',  ( 1.000000000000000000, 0.000000000000000000, -0.000000000000000000 ) ) ;
#137670=EDGE_CURVE ( 'NONE', #188934, #113441, #197812, .T. ) ;
#137715=ORIENTED_EDGE ( 'NONE', *, *, #70168, .F. ) ;
#137718=ORIENTED_EDGE ( 'NONE', *, *, #187478, .T. ) ;
#137721=VERTEX_POINT ( 'NONE', #180781 ) ;
#137723=CARTESIAN_POINT ( 'NONE',  ( -38.00000000000000711, 2.428612866367529932E-14, -1.749999994537626558 ) ) ;
#137743=DIRECTION ( 'NONE',  ( -1.000000000000000000, 0.000000000000000000, 5.204170427930421283E-16 ) ) ;
#137754=DIRECTION ( 'NONE',  ( -0.000000000000000000, -0.000000000000000000, -1.000000000000000000 ) ) ;
#137760=DIRECTION ( 'NONE',  ( 0.000000000000000000, -1.000000000000000000, 0.000000000000000000 ) ) ;
#137766=CARTESIAN_POINT ( 'NONE',  ( 19.24578484527059175, -180.9428398739492820, -25.00000000000000000 ) ) ;
#137775=CARTESIAN_POINT ( 'NONE',  ( 3.766062262543149401E-15, -39.95556452105413570, -3.499999999999999556 ) ) ;
#137786=B_SPLINE_CURVE_WITH_KNOTS ( 'NONE', 3,
 ( #146826, #10331, #133662, #60534, #116495, #183901, #148841, #100317, #195352, #54821, #71987, #178184, #115501, #90868 ),
 .UNSPECIFIED., .F., .F.,
 ( 4, 2, 2, 2, 2, 2, 4 ),
 ( 0.002367542108447648688, 0.002663271933649134175, 0.002959001758850619661, 0.003254731584052104713, 0.003550461409253590200, 0.004141921059656562473, 0.004733380710059535181 ),
 .UNSPECIFIED. ) ;
#137803=CARTESIAN_POINT ( 'NONE',  ( 12.88217944815845684, -35.43691452638582717, -29.79217952741381836 ) ) ;
#137905=( BOUNDED_CURVE ( )  B_SPLINE_CURVE ( 2, ( #79899, #51550, #174903, #141570, #64735, #98021, #159716, #21213, #126397, #188093, #191066 ),
 .UNSPECIFIED., .F., .T. ) 
 B_SPLINE_CURVE_WITH_KNOTS ( ( 3, 2, 2, 2, 2, 3 ),
 ( 0.7000000000000001776, 0.7200000000000001954, 0.7400000000000001021, 0.7600000000000001199, 0.7800000000000000266, 0.8000000000000000444 ),
 .UNSPECIFIED. ) 
 CURVE ( )  GEOMETRIC_REPRESENTATION_ITEM ( )  RATIONAL_B_SPLINE_CURVE ( ( 0.9999999999999994449, 0.9510565162951540863, 1.000000000000000000, 0.9510565162951535312, 1.000000000000000000, 0.9510565162951535312, 1.000000000000000000, 0.9510565162951535312, 1.000000000000000000, 0.9510565162951535312, 1.000000000000000000 ) ) 
 REPRESENTATION_ITEM ( '' )  );
#137919=CARTESIAN_POINT ( 'NONE',  ( -21.74947994262150175, -22.98248435370785714, -49.47049204653305310 ) ) ;
#137944=ORIENTED_EDGE ( 'NONE', *, *, #115458, .T. ) ;
#137971=CARTESIAN_POINT ( 'NONE',  ( -23.65597376185835898, -29.51279439667934668, -21.31698521574488225 ) ) ;
#137977=ORIENTED_EDGE ( 'NONE', *, *, #20816, .T. ) ;
#137994=CARTESIAN_POINT ( 'NONE',  ( 20.85174543112844603, -20.13817253549177977, -49.56969272635731727 ) ) ;
#138012=CARTESIAN_POINT ( 'NONE',  ( -11.40812507854755609, 35.11059874428196537, -7.024999997268813523 ) ) ;
#138014=AXIS2_PLACEMENT_3D ( 'NONE', #171215, #138876, #45883 ) ;
#138024=DIRECTION ( 'NONE',  ( -0.000000000000000000, -0.000000000000000000, -1.000000000000000000 ) ) ;
#138033=B_SPLINE_CURVE_WITH_KNOTS ( 'NONE', 3,
 ( #40097, #24960, #26959, #88602, #119942, #164466, #25960 ),
 .UNSPECIFIED., .F., .F.,
 ( 4, 3, 4 ),
 ( -4.508036450095025827E-05, 0.000000000000000000, 0.006877813788783031929 ),
 .UNSPECIFIED. ) ;
#138118=CARTESIAN_POINT ( 'NONE',  ( -3.573655867282028392E-15, 2.428612866367529932E-14, -24.99999999999997868 ) ) ;
#138197=VERTEX_POINT ( 'NONE', #107866 ) ;
#138227=LINE ( 'NONE', #89738, #70145 ) ;
#138240=CARTESIAN_POINT ( 'NONE',  ( 0.1001742010324345455, 9.100000000000003197, -61.89430850415824636 ) ) ;
#138243=CARTESIAN_POINT ( 'NONE',  ( -9.656827144875922642, -71.74905178543390605, 0.000000000000000000 ) ) ;
#138249=CARTESIAN_POINT ( 'NONE',  ( -21.88302055210221297, -22.95674879174745087, -45.93240442770092358 ) ) ;
#138251=AXIS2_PLACEMENT_3D ( 'NONE', #167821, #105157, #29320 ) ;
#138265=CARTESIAN_POINT ( 'NONE',  ( -38.00000000000000711, 2.428612866367529932E-14, -11.74999999453762634 ) ) ;
#138277=CARTESIAN_POINT ( 'NONE',  ( 12.24802307403557577, -10.74802307403608737, -59.32879157176802920 ) ) ;
#138282=VECTOR ( 'NONE', #160441, 1000.000000000000000 ) ;
#138326=EDGE_CURVE ( 'NONE', #190734, #45261, #32044, .T. ) ;
#138331=VERTEX_POINT ( 'NONE', #91696 ) ;
#138338=EDGE_LOOP ( 'NONE', ( #196444, #69455, #85866, #95256 ) ) ;
#138357=CARTESIAN_POINT ( 'NONE',  ( 16.70000000000002061, 0.000000000000000000, -61.34707691135562868 ) ) ;
#138495=CARTESIAN_POINT ( 'NONE',  ( -9.051216217265920960, 0.3920586954752999786, -61.90435651123958394 ) ) ;
#138547=CARTESIAN_POINT ( 'NONE',  ( -6.502961151143344942, 4.381597987324907351, -64.22400872216478263 ) ) ;
#138560=ORIENTED_EDGE ( 'NONE', *, *, #72464, .F. ) ;
#138593=DIRECTION ( 'NONE',  ( 0.000000000000000000, 0.000000000000000000, -1.000000000000000000 ) ) ;
#138614=LINE ( 'NONE', #123434, #25846 ) ;
#138619=ORIENTED_EDGE ( 'NONE', *, *, #9338, .T. ) ;
#138725=ADVANCED_FACE ( 'NONE', ( #137227 ), #183743, .T. ) ;
#138741=DIRECTION ( 'NONE',  ( 1.000000000000000000, 0.000000000000000000, 0.000000000000000000 ) ) ;
#138745=CARTESIAN_POINT ( 'NONE',  ( 13.70000000000001528, 0.000000000000000000, -60.44446360152740283 ) ) ;
#138750=FACE_BOUND ( 'NONE', #150116, .T. ) ;
#138755=CARTESIAN_POINT ( 'NONE',  ( -17.41603567004575837, 15.34147874640864906, -57.57865799245708871 ) ) ;
#138765=CARTESIAN_POINT ( 'NONE',  ( -11.74264578624799782, -36.14014761921581709, -7.599999999999999645 ) ) ;
#138782=DIRECTION ( 'NONE',  ( -0.000000000000000000, -0.000000000000000000, 1.000000000000000000 ) ) ;
#138791=CARTESIAN_POINT ( 'NONE',  ( 17.48462780208548750, -33.70920939566803298, -26.63509803227954720 ) ) ;
#138796=ORIENTED_EDGE ( 'NONE', *, *, #96295, .F. ) ;
#138810=AXIS2_PLACEMENT_3D ( 'NONE', #5975, #39322, #116163 ) ;
#138817=EDGE_CURVE ( 'NONE', #172040, #39588, #86890, .T. ) ;
#138825=VERTEX_POINT ( 'NONE', #156373 ) ;
#138876=DIRECTION ( 'NONE',  ( -0.000000000000000000, -0.000000000000000000, 1.000000000000000000 ) ) ;
#138924=AXIS2_PLACEMENT_3D ( 'NONE', #85273, #131797, #144950 ) ;
#138940=VERTEX_POINT ( 'NONE', #109866 ) ;
#138956=CARTESIAN_POINT ( 'NONE',  ( -8.122171662652368340, -45.80197342711005604, -22.32604245071853555 ) ) ;
#138979=CARTESIAN_POINT ( 'NONE',  ( 37.99999999999999289, 2.893978650043524126E-14, -9.000000000000001776 ) ) ;
#139006=DIRECTION ( 'NONE',  ( 0.000000000000000000, 0.000000000000000000, 1.000000000000000000 ) ) ;
#139018=CARTESIAN_POINT ( 'NONE',  ( -11.57166747000293228, -12.01093693996313405, -61.35735997286332122 ) ) ;
#139086=EDGE_CURVE ( 'NONE', #161460, #130499, #5662, .T. ) ;
#139104=DIRECTION ( 'NONE',  ( 0.000000000000000000, 0.000000000000000000, 1.000000000000000000 ) ) ;
#139253=CARTESIAN_POINT ( 'NONE',  ( 3.766062262543149401E-15, -39.95556452105413570, -11.24999999453762278 ) ) ;
#139299=CARTESIAN_POINT ( 'NONE',  ( -38.00000000000000711, 2.893978650043524126E-14, -25.00000000000000000 ) ) ;
#139310=CARTESIAN_POINT ( 'NONE',  ( -9.760382078682885876, 9.614343725828547349, -62.58071313852360618 ) ) ;
#139325=EDGE_LOOP ( 'NONE', ( #49777, #40827, #10502, #121460 ) ) ;
#139383=CARTESIAN_POINT ( 'NONE',  ( -32.09281931051391012, -20.34824190692417289, -24.99999999999999289 ) ) ;
#139414=ORIENTED_EDGE ( 'NONE', *, *, #5777, .T. ) ;
#139442=CYLINDRICAL_SURFACE ( 'NONE', #122502, 216.0437394197456342 ) ;
#139446=CARTESIAN_POINT ( 'NONE',  ( 1.236971479055096745, 29.54649313627097840, -48.86402641782576239 ) ) ;
#139449=CARTESIAN_POINT ( 'NONE',  ( 6.835670873143622650, -5.764277696854612998, -61.93353089080586216 ) ) ;
#139464=CARTESIAN_POINT ( 'NONE',  ( -3.949974356353050720, -4.892573799038928861, -62.47626111183155473 ) ) ;
#139494=CARTESIAN_POINT ( 'NONE',  ( 24.30000000000003268, 0.000000000000000000, -56.77278709839600879 ) ) ;
#139541=CARTESIAN_POINT ( 'NONE',  ( -29.09442113371788352, -27.25731168736310295, -16.99878707713624948 ) ) ;
#139546=CYLINDRICAL_SURFACE ( 'NONE', #169699, 214.0437394197456911 ) ;
#139549=ORIENTED_EDGE ( 'NONE', *, *, #102120, .F. ) ;
#139580=CARTESIAN_POINT ( 'NONE',  ( -3.573655867282028392E-15, 2.428612866367529932E-14, -25.00000000000000000 ) ) ;
#139631=CARTESIAN_POINT ( 'NONE',  ( -38.00000000000000711, 12.34694845685046438, -3.849999994537626424 ) ) ;
#139641=DIRECTION ( 'NONE',  ( 0.000000000000000000, 0.000000000000000000, 1.000000000000000000 ) ) ;
#139728=CARTESIAN_POINT ( 'NONE',  ( -4.072063699643443613, -4.622657777628663922, -64.52289142388788434 ) ) ;
#139738=CARTESIAN_POINT ( 'NONE',  ( -17.60164288208769889, 16.44579809102482670, -56.93377352129066082 ) ) ;
#139743=EDGE_CURVE ( 'NONE', #149545, #45716, #140212, .T. ) ;
#139759=EDGE_CURVE ( 'NONE', #178146, #85226, #105089, .T. ) ;
#139774=CARTESIAN_POINT ( 'NONE',  ( 14.93382465614801902, -34.77343615282724443, -28.53315611748132241 ) ) ;
#139804=CARTESIAN_POINT ( 'NONE',  ( 3.556970738554033499E-15, -38.81732327939057825, -10.12499999726881228 ) ) ;
#139839=CARTESIAN_POINT ( 'NONE',  ( -69.65682714487590488, -71.74905178543390605, -15.00000000000000178 ) ) ;
#139842=CARTESIAN_POINT ( 'NONE',  ( 9.100000000000001421, 0.000000000000000000, -61.89430850415821794 ) ) ;
#139863=CARTESIAN_POINT ( 'NONE',  ( 15.06137443927350361, 15.06137443927346098, -56.46919128290398504 ) ) ;
#139887=CARTESIAN_POINT ( 'NONE',  ( -30.74264578624800492, -22.33583958711396278, -7.800000000000000711 ) ) ;
#139889=CARTESIAN_POINT ( 'NONE',  ( -19.99604614807123326, -21.65269601533040245, -52.04364612718746486 ) ) ;
#139940=EDGE_CURVE ( 'NONE', #23953, #63287, #11224, .T. ) ;
#139942=CARTESIAN_POINT ( 'NONE',  ( -14.16830335033896660, -40.16376294012538040, -20.11902964094489121 ) ) ;
#139968=CARTESIAN_POINT ( 'NONE',  ( 3.873560230149206252, 5.283393095647500814, -64.45999282322711110 ) ) ;
#139971=CARTESIAN_POINT ( 'NONE',  ( -31.90000000000003411, 3.219216299777112361E-13, -49.13275782002545355 ) ) ;
#139982=DIRECTION ( 'NONE',  ( -1.000000000000000000, 0.000000000000000000, 0.000000000000000000 ) ) ;
#139988=EDGE_CURVE ( 'NONE', #126376, #154964, #149603, .T. ) ;
#139989=VERTEX_POINT ( 'NONE', #196131 ) ;
#139992=CARTESIAN_POINT ( 'NONE',  ( -11.40812507854755609, 35.11059874428196537, -1.024999997268813301 ) ) ;
#140002=CARTESIAN_POINT ( 'NONE',  ( 22.96436041962737207, -32.42578188301177988, -19.82561655440861514 ) ) ;
#140004=CARTESIAN_POINT ( 'NONE',  ( -9.574954286947731319, -11.69376568609066958, -62.03511740007206043 ) ) ;
#140047=VERTEX_POINT ( 'NONE', #180954 ) ;
#140081=DIRECTION ( 'NONE',  ( 0.000000000000000000, 0.000000000000000000, 1.000000000000000000 ) ) ;
#140087=FACE_OUTER_BOUND ( 'NONE', #5778, .T. ) ;
#140125=CARTESIAN_POINT ( 'NONE',  ( 1.499999999999996891, 7.600000000000007638, -65.00100000000003320 ) ) ;
#140212=CIRCLE ( 'NONE', #111206, 2.500000000000000000 ) ;
#140225=CARTESIAN_POINT ( 'NONE',  ( -21.00974791550152432, -22.92140990621084384, -46.84590699842355832 ) ) ;
#140240=CARTESIAN_POINT ( 'NONE',  ( 30.74264578624800137, -22.33583958711395212, -10.94999999453762562 ) ) ;
#140241=AXIS2_PLACEMENT_3D ( 'NONE', #193594, #115745, #10573 ) ;
#140249=DIRECTION ( 'NONE',  ( 0.000000000000000000, 0.000000000000000000, 1.000000000000000000 ) ) ;
#140254=LINE ( 'NONE', #184782, #118830 ) ;
#140291=CARTESIAN_POINT ( 'NONE',  ( 11.40812507854754365, 35.11059874428196537, -9.724999997268813701 ) ) ;
#140293=CARTESIAN_POINT ( 'NONE',  ( 29.86685920354754842, -21.69954338932559068, -6.324999997268814234 ) ) ;
#140310=VERTEX_POINT ( 'NONE', #139383 ) ;
#140419=VECTOR ( 'NONE', #122185, 1000.000000000000000 ) ;
#140441=DIRECTION ( 'NONE',  ( 0.000000000000000000, 0.000000000000000000, 1.000000000000000000 ) ) ;
#140445=CARTESIAN_POINT ( 'NONE',  ( -22.47021661561681327, 20.34442274205735046, -47.91864530057669924 ) ) ;
#140447=CARTESIAN_POINT ( 'NONE',  ( -21.31291730435233234, 0.2247805922401949763, -56.45983593933052447 ) ) ;
#140483=AXIS2_PLACEMENT_3D ( 'NONE', #155267, #140081, #141085 ) ;
#140485=DIRECTION ( 'NONE',  ( -0.000000000000000000, 0.000000000000000000, 1.000000000000000000 ) ) ;
#140497=CARTESIAN_POINT ( 'NONE',  ( 22.98313974082799405, -1.499560036715175126, -57.70434786042491737 ) ) ;
#140535=AXIS2_PLACEMENT_3D ( 'NONE', #81266, #142947, #130776 ) ;
#140549=CARTESIAN_POINT ( 'NONE',  ( -31.90000000000003411, 3.219216299777112361E-13, -45.64921306006598201 ) ) ;
#140573=DIRECTION ( 'NONE',  ( 1.000000000000000000, 0.000000000000000000, 0.000000000000000000 ) ) ;
#140582=CARTESIAN_POINT ( 'NONE',  ( -13.74234921310041813, 0.4081324879002323769, -62.56359473395610138 ) ) ;
#140602=DIRECTION ( 'NONE',  ( 1.000000000000000000, 0.000000000000000000, 0.000000000000000000 ) ) ;
#140636=CARTESIAN_POINT ( 'NONE',  ( 37.99999999999999289, 2.893978650043524126E-14, -4.749999994537627224 ) ) ;
#140691=EDGE_CURVE ( 'NONE', #103031, #36560, #111040, .T. ) ;
#140696=ORIENTED_EDGE ( 'NONE', *, *, #183353, .F. ) ;
#140706=AXIS2_PLACEMENT_3D ( 'NONE', #68608, #190968, #130265 ) ;
#140734=CARTESIAN_POINT ( 'NONE',  ( 22.97079825734836689, -21.83149972758499402, -45.97092040041037109 ) ) ;
#140738=FACE_BOUND ( 'NONE', #53911, .T. ) ;
#140750=ORIENTED_EDGE ( 'NONE', *, *, #125272, .F. ) ;
#140776=CARTESIAN_POINT ( 'NONE',  ( 14.90098780496084885, -35.24605353401756247, -22.56189394118873892 ) ) ;
#140780=VERTEX_POINT ( 'NONE', #125225 ) ;
#140816=EDGE_CURVE ( 'NONE', #196237, #193343, #33218, .T. ) ;
#140835=AXIS2_PLACEMENT_3D ( 'NONE', #34229, #127209, #82692 ) ;
#140845=CARTESIAN_POINT ( 'NONE',  ( 6.100000000000006750, 0.000000000000000000, -62.50719930893269805 ) ) ;
#140889=AXIS2_PLACEMENT_3D ( 'NONE', #180348, #42814, #177342 ) ;
#140891=CARTESIAN_POINT ( 'NONE',  ( 9.333912919581869971, 11.25730316407965503, -60.07366171483953110 ) ) ;
#140893=CARTESIAN_POINT ( 'NONE',  ( 14.81572341150385341, 16.93990830356618460, -55.62237631978510422 ) ) ;
#140897=EDGE_CURVE ( 'NONE', #164148, #145515, #123215, .T. ) ;
#140931=VERTEX_POINT ( 'NONE', #80694 ) ;
#140935=VERTEX_POINT ( 'NONE', #107055 ) ;
#140946=CARTESIAN_POINT ( 'NONE',  ( -28.84224951681783367, -24.48020638810389826, -21.31946643861265400 ) ) ;
#140974=CARTESIAN_POINT ( 'NONE',  ( 0.000000000000000000, 0.000000000000000000, -15.00000000000000000 ) ) ;
#140985=DIRECTION ( 'NONE',  ( 0.000000000000000000, 0.000000000000000000, -1.000000000000000000 ) ) ;
#140995=CARTESIAN_POINT ( 'NONE',  ( -22.81625015709509441, -31.40387420917324590, -6.324999997268815122 ) ) ;
#141005=CARTESIAN_POINT ( 'NONE',  ( 24.61032826407981844, -31.32210114170771220, -21.33226357150231678 ) ) ;
#141025=ORIENTED_EDGE ( 'NONE', *, *, #8030, .F. ) ;
#141045=CARTESIAN_POINT ( 'NONE',  ( -0.1105695005018468569, -21.30000000000002558, -58.85720012050614969 ) ) ;
#141054=CARTESIAN_POINT ( 'NONE',  ( -14.62203461105329438, -16.42507781964516766, -55.99240808130958413 ) ) ;
#141058=CARTESIAN_POINT ( 'NONE',  ( 22.81625015709510151, -31.40387420917324590, -8.424999997268812990 ) ) ;
#141059=CARTESIAN_POINT ( 'NONE',  ( 37.99999999999999289, 12.34694845685046793, -2.649999994537626247 ) ) ;
#141085=DIRECTION ( 'NONE',  ( -1.000000000000000000, 0.000000000000000000, 0.000000000000000000 ) ) ;
#141123=EDGE_LOOP ( 'NONE', ( #49803, #109900, #156197, #83715 ) ) ;
#141182=AXIS2_PLACEMENT_3D ( 'NONE', #172566, #98682, #51204 ) ;
#141201=CARTESIAN_POINT ( 'NONE',  ( 30.74264578624800137, -22.33583958711395212, -5.200000000000001066 ) ) ;
#141220=FACE_BOUND ( 'NONE', #34809, .T. ) ;
#141226=CARTESIAN_POINT ( 'NONE',  ( -8.388830574159379737E-16, -13.70000000000001528, -62.58071313852362039 ) ) ;
#141237=DIRECTION ( 'NONE',  ( 0.000000000000000000, -0.000000000000000000, -1.000000000000000000 ) ) ;
#141238=B_SPLINE_CURVE_WITH_KNOTS ( 'NONE', 3,
 ( #8450, #70123, #193474, #131795, #54951, #163130, #24633, #86281, #147972, #133793, #108411, #122584, #58932, #170086, #12464, #31580, #199440, #44766, #106419, #90261, #182295, #104453, #166136, #138745 ),
 .UNSPECIFIED., .F., .F.,
 ( 4, 2, 2, 2, 2, 2, 2, 2, 2, 2, 2, 4 ),
 ( 1.970462153819272771E-07, 0.0003069708713090705718, 0.0006137446964027592957, 0.001227292346590132732, 0.001534066171683819233, 0.001840839996777505734, 0.002147613821871192236, 0.002454387646964878520, 0.003067935297152264533, 0.003681482947339650546, 0.004295030597527036559, 0.004908578247714422138 ),
 .UNSPECIFIED. ) ;
#141241=CARTESIAN_POINT ( 'NONE',  ( 29.86685920354754842, -21.69954338932559068, -8.324999997268813345 ) ) ;
#141277=DIRECTION ( 'NONE',  ( 1.000000000000000000, 0.000000000000000000, 0.000000000000000000 ) ) ;
#141290=CARTESIAN_POINT ( 'NONE',  ( 3.556970738554033499E-15, -38.81732327939057825, -4.624999997268814056 ) ) ;
#141298=CARTESIAN_POINT ( 'NONE',  ( -12.05108236997114446, 9.980772036771131894, -61.81300923031701444 ) ) ;
#141302=VECTOR ( 'NONE', #37292, 1000.000000000000000 ) ;
#141314=ORIENTED_EDGE ( 'NONE', *, *, #45175, .T. ) ;
#141326=CIRCLE ( 'NONE', #18633, 10.00000000000000178 ) ;
#141367=ORIENTED_EDGE ( 'NONE', *, *, #630, .F. ) ;
#141447=CARTESIAN_POINT ( 'NONE',  ( -21.65895526037597207, 0.9928668394656959828, -56.20821996642037988 ) ) ;
#141485=DIRECTION ( 'NONE',  ( -0.000000000000000000, -0.000000000000000000, 1.000000000000000000 ) ) ;
#141494=CARTESIAN_POINT ( 'NONE',  ( 24.11964846217548342, -0.7207009035786856588, -56.90195918390940477 ) ) ;
#141496=CARTESIAN_POINT ( 'NONE',  ( 23.31485601308175148, -29.82028178162995147, -21.55021174911959747 ) ) ;
#141516=ORIENTED_EDGE ( 'NONE', *, *, #142804, .T. ) ;
#141549=VERTEX_POINT ( 'NONE', #129175 ) ;
#141570=CARTESIAN_POINT ( 'NONE',  ( 23.48529157249600630, -32.32473071737748427, -9.049999994537627046 ) ) ;
#141580=CARTESIAN_POINT ( 'NONE',  ( -1.500046863536438568, -7.503800738396990688, -62.22166870076608092 ) ) ;
#141602=CARTESIAN_POINT ( 'NONE',  ( -9.687362902255733488, 9.687362902255692632, -60.44446360152740993 ) ) ;
#141616=CARTESIAN_POINT ( 'NONE',  ( -38.00000000000000711, 2.893978650043524126E-14, -25.00000000000000000 ) ) ;
#141644=CARTESIAN_POINT ( 'NONE',  ( -5.000000000000000888, 11.45643923738960090, -18.00000000000000000 ) ) ;
#141675=CARTESIAN_POINT ( 'NONE',  ( 30.40000000000003766, -9.573269184497053765E-14, -64.92279855667830191 ) ) ;
#141704=CARTESIAN_POINT ( 'NONE',  ( 0.7300717321527865344, 24.11456854404507411, -54.35927238525124494 ) ) ;
#141733=CARTESIAN_POINT ( 'NONE',  ( 17.32164067428065835, -17.02822768543988019, -56.78066529741710156 ) ) ;
#141744=ORIENTED_EDGE ( 'NONE', *, *, #170515, .F. ) ;
#141756=ORIENTED_EDGE ( 'NONE', *, *, #60885, .T. ) ;
#141769=CARTESIAN_POINT ( 'NONE',  ( 23.14280555631448877, -30.41650385747942664, -16.87365452858796999 ) ) ;
#141773=EDGE_LOOP ( 'NONE', ( #1289, #9329, #26682, #22663 ) ) ;
#141808=DIRECTION ( 'NONE',  ( -0.000000000000000000, -0.000000000000000000, 1.000000000000000000 ) ) ;
#141880=CYLINDRICAL_SURFACE ( 'NONE', #23657, 13.70000000000001528 ) ;
#141882=PLANE ( 'NONE',  #91606 ) ;
#141916=ORIENTED_EDGE ( 'NONE', *, *, #55568, .F. ) ;
#141921=FACE_OUTER_BOUND ( 'NONE', #63485, .T. ) ;
#141931=CARTESIAN_POINT ( 'NONE',  ( -28.40128899756798120, -24.57310642926549349, -18.78835905295398589 ) ) ;
#141943=AXIS2_PLACEMENT_3D ( 'NONE', #101313, #179194, #24509 ) ;
#141949=CYLINDRICAL_SURFACE ( 'NONE', #186043, 21.30000000000002913 ) ;
#141955=DIRECTION ( 'NONE',  ( 0.000000000000000000, 0.000000000000000000, 1.000000000000000000 ) ) ;
#141963=CARTESIAN_POINT ( 'NONE',  ( 22.63233124262814044, -20.50857827831517355, -50.83049096057695238 ) ) ;
#141972=CARTESIAN_POINT ( 'NONE',  ( -19.99999999999998224, -188.0000000000000000, -15.00000000000000178 ) ) ;
#141981=CARTESIAN_POINT ( 'NONE',  ( 29.86685920354754487, 21.69954338932564752, -3.424999997268813434 ) ) ;
#141991=CARTESIAN_POINT ( 'NONE',  ( 21.14397880779448968, -35.31393329058613517, -18.60109459635480889 ) ) ;
#142043=CARTESIAN_POINT ( 'NONE',  ( -22.81625015709510507, 31.40387420917330275, -0.9249999972688132122 ) ) ;
#142078=CARTESIAN_POINT ( 'NONE',  ( 31.67901979315914573, -0.7913989229878923837, -49.40962234820030829 ) ) ;
#142101=CARTESIAN_POINT ( 'NONE',  ( 0.000000000000000000, 0.000000000000000000, -25.00000000000000000 ) ) ;
#142110=VERTEX_POINT ( 'NONE', #41195 ) ;
#142207=CARTESIAN_POINT ( 'NONE',  ( 1.249015985346455970, 21.94700952099570301, -55.99705856128547765 ) ) ;
#142222=ORIENTED_EDGE ( 'NONE', *, *, #54562, .T. ) ;
#142230=CARTESIAN_POINT ( 'NONE',  ( 36.91746825000000598, -11.99521256947793546, -6.224999997268814589 ) ) ;
#142281=CARTESIAN_POINT ( 'NONE',  ( -5.950531402560715689E-15, 38.81732327939063509, -1.624999997268813612 ) ) ;
#142298=EDGE_LOOP ( 'NONE', ( #85899, #4763, #85138, #113941, #190686, #167976, #170866 ) ) ;
#142356=ORIENTED_EDGE ( 'NONE', *, *, #20816, .F. ) ;
#142436=CARTESIAN_POINT ( 'NONE',  ( -24.20415418211123537, 0.5379555815581192890, -54.28961862586981368 ) ) ;
#142453=CARTESIAN_POINT ( 'NONE',  ( -31.82351365011400901, 0.4884129450686308105, -49.22894560581806900 ) ) ;
#142470=CARTESIAN_POINT ( 'NONE',  ( -6.020228577223754586E-15, 39.95556452105416412, -6.249999994537626336 ) ) ;
#142472=CARTESIAN_POINT ( 'NONE',  ( -30.74264578624800492, 22.33583958711400186, -1.949999994537626735 ) ) ;
#142482=CARTESIAN_POINT ( 'NONE',  ( 24.20670376297029236, -0.5310992180246828509, -56.83968087238904587 ) ) ;
#142520=DIRECTION ( 'NONE',  ( 0.000000000000000000, -1.000000000000000000, 0.000000000000000000 ) ) ;
#142537=DIRECTION ( 'NONE',  ( -0.07151044867601363819, 0.9974398506828144884, 0.000000000000000000 ) ) ;
#142563=FACE_BOUND ( 'NONE', #179396, .T. ) ;
#142571=CARTESIAN_POINT ( 'NONE',  ( -1.452998035947202560, -7.215019197202739321, -62.28058590214430268 ) ) ;
#142594=CARTESIAN_POINT ( 'NONE',  ( -8.204442743001470362, -36.48291145135368652, -31.77125895174630443 ) ) ;
#142605=CARTESIAN_POINT ( 'NONE',  ( -5.511913701082267636, -6.874908499604756251, -61.96452946383318050 ) ) ;
#142684=ORIENTED_EDGE ( 'NONE', *, *, #3940, .F. ) ;
#142717=CARTESIAN_POINT ( 'NONE',  ( 27.44803035730394924, -28.83687526680896696, -16.92468093647911331 ) ) ;
#142718=LINE ( 'NONE', #52702, #21024 ) ;
#142729=CARTESIAN_POINT ( 'NONE',  ( -16.68934465457932603, 0.2055526423336037911, -59.13845350790285949 ) ) ;
#142762=CARTESIAN_POINT ( 'NONE',  ( 30.04893132686963853, -22.76590847478654211, -19.45433810172651334 ) ) ;
#142787=ORIENTED_EDGE ( 'NONE', *, *, #129491, .T. ) ;
#142804=EDGE_CURVE ( 'NONE', #140780, #9769, #193785, .T. ) ;
#142823=CARTESIAN_POINT ( 'NONE',  ( 20.43538597629128262, -20.43538597629122222, -52.65483682830183199 ) ) ;
#142828=CARTESIAN_POINT ( 'NONE',  ( 9.051216217265929842, -0.3920586954752088293, -61.90435651123959104 ) ) ;
#142839=CARTESIAN_POINT ( 'NONE',  ( -2.285367203649865752E-16, -64.83960026421343059, -23.00000000000000000 ) ) ;
#142873=CARTESIAN_POINT ( 'NONE',  ( -20.29110136410554333, -20.59644990402605558, -52.64180230391848170 ) ) ;
#142912=VERTEX_POINT ( 'NONE', #19129 ) ;
#142922=CARTESIAN_POINT ( 'NONE',  ( -31.20004872165591436, -21.37828431676506113, -20.08970689225503392 ) ) ;
#142947=DIRECTION ( 'NONE',  ( -0.000000000000000000, -0.000000000000000000, 1.000000000000000000 ) ) ;
#142953=CARTESIAN_POINT ( 'NONE',  ( 22.71303993882839833, -20.60981468104613512, -50.67862666510512781 ) ) ;
#142968=UNCERTAINTY_MEASURE_WITH_UNIT (LENGTH_MEASURE( 1.000000000000000082E-05 ), #28026, 'distance_accuracy_value', 'NONE');
#142971=CARTESIAN_POINT ( 'NONE',  ( 36.91746824999999177, 2.880721459617395097E-14, -1.624999997268813390 ) ) ;
#142981=CARTESIAN_POINT ( 'NONE',  ( 15.71981542752503103, -36.60361700297598730, -28.71911170260956681 ) ) ;
#143032=CARTESIAN_POINT ( 'NONE',  ( 3.556970738554033499E-15, -38.81732327939057825, -10.62499999726881050 ) ) ;
#143051=CARTESIAN_POINT ( 'NONE',  ( -0.7621229312825035240, -6.292920404648720378, -64.49503546857650349 ) ) ;
#143066=CARTESIAN_POINT ( 'NONE',  ( 30.09553654342099094, -1.478515647795636490, -51.30846887466859130 ) ) ;
#143133=AXIS2_PLACEMENT_3D ( 'NONE', #24897, #146206, #69376 ) ;
#143164=EDGE_LOOP ( 'NONE', ( #184229, #178599, #133778, #85608, #63865 ) ) ;
#143190=EDGE_CURVE ( 'NONE', #119352, #181556, #113104, .T. ) ;
#143208=ORIENTED_EDGE ( 'NONE', *, *, #4389, .T. ) ;
#143210=VERTEX_POINT ( 'NONE', #84754 ) ;
#143217=CARTESIAN_POINT ( 'NONE',  ( 29.86685920354754842, -21.69954338932559068, -6.324999997268814234 ) ) ;
#143263=CARTESIAN_POINT ( 'NONE',  ( 11.40812507854754365, 35.11059874428196537, -5.724999997268812812 ) ) ;
#143271=CARTESIAN_POINT ( 'NONE',  ( 5.883457575057182254, -36.84471599068518799, -32.38015766500865311 ) ) ;
#143275=CARTESIAN_POINT ( 'NONE',  ( 16.74109322108054343, 17.49235657833704138, -56.83968056806632774 ) ) ;
#143310=CARTESIAN_POINT ( 'NONE',  ( -7.656827144875921753, -71.74905178543390605, 0.000000000000000000 ) ) ;
#143321=ADVANCED_FACE ( 'NONE', ( #98925 ), #174795, .F. ) ;
#143410=CARTESIAN_POINT ( 'NONE',  ( 7.600000000000007638, -2.566789643721943520E-14, -64.92279855667830191 ) ) ;
#143431=CARTESIAN_POINT ( 'NONE',  ( 37.99999999999999289, 12.34694845685046793, -0.9000000000000000222 ) ) ;
#143434=CARTESIAN_POINT ( 'NONE',  ( -29.53952216915896400, 1.232294487434969499, -51.94279119241696918 ) ) ;
#143452=CARTESIAN_POINT ( 'NONE',  ( -23.48529157249600985, 32.32473071737754111, -4.049999994537626158 ) ) ;
#143487=VERTEX_POINT ( 'NONE', #40267 ) ;
#143502=CARTESIAN_POINT ( 'NONE',  ( -36.91746825000000598, 11.99521256947798520, -1.224999997268813257 ) ) ;
#143520=CARTESIAN_POINT ( 'NONE',  ( -17.43506102071591357, -39.09281690107973617, -20.41854293744172821 ) ) ;
#143542=CIRCLE ( 'NONE', #185570, 40.00000000000002132 ) ;
#143559=CARTESIAN_POINT ( 'NONE',  ( -1.425225664899842037, -7.122238460089386436, -62.29949481927936716 ) ) ;
#143583=CARTESIAN_POINT ( 'NONE',  ( -18.83841601638275520, -33.00795687112476173, -25.49111855720881792 ) ) ;
#143593=CARTESIAN_POINT ( 'NONE',  ( -6.434671708797631950, -6.434671708797536027, -61.89430850415821794 ) ) ;
#143629=EDGE_CURVE ( 'NONE', #161460, #93860, #101941, .T. ) ;
#143637=CIRCLE ( 'NONE', #14489, 31.90000000000003411 ) ;
#143687=CARTESIAN_POINT ( 'NONE',  ( 1.500000000001896261, 23.15496181198761150, -55.09642484015217434 ) ) ;
#143694=ORIENTED_EDGE ( 'NONE', *, *, #163998, .F. ) ;
#143724=CARTESIAN_POINT ( 'NONE',  ( -15.66521691804237015, 1.429200727443527663, -59.59145728475412795 ) ) ;
#143726=AXIS2_PLACEMENT_3D ( 'NONE', #125094, #157424, #60426 ) ;
#143732=ORIENTED_EDGE ( 'NONE', *, *, #110412, .F. ) ;
#143757=CARTESIAN_POINT ( 'NONE',  ( 37.02045864137332387, -17.72559658019842743, -19.07609595512616707 ) ) ;
#143785=CARTESIAN_POINT ( 'NONE',  ( -2.500000000000000000, -105.0000000000000000, 12.00000000000000355 ) ) ;
#143796=FACE_OUTER_BOUND ( 'NONE', #69703, .T. ) ;
#143815=CIRCLE ( 'NONE', #4526, 13.70000000000001528 ) ;
#143846=DIRECTION ( 'NONE',  ( 0.000000000000000000, 0.000000000000000000, 1.000000000000000000 ) ) ;
#143866=CARTESIAN_POINT ( 'NONE',  ( 6.100000000000006750, -2.167155344068307965E-14, -64.53213882399991519 ) ) ;
#143871=CARTESIAN_POINT ( 'NONE',  ( 23.48529157249600630, -32.32473071737748427, -7.299999999999998934 ) ) ;
#143915=AXIS2_PLACEMENT_3D ( 'NONE', #14575, #12613, #45905 ) ;
#143923=CARTESIAN_POINT ( 'NONE',  ( -26.91739389983944264, -26.09363094301675901, -18.46721497145169977 ) ) ;
#143939=ORIENTED_EDGE ( 'NONE', *, *, #79274, .T. ) ;
#143950=CARTESIAN_POINT ( 'NONE',  ( 4.381597987324926002, 6.502961151143325402, -64.22400872216481105 ) ) ;
#143956=CARTESIAN_POINT ( 'NONE',  ( 31.75360176573013860, -24.33155002292239288, -19.38334379417544184 ) ) ;
#143974=CARTESIAN_POINT ( 'NONE',  ( -29.86685920354755197, -21.69954338932560134, -2.424999997268813434 ) ) ;
#143984=CARTESIAN_POINT ( 'NONE',  ( 23.77862661291771929, -32.55609251395039649, -17.57696395782325283 ) ) ;
#143998=PLANE ( 'NONE',  #134972 ) ;
#144031=CARTESIAN_POINT ( 'NONE',  ( -16.62134038107351230, -17.54604082932918274, -54.32399035855149805 ) ) ;
#144034=CARTESIAN_POINT ( 'NONE',  ( 11.40812507854754365, 35.11059874428196537, -1.224999997268813479 ) ) ;
#144070=CARTESIAN_POINT ( 'NONE',  ( 28.97745891950394537, -0.4911207797135175301, -52.56957762865169315 ) ) ;
#144091=CYLINDRICAL_SURFACE ( 'NONE', #103472, 1.499999999999997780 ) ;
#144097=EDGE_CURVE ( 'NONE', #102970, #194207, #132547, .T. ) ;
#144150=DIRECTION ( 'NONE',  ( 0.000000000000000000, 0.000000000000000000, -1.000000000000000000 ) ) ;
#144179=CARTESIAN_POINT ( 'NONE',  ( 22.13519047554794739, 22.85886502250322039, -45.77314885760243612 ) ) ;
#144188=DIRECTION ( 'NONE',  ( -0.000000000000000000, -0.000000000000000000, -1.000000000000000000 ) ) ;
#144194=CARTESIAN_POINT ( 'NONE',  ( 1.204023950788500885, 8.515746792609135696, -62.01447643120975783 ) ) ;
#144205=CARTESIAN_POINT ( 'NONE',  ( 36.91746824999999887, -11.99521256947793546, -3.724999997268813257 ) ) ;
#144220=CARTESIAN_POINT ( 'NONE',  ( -29.86685920354755197, -21.69954338932560134, -6.924999997268813878 ) ) ;
#144263=CARTESIAN_POINT ( 'NONE',  ( 3.503282210674363295, -48.86437366581479580, -25.00000000000000000 ) ) ;
#144266=CARTESIAN_POINT ( 'NONE',  ( -5.950531402560715689E-15, 38.81732327939063509, -3.624999997268813168 ) ) ;
#144267=CARTESIAN_POINT ( 'NONE',  ( -22.99799039501310105, 21.44473182883388773, -49.72310555961293943 ) ) ;
#144277=CARTESIAN_POINT ( 'NONE',  ( 16.83584321579687781, 17.44568526726159874, -56.81531555676559009 ) ) ;
#144280=VERTEX_POINT ( 'NONE', #48238 ) ;
#144333=ADVANCED_FACE ( 'NONE', ( #106908 ), #184754, .F. ) ;
#144357=CARTESIAN_POINT ( 'NONE',  ( -19.99604614807126524, -21.49604614807087799, -52.16759353428663104 ) ) ;
#144413=CARTESIAN_POINT ( 'NONE',  ( -4.595912276383594453, -38.76652190272483267, -23.69787631201921840 ) ) ;
#144417=CYLINDRICAL_SURFACE ( 'NONE', #149916, 1.499999999999997780 ) ;
#144467=EDGE_CURVE ( 'NONE', #47952, #73471, #31194, .T. ) ;
#144469=CARTESIAN_POINT ( 'NONE',  ( -36.91746825000000598, 2.428612866367529932E-14, -1.124999997268813390 ) ) ;
#144485=VECTOR ( 'NONE', #19869, 1000.000000000000000 ) ;
#144505=DIRECTION ( 'NONE',  ( 1.000000000000000000, 0.000000000000000000, 0.000000000000000000 ) ) ;
#144518=ORIENTED_EDGE ( 'NONE', *, *, #173803, .T. ) ;
#144524=CARTESIAN_POINT ( 'NONE',  ( -16.41350681615411489, -36.34403388527378098, -28.23867313180392458 ) ) ;
#144540=EDGE_CURVE ( 'NONE', #185826, #60353, #67339, .T. ) ;
#144582=CARTESIAN_POINT ( 'NONE',  ( -11.30153831258472508, -180.0000000000000000, -15.00000000000000178 ) ) ;
#144674=EDGE_LOOP ( 'NONE', ( #73154, #123875, #145445, #57455, #96832 ) ) ;
#144708=CARTESIAN_POINT ( 'NONE',  ( 26.36902008128207697, -29.90370362120039971, -17.00062383490519835 ) ) ;
#144739=ORIENTED_EDGE ( 'NONE', *, *, #89447, .T. ) ;
#144746=VECTOR ( 'NONE', #73447, 1000.000000000000000 ) ;
#144755=CARTESIAN_POINT ( 'NONE',  ( 25.98457697381383369, -27.33515243881158341, -20.34861096990326246 ) ) ;
#144817=CARTESIAN_POINT ( 'NONE',  ( 16.70000000000002061, -5.933031843596843873E-14, -64.92279855667830191 ) ) ;
#144822=DIRECTION ( 'NONE',  ( 0.000000000000000000, 0.000000000000000000, 1.000000000000000000 ) ) ;
#144904=VERTEX_POINT ( 'NONE', #141226 ) ;
#144910=CARTESIAN_POINT ( 'NONE',  ( -21.23184647844206197, -181.1785498424364675, 0.000000000000000000 ) ) ;
#144917=ORIENTED_EDGE ( 'NONE', *, *, #101613, .T. ) ;
#144919=CARTESIAN_POINT ( 'NONE',  ( -24.94736998983943366, -28.55544918295244372, -16.60430580961714142 ) ) ;
#144945=DIRECTION ( 'NONE',  ( -0.000000000000000000, 0.000000000000000000, 1.000000000000000000 ) ) ;
#144950=DIRECTION ( 'NONE',  ( -1.000000000000000000, 0.000000000000000000, 0.000000000000000000 ) ) ;
#144962=ADVANCED_FACE ( 'NONE', ( #76574 ), #64394, .T. ) ;
#144967=CARTESIAN_POINT ( 'NONE',  ( 38.00000000000000711, -12.34694845685040754, -1.099999999999999645 ) ) ;
#144977=CARTESIAN_POINT ( 'NONE',  ( 33.88770617168000854, -21.25088722958024334, -25.15219191025233769 ) ) ;
#144997=ORIENTED_EDGE ( 'NONE', *, *, #78423, .T. ) ;
#145004=CARTESIAN_POINT ( 'NONE',  ( -2.973862142520655727, -93.04182470242767522, -15.00000000000000178 ) ) ;
#145024=EDGE_LOOP ( 'NONE', ( #18218, #86799, #85855, #78557 ) ) ;
#145026=CARTESIAN_POINT ( 'NONE',  ( -15.23006821330878502, -17.33560778597399477, -55.19189381068117228 ) ) ;
#145029=CARTESIAN_POINT ( 'NONE',  ( -29.86685920354755197, -21.69954338932560134, -2.424999997268813434 ) ) ;
#145063=DIRECTION ( 'NONE',  ( 1.000000000000000000, 6.391086490440868450E-16, 0.000000000000000000 ) ) ;
#145064=CARTESIAN_POINT ( 'NONE',  ( 28.91687668646898146, -0.2552802045322939972, -52.63629878241255255 ) ) ;
#145067=DIRECTION ( 'NONE',  ( 0.000000000000000000, 0.000000000000000000, -1.000000000000000000 ) ) ;
#145117=EDGE_CURVE ( 'NONE', #44838, #69503, #156690, .T. ) ;
#145144=ORIENTED_EDGE ( 'NONE', *, *, #42515, .T. ) ;
#145189=CARTESIAN_POINT ( 'NONE',  ( -28.30127546286004403, -27.84967942650712303, -20.15398247455540215 ) ) ;
#145198=VERTEX_POINT ( 'NONE', #177568 ) ;
#145200=CARTESIAN_POINT ( 'NONE',  ( 0.000000000000000000, 0.000000000000000000, -49.67367017693150189 ) ) ;
#145210=VERTEX_POINT ( 'NONE', #67365 ) ;
#145223=CARTESIAN_POINT ( 'NONE',  ( -19.99999999999998224, -190.0000000000000000, -15.00000000000000178 ) ) ;
#145235=EDGE_CURVE ( 'NONE', #46465, #104408, #95716, .T. ) ;
#145265=CARTESIAN_POINT ( 'NONE',  ( -22.45862007004993188, 20.33413869251830164, -51.11888769873471006 ) ) ;
#145315=EDGE_CURVE ( 'NONE', #148642, #57253, #192723, .T. ) ;
#145335=VERTEX_POINT ( 'NONE', #36029 ) ;
#145409=DIRECTION ( 'NONE',  ( 0.000000000000000000, 0.000000000000000000, 1.000000000000000000 ) ) ;
#145415=CARTESIAN_POINT ( 'NONE',  ( -0.4081324879000859940, -13.74234921310041280, -62.56359473395608717 ) ) ;
#145431=CARTESIAN_POINT ( 'NONE',  ( -29.39134536520996122, 1.114265510929974390, -52.10946600208640689 ) ) ;
#145438=VECTOR ( 'NONE', #8084, 1000.000000000000000 ) ;
#145445=ORIENTED_EDGE ( 'NONE', *, *, #136647, .T. ) ;
#145448=DIRECTION ( 'NONE',  ( 1.000000000000000000, 0.000000000000000000, 0.000000000000000000 ) ) ;
#145450=CARTESIAN_POINT ( 'NONE',  ( -38.00000000000000711, 2.428612866367529932E-14, -3.749999994537626780 ) ) ;
#145462=CARTESIAN_POINT ( 'NONE',  ( -21.30000000000002913, 2.244099063931684814E-13, -64.92279855667830191 ) ) ;
#145465=CARTESIAN_POINT ( 'NONE',  ( -0.8768460684518564197, -31.62105185743270397, -49.48175094143205399 ) ) ;
#145478=CARTESIAN_POINT ( 'NONE',  ( -19.99604614807126524, -21.49604614807087799, -49.12629558063592583 ) ) ;
#145501=CARTESIAN_POINT ( 'NONE',  ( -1.467328942210815335, -23.16108095314130466, -57.58004187413776265 ) ) ;
#145515=VERTEX_POINT ( 'NONE', #97678 ) ;
#145521=CARTESIAN_POINT ( 'NONE',  ( -10.05780954200478305, -38.14163830725842530, -31.65208490131487551 ) ) ;
#145522=AXIS2_PLACEMENT_3D ( 'NONE', #106415, #32571, #138741 ) ;
#145534=CARTESIAN_POINT ( 'NONE',  ( 9.980772036771176303, 12.05108236997111071, -61.81300923031701444 ) ) ;
#145538=FACE_OUTER_BOUND ( 'NONE', #125907, .T. ) ;
#145557=CARTESIAN_POINT ( 'NONE',  ( -3.573655867282028392E-15, 2.428612866367529932E-14, -18.00000000000000000 ) ) ;
#145595=LINE ( 'NONE', #7074, #197151 ) ;
#145688=CARTESIAN_POINT ( 'NONE',  ( 1.500000000000020872, 22.80000000000002913, -55.36297086913598520 ) ) ;
#145708=CYLINDRICAL_SURFACE ( 'NONE', #123965, 1.500000000000001332 ) ;
#145712=EDGE_CURVE ( 'NONE', #57684, #70174, #198557, .T. ) ;
#145723=CARTESIAN_POINT ( 'NONE',  ( -13.70000000000001528, 0.2077008434175769414, -60.44446360152740993 ) ) ;
#145730=ORIENTED_EDGE ( 'NONE', *, *, #60319, .F. ) ;
#145758=ORIENTED_EDGE ( 'NONE', *, *, #181804, .F. ) ;
#145835=EDGE_CURVE ( 'NONE', #58799, #137572, #93458, .T. ) ;
#145858=CARTESIAN_POINT ( 'NONE',  ( 22.99604614807110181, -21.49604614807104142, -49.67998909148434450 ) ) ;
#145907=EDGE_LOOP ( 'NONE', ( #86482, #145963, #69637, #177305 ) ) ;
#145908=DIRECTION ( 'NONE',  ( 0.000000000000000000, 0.000000000000000000, 1.000000000000000000 ) ) ;
#145918=DIRECTION ( 'NONE',  ( 0.000000000000000000, 0.000000000000000000, 1.000000000000000000 ) ) ;
#145923=CIRCLE ( 'NONE', #158763, 38.00000000000002132 ) ;
#145946=CARTESIAN_POINT ( 'NONE',  ( -69.65682714487590488, -71.74905178543390605, -15.00000000000000178 ) ) ;
#145963=ORIENTED_EDGE ( 'NONE', *, *, #5408, .T. ) ;
#145966=CARTESIAN_POINT ( 'NONE',  ( -23.48529157249599919, -32.32473071737750558, -1.699999999999999734 ) ) ;
#145976=CARTESIAN_POINT ( 'NONE',  ( 35.06017246933186726, -19.40171014085571954, -22.29041292151832820 ) ) ;
#145992=CARTESIAN_POINT ( 'NONE',  ( 1.022580077288041090E-15, 16.70000000000002061, -61.34707691135562868 ) ) ;
#146022=ORIENTED_EDGE ( 'NONE', *, *, #26122, .T. ) ;
#146027=CARTESIAN_POINT ( 'NONE',  ( 36.91746824999999887, 11.99521256947799053, -7.524999997268814411 ) ) ;
#146060=FACE_OUTER_BOUND ( 'NONE', #44268, .T. ) ;
#146061=CARTESIAN_POINT ( 'NONE',  ( 29.85394078251576744, -1.399641368455794899, -51.58569050288883062 ) ) ;
#146083=CARTESIAN_POINT ( 'NONE',  ( 20.41037832431316090, -34.40082058117813801, -24.99999999999991829 ) ) ;
#146158=ORIENTED_EDGE ( 'NONE', *, *, #124684, .T. ) ;
#146194=ORIENTED_EDGE ( 'NONE', *, *, #119036, .F. ) ;
#146204=ORIENTED_EDGE ( 'NONE', *, *, #6795, .F. ) ;
#146206=DIRECTION ( 'NONE',  ( -0.000000000000000000, -0.000000000000000000, 1.000000000000000000 ) ) ;
#146256=AXIS2_PLACEMENT_3D ( 'NONE', #49596, #78926, #140602 ) ;
#146258=CARTESIAN_POINT ( 'NONE',  ( 28.91886483090991433, -0.2690448904508166983, -49.65045026909250936 ) ) ;
#146272=CARTESIAN_POINT ( 'NONE',  ( 14.83455351965412561, 16.91340028822891384, -58.07447375877295315 ) ) ;
#146333=LINE ( 'NONE', #193869, #17727 ) ;
#146334=EDGE_CURVE ( 'NONE', #27708, #127799, #172944, .T. ) ;
#146427=CARTESIAN_POINT ( 'NONE',  ( -31.21487366219223603, 1.272595016298921244, -49.98150452412669154 ) ) ;
#146440=VERTEX_POINT ( 'NONE', #55149 ) ;
#146444=EDGE_CURVE ( 'NONE', #28673, #14377, #118115, .T. ) ;
#146445=CARTESIAN_POINT ( 'NONE',  ( 3.766062262543149401E-15, -39.95556452105413570, -7.249999994537627224 ) ) ;
#146453=CARTESIAN_POINT ( 'NONE',  ( -20.73749492396214933, -155.7167183371837496, -15.00000000000000178 ) ) ;
#146463=CARTESIAN_POINT ( 'NONE',  ( -0.8004727011103912604, -29.12650189376887866, -52.40478149256038165 ) ) ;
#146481=SPHERICAL_SURFACE ( 'NONE', #89240, 38.00000000000002132 ) ;
#146496=CARTESIAN_POINT ( 'NONE',  ( 3.556970738554034288E-15, -38.81732327939057114, -2.624999997268812724 ) ) ;
#146497=CARTESIAN_POINT ( 'NONE',  ( -0.1103568551766080236, -24.30000000000002913, -56.77278709839600168 ) ) ;
#146506=CARTESIAN_POINT ( 'NONE',  ( -1.297617798568277969, -29.64248797448947315, -48.74145669546047088 ) ) ;
#146520=EDGE_LOOP ( 'NONE', ( #113594, #60536, #129271, #171043 ) ) ;
#146545=DIRECTION ( 'NONE',  ( -0.000000000000000000, -0.000000000000000000, 1.000000000000000000 ) ) ;
#146611=ADVANCED_FACE ( 'NONE', ( #26788 ), #184425, .T. ) ;
#146625=AXIS2_PLACEMENT_3D ( 'NONE', #4841, #53349, #189888 ) ;
#146652=CYLINDRICAL_SURFACE ( 'NONE', #6300, 40.00000000000000000 ) ;
#146675=CARTESIAN_POINT ( 'NONE',  ( 9.441188956457336801, -38.26011958722975947, -31.87100816096936384 ) ) ;
#146693=ORIENTED_EDGE ( 'NONE', *, *, #194310, .F. ) ;
#146702=CARTESIAN_POINT ( 'NONE',  ( 20.70421334297370919, 22.78074831271776191, -50.54281738342969987 ) ) ;
#146707=CARTESIAN_POINT ( 'NONE',  ( -30.74264578624800492, 22.33583958711400186, -4.200000000000000178 ) ) ;
#146711=VECTOR ( 'NONE', #51184, 1000.000000000000000 ) ;
#146739=AXIS2_PLACEMENT_3D ( 'NONE', #187624, #62249, #45122 ) ;
#146757=CARTESIAN_POINT ( 'NONE',  ( 28.84224951681686377, -24.48020638810656280, -21.31946643862243462 ) ) ;
#146823=ADVANCED_FACE ( 'NONE', ( #199595 ), #5055, .T. ) ;
#146824=LINE ( 'NONE', #120469, #91544 ) ;
#146826=CARTESIAN_POINT ( 'NONE',  ( 1.500000000004810818, 7.599999999999482725, -64.24270632869257724 ) ) ;
#146829=CARTESIAN_POINT ( 'NONE',  ( -3.573655867282028392E-15, 2.428612866367529932E-14, -18.00000000000000000 ) ) ;
#146850=AXIS2_PLACEMENT_3D ( 'NONE', #113499, #143846, #111525 ) ;
#146860=ADVANCED_FACE ( 'NONE', ( #103619 ), #73293, .T. ) ;
#146876=AXIS2_PLACEMENT_3D ( 'NONE', #152421, #49229, #61396 ) ;
#146908=DIRECTION ( 'NONE',  ( 1.000000000000000000, 0.000000000000000000, 0.000000000000000000 ) ) ;
#146927=VECTOR ( 'NONE', #17645, 1000.000000000000000 ) ;
#146933=CARTESIAN_POINT ( 'NONE',  ( 1.473961946532198919, 30.07508824747824150, -51.33206735129527942 ) ) ;
#146944=B_SPLINE_CURVE_WITH_KNOTS ( 'NONE', 3,
 ( #182008, #172793, #110116, #18121, #186988, #157619, #173794, #51423 ),
 .UNSPECIFIED., .F., .F.,
 ( 4, 2, 2, 4 ),
 ( 2.787091001330594030E-07, 0.0002981295844663114534, 0.0005959804598324898710, 0.001191682210564843237 ),
 .UNSPECIFIED. ) ;
#146951=DIRECTION ( 'NONE',  ( -0.000000000000000000, -0.000000000000000000, 1.000000000000000000 ) ) ;
#146960=CARTESIAN_POINT ( 'NONE',  ( 37.99999999999996447, -12.34694845685046793, -6.849999994537626868 ) ) ;
#146969=VECTOR ( 'NONE', #101648, 1000.000000000000000 ) ;
#146978=ORIENTED_EDGE ( 'NONE', *, *, #97036, .T. ) ;
#146981=CARTESIAN_POINT ( 'NONE',  ( -23.48529157249600985, 32.32473071737754111, -2.299999999999999822 ) ) ;
#146999=LINE ( 'NONE', #178348, #40121 ) ;
#147004=ORIENTED_EDGE ( 'NONE', *, *, #100613, .T. ) ;
#147043=CARTESIAN_POINT ( 'NONE',  ( -36.91746825000001309, -11.99521256947794789, -4.524999997268813523 ) ) ;
#147057=CIRCLE ( 'NONE', #91736, 8.000000000000000000 ) ;
#147079=EDGE_CURVE ( 'NONE', #46465, #42359, #176274, .T. ) ;
#147081=DIRECTION ( 'NONE',  ( -0.000000000000000000, 0.000000000000000000, 1.000000000000000000 ) ) ;
#147190=ORIENTED_EDGE ( 'NONE', *, *, #68244, .T. ) ;
#147191=CARTESIAN_POINT ( 'NONE',  ( 21.71449870906583257, 22.98327899303666300, -46.07764953322298140 ) ) ;
#147205=CARTESIAN_POINT ( 'NONE',  ( -29.23421922662623373, -26.92455035691573073, -20.45761606001068245 ) ) ;
#147216=CARTESIAN_POINT ( 'NONE',  ( -11.40812507854754720, -35.11059874428192273, -4.224999997268813701 ) ) ;
#147226=CARTESIAN_POINT ( 'NONE',  ( -30.98568851139534530, -22.00224967906137863, -21.15899255711320492 ) ) ;
#147318=EDGE_CURVE ( 'NONE', #194492, #130499, #181464, .T. ) ;
#147320=B_SPLINE_CURVE_WITH_KNOTS ( 'NONE', 3,
 ( #42498, #133494, #27340, #69826, #9166, #178016, #120311, #88986, #182004, #116327, #43487, #132501, #71826, #105154, #8149, #117327, #131493, #179023, #102163, #163849, #195186, #56667, #180033, #30292 ),
 .UNSPECIFIED., .F., .F.,
 ( 4, 2, 2, 2, 2, 2, 2, 2, 2, 2, 2, 4 ),
 ( 0.01933719746734626627, 0.02187858767233087642, 0.02441997787731549352, 0.02696136808230011062, 0.02823206318479242263, 0.02950275828728473812, 0.03013810583853089586, 0.03077345338977705361, 0.03204414849226937256, 0.03458553869725403129, 0.03712692890223869002, 0.03966831910722334875 ),
 .UNSPECIFIED. ) ;
#147351=ORIENTED_EDGE ( 'NONE', *, *, #163221, .T. ) ;
#147409=CARTESIAN_POINT ( 'NONE',  ( -15.14060719587552128, 14.98214168267144508, -56.46919128290399215 ) ) ;
#147427=DIRECTION ( 'NONE',  ( -0.000000000000000000, -0.000000000000000000, -1.000000000000000000 ) ) ;
#147433=CARTESIAN_POINT ( 'NONE',  ( -0.5018587474792274294, -16.61713888009426299, -61.38171595447353468 ) ) ;
#147469=CARTESIAN_POINT ( 'NONE',  ( 23.48529157249600630, -32.32473071737749137, -5.049999994537627046 ) ) ;
#147476=CARTESIAN_POINT ( 'NONE',  ( 6.767139177214389179, -4.798834252846686077, -62.08368047933343803 ) ) ;
#147482=DIRECTION ( 'NONE',  ( 0.000000000000000000, 0.000000000000000000, 1.000000000000000000 ) ) ;
#147502=VECTOR ( 'NONE', #133704, 1000.000000000000000 ) ;
#147506=FACE_OUTER_BOUND ( 'NONE', #10269, .T. ) ;
#147518=EDGE_LOOP ( 'NONE', ( #40103, #8410, #51452, #36328 ) ) ;
#147520=AXIS2_PLACEMENT_3D ( 'NONE', #197183, #184971, #46456 ) ;
#147523=CARTESIAN_POINT ( 'NONE',  ( -36.91746825000000598, 11.99521256947798520, -5.224999997268812812 ) ) ;
#147533=CARTESIAN_POINT ( 'NONE',  ( -27.83212366386707615, -25.89052209088941225, -16.12745387078197012 ) ) ;
#147537=DIRECTION ( 'NONE',  ( -0.000000000000000000, -0.000000000000000000, 1.000000000000000000 ) ) ;
#147543=CARTESIAN_POINT ( 'NONE',  ( -25.01910340989286752, -31.27285607037816462, -17.23782325462181220 ) ) ;
#147554=CARTESIAN_POINT ( 'NONE',  ( 11.80868324581537543, 11.80868324581533990, -61.34707691135562868 ) ) ;
#147555=ORIENTED_EDGE ( 'NONE', *, *, #168309, .T. ) ;
#147560=CARTESIAN_POINT ( 'NONE',  ( -2.577820198429831642E-15, -9.100000000000001421, -63.95112321872120731 ) ) ;
#147567=CARTESIAN_POINT ( 'NONE',  ( 27.16368555717295763, -26.59078835260041629, -15.56371235017464727 ) ) ;
#147587=EDGE_LOOP ( 'NONE', ( #186664, #5177, #38837, #160908 ) ) ;
#147598=FACE_OUTER_BOUND ( 'NONE', #87792, .T. ) ;
#147656=CARTESIAN_POINT ( 'NONE',  ( 0.000000000000000000, 0.000000000000000000, -65.00100000000003320 ) ) ;
#147699=CARTESIAN_POINT ( 'NONE',  ( 11.02000550219334407, -37.94488912280207416, -31.28304700362889079 ) ) ;
#147730=CARTESIAN_POINT ( 'NONE',  ( 37.99999999999999289, 2.893978650043524126E-14, -5.000000000000000000 ) ) ;
#147737=CARTESIAN_POINT ( 'NONE',  ( -11.74264578624799782, -36.14014761921581709, -5.349999994537626868 ) ) ;
#147751=EDGE_LOOP ( 'NONE', ( #161993, #1179, #137715, #29388 ) ) ;
#147752=EDGE_CURVE ( 'NONE', #75168, #36560, #185946, .T. ) ;
#147775=FACE_OUTER_BOUND ( 'NONE', #20155, .T. ) ;
#147807=DIRECTION ( 'NONE',  ( -0.000000000000000000, 0.000000000000000000, 1.000000000000000000 ) ) ;
#147808=VERTEX_POINT ( 'NONE', #143866 ) ;
#147849=CARTESIAN_POINT ( 'NONE',  ( -3.573655867282028392E-15, 2.428612866367529932E-14, -25.00000000000000000 ) ) ;
#147889=DIRECTION ( 'NONE',  ( -0.1178549842436478201, -0.9930308165857339997, -0.000000000000000000 ) ) ;
#147928=ORIENTED_EDGE ( 'NONE', *, *, #62085, .F. ) ;
#147933=ORIENTED_EDGE ( 'NONE', *, *, #7594, .F. ) ;
#147942=CARTESIAN_POINT ( 'NONE',  ( 0.7923078531248324285, 29.12150355453722028, -52.41032305705210348 ) ) ;
#147962=CIRCLE ( 'NONE', #54418, 24.30000000000003268 ) ;
#147969=CARTESIAN_POINT ( 'NONE',  ( 17.23854840241255815, -15.08343195521229774, -57.79379418917771005 ) ) ;
#147970=CARTESIAN_POINT ( 'NONE',  ( -23.48529157249599919, -32.32473071737749848, -7.449999994537625625 ) ) ;
#147972=CARTESIAN_POINT ( 'NONE',  ( 16.08916976210840843, -1.211883243535162524, -59.40465844715060229 ) ) ;
#147974=CARTESIAN_POINT ( 'NONE',  ( 32.86279873472853552, -22.80822080465439328, -22.12545596063183240 ) ) ;
#147990=CARTESIAN_POINT ( 'NONE',  ( -5.950531402560715689E-15, 38.81732327939063509, -9.124999997268815832 ) ) ;
#147999=CARTESIAN_POINT ( 'NONE',  ( 37.91032098691110264, -19.19859865632790630, -20.09511994390771150 ) ) ;
#148000=LINE ( 'NONE', #24662, #37553 ) ;
#148015=CARTESIAN_POINT ( 'NONE',  ( 4.347827484049394897, -37.01609572857267239, -32.59999999895043743 ) ) ;
#148047=CARTESIAN_POINT ( 'NONE',  ( -36.91746825000001309, 11.99521256947798342, -6.724999997268813701 ) ) ;
#148080=DIRECTION ( 'NONE',  ( 0.000000000000000000, 0.000000000000000000, -1.000000000000000000 ) ) ;
#148107=CARTESIAN_POINT ( 'NONE',  ( -38.00000000000000711, 2.428612866367529932E-14, -7.749999994537626336 ) ) ;
#148195=CARTESIAN_POINT ( 'NONE',  ( 20.57406348593929479, 22.68986043004503372, -47.49330165217067901 ) ) ;
#148220=CARTESIAN_POINT ( 'NONE',  ( 3.556970738554034288E-15, -38.81732327939057114, -4.124999997268813168 ) ) ;
#148240=DIRECTION ( 'NONE',  ( 1.000000000000000000, 0.000000000000000000, 0.000000000000000000 ) ) ;
#148266=B_SPLINE_CURVE_WITH_KNOTS ( 'NONE', 3,
 ( #173811, #50460, #5921, #95951, #130248, #6914, #3931, #160612, #192956, #37262, #161609, #67598, #23103, #36257 ),
 .UNSPECIFIED., .F., .F.,
 ( 4, 2, 2, 2, 2, 2, 4 ),
 ( 2.784207231363245562E-07, 0.0005083736299775801996, 0.001016468839232024125, 0.002032659257740903301, 0.003048849676249782478, 0.003556944885504227487, 0.004065040094758672930 ),
 .UNSPECIFIED. ) ;
#148278=CARTESIAN_POINT ( 'NONE',  ( 29.56482114129866900, -1.249513161672083372, -48.84067647644820198 ) ) ;
#148295=ORIENTED_EDGE ( 'NONE', *, *, #39724, .T. ) ;
#148320=FACE_OUTER_BOUND ( 'NONE', #155233, .T. ) ;
#148332=AXIS2_PLACEMENT_3D ( 'NONE', #115748, #161245, #71243 ) ;
#148359=CIRCLE ( 'NONE', #151690, 61.99999999999998579 ) ;
#148405=CARTESIAN_POINT ( 'NONE',  ( -16.01221511231805650, 14.62261807015716997, -56.20577350945247019 ) ) ;
#148423=CARTESIAN_POINT ( 'NONE',  ( -14.77336750280015387, -39.52550427972444425, -19.86057791183451116 ) ) ;
#148429=CARTESIAN_POINT ( 'NONE',  ( -1.455575599910876816, -15.57446157010955012, -61.81477736546833057 ) ) ;
#148457=ORIENTED_EDGE ( 'NONE', *, *, #91512, .T. ) ;
#148467=CARTESIAN_POINT ( 'NONE',  ( 11.74264578624800315, -36.14014761921581709, -5.149999994537626691 ) ) ;
#148472=ADVANCED_FACE ( 'NONE', ( #190385 ), #21525, .F. ) ;
#148475=AXIS2_PLACEMENT_3D ( 'NONE', #146829, #51820, #68989 ) ;
#148502=CIRCLE ( 'NONE', #48483, 38.00000000000000000 ) ;
#148520=CARTESIAN_POINT ( 'NONE',  ( -22.81625015709509441, -31.40387420917324590, -4.824999997268813345 ) ) ;
#148521=CARTESIAN_POINT ( 'NONE',  ( -1.227931366032057224E-14, -24.30000000000003268, -56.77278709839600879 ) ) ;
#148536=ORIENTED_EDGE ( 'NONE', *, *, #24130, .T. ) ;
#148542=CARTESIAN_POINT ( 'NONE',  ( -27.28412861566019743, -28.99984389462718681, -16.93987563810431851 ) ) ;
#148556=CARTESIAN_POINT ( 'NONE',  ( -1.499903966022400947, -7.794767548047344619, -64.20498622968422353 ) ) ;
#148611=CIRCLE ( 'NONE', #71105, 6.100000000000006750 ) ;
#148642=VERTEX_POINT ( 'NONE', #145858 ) ;
#148678=CARTESIAN_POINT ( 'NONE',  ( 1.474428118389591535, 30.72100710653361233, -47.31857186563917850 ) ) ;
#148696=ORIENTED_EDGE ( 'NONE', *, *, #81756, .T. ) ;
#148699=DIRECTION ( 'NONE',  ( -1.000000000000000000, 0.000000000000000000, 0.000000000000000000 ) ) ;
#148719=DIRECTION ( 'NONE',  ( 0.000000000000000000, 0.000000000000000000, 1.000000000000000000 ) ) ;
#148723=DIRECTION ( 'NONE',  ( 0.000000000000000000, 0.000000000000000000, 1.000000000000000000 ) ) ;
#148744=CARTESIAN_POINT ( 'NONE',  ( 9.021937450273815884, -0.4877194249720462338, -63.96635223026898842 ) ) ;
#148801=EDGE_CURVE ( 'NONE', #119464, #89770, #86315, .T. ) ;
#148838=ORIENTED_EDGE ( 'NONE', *, *, #72845, .T. ) ;
#148839=LINE ( 'NONE', #166005, #117405 ) ;
#148841=CARTESIAN_POINT ( 'NONE',  ( 1.304474898271996253, 6.853129728370680240, -64.38708764409373941 ) ) ;
#148844=FACE_OUTER_BOUND ( 'NONE', #131582, .T. ) ;
#148960=CARTESIAN_POINT ( 'NONE',  ( 0.3921787546847190220, 9.051185887784736650, -61.90436275749404160 ) ) ;
#148974=ORIENTED_EDGE ( 'NONE', *, *, #192660, .F. ) ;
#148985=EDGE_LOOP ( 'NONE', ( #122324, #76659, #142684, #36987 ) ) ;
#148988=CARTESIAN_POINT ( 'NONE',  ( -22.81625015709509441, -31.40387420917324590, -8.324999997268815122 ) ) ;
#148994=CARTESIAN_POINT ( 'NONE',  ( 1.022580077288041090E-15, 16.70000000000002061, -59.13370768023891344 ) ) ;
#149016=CARTESIAN_POINT ( 'NONE',  ( 7.005188342142080415, -46.65430082754588170, -22.59844067006618573 ) ) ;
#149020=ORIENTED_EDGE ( 'NONE', *, *, #49003, .F. ) ;
#149049=CARTESIAN_POINT ( 'NONE',  ( -22.81625015709510507, 31.40387420917330275, -6.924999997268812990 ) ) ;
#149053=CARTESIAN_POINT ( 'NONE',  ( 4.313351365237961588, -4.313351365237934942, -64.53213882399992940 ) ) ;
#149078=FACE_OUTER_BOUND ( 'NONE', #132751, .T. ) ;
#149088=FACE_OUTER_BOUND ( 'NONE', #108797, .T. ) ;
#149170=ORIENTED_EDGE ( 'NONE', *, *, #28639, .T. ) ;
#149213=CARTESIAN_POINT ( 'NONE',  ( -26.05560406886080216, -30.01072603040635300, -20.45417971608944185 ) ) ;
#149223=CARTESIAN_POINT ( 'NONE',  ( 29.86685920354754842, -21.69954338932559068, -7.824999997268813345 ) ) ;
#149233=FACE_BOUND ( 'NONE', #90014, .T. ) ;
#149278=CARTESIAN_POINT ( 'NONE',  ( 29.41559601785650102, -1.135674102528286156, -49.03020479230155360 ) ) ;
#149302=ORIENTED_EDGE ( 'NONE', *, *, #87955, .T. ) ;
#149348=ORIENTED_EDGE ( 'NONE', *, *, #131670, .F. ) ;
#149391=EDGE_CURVE ( 'NONE', #16157, #87857, #150877, .T. ) ;
#149425=DIRECTION ( 'NONE',  ( 1.000000000000000000, 0.000000000000000000, 0.000000000000000000 ) ) ;
#149453=ORIENTED_EDGE ( 'NONE', *, *, #163221, .F. ) ;
#149461=CARTESIAN_POINT ( 'NONE',  ( -23.48529157249600985, 32.32473071737754111, -10.04999999453762705 ) ) ;
#149469=CARTESIAN_POINT ( 'NONE',  ( 2.577820198429831642E-15, 9.100000000000001421, -63.95112321872120731 ) ) ;
#149485=DIRECTION ( 'NONE',  ( -1.000000000000000000, -0.000000000000000000, -0.000000000000000000 ) ) ;
#149500=CARTESIAN_POINT ( 'NONE',  ( 20.73749492396215288, -155.7167183371838064, -15.00000000000000178 ) ) ;
#149510=CARTESIAN_POINT ( 'NONE',  ( 36.91746824999999177, 11.99521256947799230, -2.024999997268813523 ) ) ;
#149511=LINE ( 'NONE', #103005, #163727 ) ;
#149528=ORIENTED_EDGE ( 'NONE', *, *, #195188, .F. ) ;
#149534=CARTESIAN_POINT ( 'NONE',  ( -29.21837264310262228, -26.94013878454652300, -20.44914777674790685 ) ) ;
#149545=VERTEX_POINT ( 'NONE', #181223 ) ;
#149562=LINE ( 'NONE', #12070, #20684 ) ;
#149597=VECTOR ( 'NONE', #5301, 1000.000000000000000 ) ;
#149603=LINE ( 'NONE', #72776, #72558 ) ;
#149649=CARTESIAN_POINT ( 'NONE',  ( -38.00000000000000711, 2.428612866367529932E-14, -0.8749999972688132788 ) ) ;
#149670=CARTESIAN_POINT ( 'NONE',  ( 1.290379407950561275, 31.18582982555689753, -46.67606730179129215 ) ) ;
#149684=VERTEX_POINT ( 'NONE', #157819 ) ;
#149720=CARTESIAN_POINT ( 'NONE',  ( -9.248023074035634394, -11.04474067092430190, -60.16509628334827653 ) ) ;
#149736=CARTESIAN_POINT ( 'NONE',  ( 14.53388260107743868, -39.78846373132473957, -19.96647037889509946 ) ) ;
#149791=DIRECTION ( 'NONE',  ( -1.000000000000000000, 0.000000000000000000, 4.336808689942017736E-16 ) ) ;
#149831=ADVANCED_FACE ( 'NONE', ( #63816 ), #96130, .T. ) ;
#149834=LINE ( 'NONE', #199320, #57986 ) ;
#149860=CARTESIAN_POINT ( 'NONE',  ( 0.000000000000000000, 0.000000000000000000, -65.00100000000003320 ) ) ;
#149916=AXIS2_PLACEMENT_3D ( 'NONE', #157616, #112101, #80757 ) ;
#149935=EDGE_CURVE ( 'NONE', #112132, #171824, #111304, .T. ) ;
#149958=CARTESIAN_POINT ( 'NONE',  ( 17.02936912484732801, -14.89509079785907275, -57.98861440449752536 ) ) ;
#149977=ORIENTED_EDGE ( 'NONE', *, *, #97418, .F. ) ;
#149980=CARTESIAN_POINT ( 'NONE',  ( -38.00000000000000711, 2.428612866367529932E-14, -8.000000000000000000 ) ) ;
#149997=CARTESIAN_POINT ( 'NONE',  ( -3.573655867282028392E-15, 2.428612866367529932E-14, -25.00000000000000000 ) ) ;
#150015=EDGE_CURVE ( 'NONE', #176035, #71451, #46659, .T. ) ;
#150038=VERTEX_POINT ( 'NONE', #171991 ) ;
#150043=CARTESIAN_POINT ( 'NONE',  ( -29.86685920354755552, 21.69954338932564397, -6.824999997268814234 ) ) ;
#150047=CARTESIAN_POINT ( 'NONE',  ( 4.943711336861328576, -3.929442668020362017, -64.49862517692662323 ) ) ;
#150060=VECTOR ( 'NONE', #172726, 1000.000000000000000 ) ;
#150090=CIRCLE ( 'NONE', #172586, 206.0437394197456911 ) ;
#150098=( BOUNDED_CURVE ( )  B_SPLINE_CURVE ( 2, ( #17739, #13753, #62224, #63228, #122909, #170417, #45095, #106752, #31909, #93562, #78386 ),
 .UNSPECIFIED., .F., .T. ) 
 B_SPLINE_CURVE_WITH_KNOTS ( ( 3, 2, 2, 2, 2, 3 ),
 ( 0.2000000000000000111, 0.2200000000000000011, 0.2400000000000000189, 0.2600000000000000644, 0.2800000000000000822, 0.3000000000000000444 ),
 .UNSPECIFIED. ) 
 CURVE ( )  GEOMETRIC_REPRESENTATION_ITEM ( )  RATIONAL_B_SPLINE_CURVE ( ( 1.000000000000000000, 0.9510565162951535312, 1.000000000000000000, 0.9510565162951535312, 1.000000000000000000, 0.9510565162951535312, 1.000000000000000000, 0.9510565162951535312, 1.000000000000000000, 0.9510565162951534202, 1.000000000000000222 ) ) 
 REPRESENTATION_ITEM ( '' )  );
#150116=EDGE_LOOP ( 'NONE', ( #63532, #187837, #169641, #148838, #35799 ) ) ;
#150124=DIRECTION ( 'NONE',  ( 1.000000000000000000, 0.000000000000000000, 0.000000000000000000 ) ) ;
#150147=EDGE_CURVE ( 'NONE', #167327, #117002, #59929, .T. ) ;
#150161=EDGE_CURVE ( 'NONE', #71928, #1233, #47638, .T. ) ;
#150172=ORIENTED_EDGE ( 'NONE', *, *, #120340, .T. ) ;
#150187=EDGE_CURVE ( 'NONE', #70273, #106917, #15326, .T. ) ;
#150189=CIRCLE ( 'NONE', #62964, 2.500000000000000000 ) ;
#150200=CARTESIAN_POINT ( 'NONE',  ( -26.33511944008826688, -27.18111610334197081, -16.53814760372663173 ) ) ;
#150226=CARTESIAN_POINT ( 'NONE',  ( 11.40812507854754365, 35.11059874428196537, -7.224999997268813701 ) ) ;
#150240=AXIS2_PLACEMENT_3D ( 'NONE', #139839, #169193, #155027 ) ;
#150285=VERTEX_POINT ( 'NONE', #108318 ) ;
#150317=AXIS2_PLACEMENT_3D ( 'NONE', #49693, #1181, #155871 ) ;
#150361=ORIENTED_EDGE ( 'NONE', *, *, #4389, .F. ) ;
#150372=VECTOR ( 'NONE', #73898, 1000.000000000000000 ) ;
#150437=DIRECTION ( 'NONE',  ( -0.000000000000000000, -0.000000000000000000, 1.000000000000000000 ) ) ;
#150472=CARTESIAN_POINT ( 'NONE',  ( 38.00000000000000000, 12.34694845685046616, -4.649999994537627579 ) ) ;
#150478=CARTESIAN_POINT ( 'NONE',  ( 6.442991741790385696, -4.311730449243174945, -62.20106008945930398 ) ) ;
#150485=CARTESIAN_POINT ( 'NONE',  ( -12.25194888441104091, 10.91206588261560562, -59.27621954310795616 ) ) ;
#150522=CARTESIAN_POINT ( 'NONE',  ( 36.91746824999999887, -11.99521256947793546, -2.224999997268813701 ) ) ;
#150523=CARTESIAN_POINT ( 'NONE',  ( -1.304248841091933035E-15, -21.30000000000002913, -58.85720012050612837 ) ) ;
#150542=CARTESIAN_POINT ( 'NONE',  ( -23.38344545171685240, -32.96869167543736978, -17.70766473210117198 ) ) ;
#150554=ORIENTED_EDGE ( 'NONE', *, *, #11846, .T. ) ;
#150556=AXIS2_PLACEMENT_3D ( 'NONE', #116612, #146951, #67105 ) ;
#150601=AXIS2_PLACEMENT_3D ( 'NONE', #124605, #182326, #120629 ) ;
#150680=CARTESIAN_POINT ( 'NONE',  ( -11.30153831258471442, -180.0000000000000000, -25.00000000000000000 ) ) ;
#150689=EDGE_LOOP ( 'NONE', ( #5992, #91522, #172861, #115437 ) ) ;
#150736=DIRECTION ( 'NONE',  ( -0.000000000000000000, -0.000000000000000000, 1.000000000000000000 ) ) ;
#150741=CARTESIAN_POINT ( 'NONE',  ( -3.981139134329680029, -5.949693216777165006, -64.35446363059463692 ) ) ;
#150779=VERTEX_POINT ( 'NONE', #53619 ) ;
#150877=LINE ( 'NONE', #58841, #1906 ) ;
#150928=VERTEX_POINT ( 'NONE', #38458 ) ;
#150966=CARTESIAN_POINT ( 'NONE',  ( 0.000000000000000000, 0.000000000000000000, -45.64921306006598201 ) ) ;
#150969=CARTESIAN_POINT ( 'NONE',  ( -1.498759781556145754, -23.15940025311443407, -55.09305739490149989 ) ) ;
#150973=DIRECTION ( 'NONE',  ( -1.000000000000000000, 0.000000000000000000, 4.336808689942017736E-16 ) ) ;
#150979=DIRECTION ( 'NONE',  ( 1.000000000000000000, 0.000000000000000000, 0.000000000000000000 ) ) ;
#150981=AXIS2_PLACEMENT_3D ( 'NONE', #102779, #42121, #163462 ) ;
#150986=ORIENTED_EDGE ( 'NONE', *, *, #73257, .T. ) ;
#150989=CARTESIAN_POINT ( 'NONE',  ( 23.48529157249599919, 32.32473071737754111, -2.700000000000000622 ) ) ;
#151015=DIRECTION ( 'NONE',  ( 0.000000000000000000, 0.000000000000000000, -1.000000000000000000 ) ) ;
#151019=ORIENTED_EDGE ( 'NONE', *, *, #121441, .F. ) ;
#151078=DIRECTION ( 'NONE',  ( -0.000000000000000000, -0.000000000000000000, -1.000000000000000000 ) ) ;
#151157=VECTOR ( 'NONE', #159517, 1000.000000000000000 ) ;
#151218=CARTESIAN_POINT ( 'NONE',  ( -30.20036327792369235, -26.22857331006468229, -17.18026671435357500 ) ) ;
#151224=ORIENTED_EDGE ( 'NONE', *, *, #26654, .F. ) ;
#151235=CARTESIAN_POINT ( 'NONE',  ( 13.56018889279821771, -37.30201529093263701, -30.04439950253996017 ) ) ;
#151291=AXIS2_PLACEMENT_3D ( 'NONE', #159929, #194285, #55751 ) ;
#151453=ORIENTED_EDGE ( 'NONE', *, *, #21485, .T. ) ;
#151461=CARTESIAN_POINT ( 'NONE',  ( -5.950531402560715689E-15, 38.81732327939063509, -3.624999997268813168 ) ) ;
#151484=CARTESIAN_POINT ( 'NONE',  ( -22.62413958104530209, 1.500431131851542643, -57.95367621771161026 ) ) ;
#151499=DIRECTION ( 'NONE',  ( -0.000000000000000000, -0.000000000000000000, 1.000000000000000000 ) ) ;
#151510=CARTESIAN_POINT ( 'NONE',  ( -29.86685920354755197, -21.69954338932560134, -8.924999997268812990 ) ) ;
#151514=CIRCLE ( 'NONE', #125649, 9.100000000000001421 ) ;
#151524=EDGE_CURVE ( 'NONE', #140935, #93860, #95565, .T. ) ;
#151533=CARTESIAN_POINT ( 'NONE',  ( -22.96436041963305286, -32.42578188300798558, -19.82561655441343973 ) ) ;
#151560=CARTESIAN_POINT ( 'NONE',  ( 7.503727747132447057, -1.500047742438187059, -64.26135111332261829 ) ) ;
#151568=DIRECTION ( 'NONE',  ( -3.491481338843133355E-15, 0.000000000000000000, 1.000000000000000000 ) ) ;
#151594=DIRECTION ( 'NONE',  ( -0.000000000000000000, -0.000000000000000000, -1.000000000000000000 ) ) ;
#151657=CARTESIAN_POINT ( 'NONE',  ( -6.297279900606389980, 4.176031345420732954, -62.24169944404286525 ) ) ;
#151680=CARTESIAN_POINT ( 'NONE',  ( -2.260530480648137177E-15, -78.64506293871966136, -22.99999966871703094 ) ) ;
#151690=AXIS2_PLACEMENT_3D ( 'NONE', #69579, #147427, #189942 ) ;
#151708=CYLINDRICAL_SURFACE ( 'NONE', #50812, 1.499999999999996225 ) ;
#151731=EDGE_LOOP ( 'NONE', ( #153734, #94823, #46950, #181327 ) ) ;
#151821=DIRECTION ( 'NONE',  ( 1.000000000000000000, 0.000000000000000000, 0.000000000000000000 ) ) ;
#151828=DIRECTION ( 'NONE',  ( -1.000000000000000000, 0.000000000000000000, 0.000000000000000000 ) ) ;
#151845=CARTESIAN_POINT ( 'NONE',  ( 38.00000000000001421, 12.34694845685043951, -4.649999994537627579 ) ) ;
#151935=CARTESIAN_POINT ( 'NONE',  ( -22.55670631985108443, -22.55670631985069008, -45.64921306006598201 ) ) ;
#151948=DIRECTION ( 'NONE',  ( 0.000000000000000000, 0.000000000000000000, 1.000000000000000000 ) ) ;
#151963=CARTESIAN_POINT ( 'NONE',  ( -38.00000000000001421, 12.34694845685046438, -8.099999999999997868 ) ) ;
#151968=DIRECTION ( 'NONE',  ( 1.000000000000000000, 0.000000000000000000, 0.000000000000000000 ) ) ;
#151987=VERTEX_POINT ( 'NONE', #99469 ) ;
#151990=FACE_OUTER_BOUND ( 'NONE', #42989, .T. ) ;
#152016=ORIENTED_EDGE ( 'NONE', *, *, #47644, .F. ) ;
#152057=DIRECTION ( 'NONE',  ( -1.000000000000000000, 0.000000000000000000, 0.000000000000000000 ) ) ;
#152106=CARTESIAN_POINT ( 'NONE',  ( 14.64731493820428021, 16.60031353666870402, -55.88827192845551650 ) ) ;
#152144=ORIENTED_EDGE ( 'NONE', *, *, #172898, .T. ) ;
#152148=DIRECTION ( 'NONE',  ( -0.000000000000000000, 0.000000000000000000, 1.000000000000000000 ) ) ;
#152156=CARTESIAN_POINT ( 'NONE',  ( -9.524678007112646227, -44.64363251549263367, -21.91146642400208577 ) ) ;
#152186=CARTESIAN_POINT ( 'NONE',  ( 20.43538597629128262, -20.43538597629122222, -52.65483682830183199 ) ) ;
#152195=CARTESIAN_POINT ( 'NONE',  ( 36.91746824999999887, -11.99521256947793546, -9.724999997268813701 ) ) ;
#152213=CARTESIAN_POINT ( 'NONE',  ( 7.905529020989565225, -46.70198807554292841, -24.42054064165401428 ) ) ;
#152215=CARTESIAN_POINT ( 'NONE',  ( -9.338259190353433326, -11.33508666705209933, -62.20763404149727194 ) ) ;
#152268=DIRECTION ( 'NONE',  ( 1.000000000000000000, 6.391086490440868450E-16, 0.000000000000000000 ) ) ;
#152270=EDGE_CURVE ( 'NONE', #6817, #154699, #108568, .T. ) ;
#152399=CARTESIAN_POINT ( 'NONE',  ( 6.874011537017776341, -5.374011537017756801, -64.92279855667830191 ) ) ;
#152415=CARTESIAN_POINT ( 'NONE',  ( -0.9487569900773351605, -16.37811251030164073, -59.27680374464308244 ) ) ;
#152421=CARTESIAN_POINT ( 'NONE',  ( 0.000000000000000000, 0.000000000000000000, -64.92279855667830191 ) ) ;
#152428=ORIENTED_EDGE ( 'NONE', *, *, #111893, .T. ) ;
#152430=VERTEX_POINT ( 'NONE', #56983 ) ;
#152432=ADVANCED_FACE ( 'NONE', ( #133819 ), #103484, .T. ) ;
#152437=CARTESIAN_POINT ( 'NONE',  ( -23.48529157249599919, -32.32473071737750558, -11.44999999453762385 ) ) ;
#152488=CARTESIAN_POINT ( 'NONE',  ( -36.91746825000000598, 2.428612866367529932E-14, -1.124999997268813390 ) ) ;
#152489=CARTESIAN_POINT ( 'NONE',  ( 0.2184195620311772945, 24.28793279613386957, -56.78144967823585887 ) ) ;
#152500=ORIENTED_EDGE ( 'NONE', *, *, #24668, .T. ) ;
#152570=DIRECTION ( 'NONE',  ( -0.000000000000000000, -0.000000000000000000, 1.000000000000000000 ) ) ;
#152623=EDGE_CURVE ( 'NONE', #85226, #114628, #13613, .T. ) ;
#152630=CARTESIAN_POINT ( 'NONE',  ( -5.577594645134348994, 3.875073520655145654, -62.38867879588715937 ) ) ;
#152634=CARTESIAN_POINT ( 'NONE',  ( -22.98327899303673405, 21.71449870906575796, -46.07764953322298140 ) ) ;
#152680=DIRECTION ( 'NONE',  ( -0.000000000000000000, -0.000000000000000000, 1.000000000000000000 ) ) ;
#152700=CARTESIAN_POINT ( 'NONE',  ( 12.56216403881617083, -41.81473846791988080, -20.79002063418672464 ) ) ;
#152759=CARTESIAN_POINT ( 'NONE',  ( 0.000000000000000000, 0.000000000000000000, -59.13370768023891344 ) ) ;
#152760=ORIENTED_EDGE ( 'NONE', *, *, #133785, .T. ) ;
#152770=CARTESIAN_POINT ( 'NONE',  ( 0.000000000000000000, 0.000000000000000000, -49.13275782002545355 ) ) ;
#152800=CARTESIAN_POINT ( 'NONE',  ( 11.30153831258470731, -188.0000000000000000, 0.000000000000000000 ) ) ;
#152812=CIRCLE ( 'NONE', #165845, 10.00000000000000355 ) ;
#152825=CARTESIAN_POINT ( 'NONE',  ( -23.48529157249600985, 32.32473071737754111, -4.049999994537626158 ) ) ;
#152831=CARTESIAN_POINT ( 'NONE',  ( -7.405238625847228917, 1.490470117976274045, -64.28041130758167299 ) ) ;
#152910=CARTESIAN_POINT ( 'NONE',  ( -1.227931366032057224E-14, -24.30000000000003268, -64.92279855667830191 ) ) ;
#152920=CARTESIAN_POINT ( 'NONE',  ( -0.2213677808126943147, -24.28759355007370857, -54.22458008397515528 ) ) ;
#152929=CARTESIAN_POINT ( 'NONE',  ( -15.06137443927351249, 15.06137443927345210, -58.85720012050612837 ) ) ;
#152938=CARTESIAN_POINT ( 'NONE',  ( 38.00000000000000711, -12.34694845685040754, -5.099999999999999645 ) ) ;
#152953=CIRCLE ( 'NONE', #23810, 31.90000000000003411 ) ;
#152964=CARTESIAN_POINT ( 'NONE',  ( 12.11826072627459183, -36.49684537641077497, -23.43927118307718160 ) ) ;
#152991=EDGE_LOOP ( 'NONE', ( #129837, #36863, #170379, #158953 ) ) ;
#152992=ORIENTED_EDGE ( 'NONE', *, *, #42515, .F. ) ;
#152996=CARTESIAN_POINT ( 'NONE',  ( 1.500000000000166533, 15.01069668396672618, -62.04687407567888613 ) ) ;
#153055=CARTESIAN_POINT ( 'NONE',  ( 0.2597368657414628190, 31.90000000000004121, -49.13275782002544645 ) ) ;
#153073=DIRECTION ( 'NONE',  ( -1.000000000000000000, 1.154084784954514691E-14, 0.000000000000000000 ) ) ;
#153081=CARTESIAN_POINT ( 'NONE',  ( -20.43538597629143538, -20.43538597629106945, -52.65483682830182488 ) ) ;
#153083=FACE_OUTER_BOUND ( 'NONE', #119822, .T. ) ;
#153117=ORIENTED_EDGE ( 'NONE', *, *, #23834, .F. ) ;
#153131=CARTESIAN_POINT ( 'NONE',  ( -21.54936698787217253, -30.95672727791941625, -19.59590204859394191 ) ) ;
#153154=VECTOR ( 'NONE', #24631, 1000.000000000000000 ) ;
#153155=CARTESIAN_POINT ( 'NONE',  ( 21.28441087011643162, -20.00855284718919336, -49.30314046027508113 ) ) ;
#153172=CARTESIAN_POINT ( 'NONE',  ( 22.81625015709510151, -31.40387420917324590, -5.924999997268812990 ) ) ;
#153182=LINE ( 'NONE', #166402, #30056 ) ;
#153190=DIRECTION ( 'NONE',  ( -0.000000000000000000, -0.000000000000000000, 1.000000000000000000 ) ) ;
#153273=DIRECTION ( 'NONE',  ( -0.000000000000000000, 0.000000000000000000, 1.000000000000000000 ) ) ;
#153280=DIRECTION ( 'NONE',  ( 1.000000000000000000, 0.000000000000000000, 0.000000000000000000 ) ) ;
#153311=ORIENTED_EDGE ( 'NONE', *, *, #117840, .T. ) ;
#153391=CARTESIAN_POINT ( 'NONE',  ( -4.999999999999996447, 5.000000000000003553, -15.00000000000000000 ) ) ;
#153408=FACE_BOUND ( 'NONE', #162272, .T. ) ;
#153431=CARTESIAN_POINT ( 'NONE',  ( 23.48529157249600630, -32.32473071737749137, -11.04999999453762527 ) ) ;
#153438=FACE_OUTER_BOUND ( 'NONE', #153876, .T. ) ;
#153458=AXIS2_PLACEMENT_3D ( 'NONE', #83572, #69417, #96745 ) ;
#153468=ADVANCED_FACE ( 'NONE', ( #182321 ), #92263, .F. ) ;
#153482=CARTESIAN_POINT ( 'NONE',  ( 0.7217796442344650565, 24.11907168720511407, -56.90237149053705679 ) ) ;
#153527=CARTESIAN_POINT ( 'NONE',  ( 7.121805330552581914, -1.425084765988108071, -64.33521149768084513 ) ) ;
#153595=EDGE_LOOP ( 'NONE', ( #1786, #61973, #175262, #192969, #137152 ) ) ;
#153602=ADVANCED_FACE ( 'NONE', ( #122607 ), #61920, .F. ) ;
#153605=CARTESIAN_POINT ( 'NONE',  ( 0.2002308779610947886, 6.100000000000010303, -62.50719930893269805 ) ) ;
#153633=DIRECTION ( 'NONE',  ( 1.000000000000000000, 0.000000000000000000, 0.000000000000000000 ) ) ;
#153668=CARTESIAN_POINT ( 'NONE',  ( -6.100000000000006750, 6.426762577456935076E-14, -62.50719930893269805 ) ) ;
#153678=CARTESIAN_POINT ( 'NONE',  ( 23.50300173439386242, -1.337618122189738967, -57.33987540012255835 ) ) ;
#153681=DIRECTION ( 'NONE',  ( -0.000000000000000000, -0.000000000000000000, 1.000000000000000000 ) ) ;
#153691=CARTESIAN_POINT ( 'NONE',  ( 1.499999999999999556, 15.20000000000001883, -65.00100000000003320 ) ) ;
#153702=ORIENTED_EDGE ( 'NONE', *, *, #1430, .F. ) ;
#153734=ORIENTED_EDGE ( 'NONE', *, *, #34928, .F. ) ;
#153759=ORIENTED_EDGE ( 'NONE', *, *, #14345, .T. ) ;
#153798=ADVANCED_FACE ( 'NONE', ( #70664 ), #84802, .F. ) ;
#153821=CARTESIAN_POINT ( 'NONE',  ( 4.999999999999999112, 5.000000000000000888, -15.00000000000000000 ) ) ;
#153828=CARTESIAN_POINT ( 'NONE',  ( -6.100000000000006750, 6.426762577456935076E-14, -64.53213882399991519 ) ) ;
#153876=EDGE_LOOP ( 'NONE', ( #23664, #108606, #65893 ) ) ;
#153893=TOROIDAL_SURFACE ( 'NONE', #111887, 69.99999999999998579, 8.000000000000000000 ) ;
#153897=ADVANCED_FACE ( 'NONE', ( #147506 ), #146481, .F. ) ;
#153912=DIRECTION ( 'NONE',  ( 1.000000000000000000, 0.000000000000000000, 0.000000000000000000 ) ) ;
#153918=CARTESIAN_POINT ( 'NONE',  ( 6.259396865588135128, -47.62116666102460272, -24.77619460540839214 ) ) ;
#153923=CARTESIAN_POINT ( 'NONE',  ( -4.180869859159739299, -4.459673755041124288, -64.53025741665265969 ) ) ;
#153942=CARTESIAN_POINT ( 'NONE',  ( 23.48529157249600630, -32.32473071737749137, -7.299999999999998934 ) ) ;
#153966=ORIENTED_EDGE ( 'NONE', *, *, #97744, .T. ) ;
#153968=CARTESIAN_POINT ( 'NONE',  ( 12.81081878836725707, -36.21111560917147898, -23.25335493478531745 ) ) ;
#153996=VERTEX_POINT ( 'NONE', #174843 ) ;
#154084=CARTESIAN_POINT ( 'NONE',  ( 15.84704938773726823, 17.60909914540862431, -54.71262039249373998 ) ) ;
#154124=EDGE_LOOP ( 'NONE', ( #112765, #98483, #147928, #172580 ) ) ;
#154131=AXIS2_PLACEMENT_3D ( 'NONE', #161215, #80379, #68198 ) ;
#154137=CARTESIAN_POINT ( 'NONE',  ( -18.67464278970884806, -33.09908666442120051, -25.63618526509586815 ) ) ;
#154157=CIRCLE ( 'NONE', #66964, 38.00000000000000711 ) ;
#154178=DIRECTION ( 'NONE',  ( -0.000000000000000000, -0.000000000000000000, -1.000000000000000000 ) ) ;
#154186=ORIENTED_EDGE ( 'NONE', *, *, #156407, .F. ) ;
#154189=FACE_OUTER_BOUND ( 'NONE', #33349, .T. ) ;
#154198=CARTESIAN_POINT ( 'NONE',  ( 7.765519415021292282, -39.80263117873665379, -25.57543461820742436 ) ) ;
#154276=DIRECTION ( 'NONE',  ( -0.8571673007021135549, 1.049727191138620175E-16, 0.5150380749100520461 ) ) ;
#154292=LINE ( 'NONE', #15782, #156223 ) ;
#154300=EDGE_CURVE ( 'NONE', #22413, #12839, #122129, .T. ) ;
#154389=CARTESIAN_POINT ( 'NONE',  ( 0.000000000000000000, 0.000000000000000000, -58.85720012050612837 ) ) ;
#154408=CARTESIAN_POINT ( 'NONE',  ( -0.4100021152176883121, -13.74275686049845291, -60.42614020214177373 ) ) ;
#154414=CARTESIAN_POINT ( 'NONE',  ( -20.66645964050063000, -22.75219995122948546, -47.34454927323474038 ) ) ;
#154423=EDGE_LOOP ( 'NONE', ( #83765, #185647, #7472, #87327 ) ) ;
#154429=CARTESIAN_POINT ( 'NONE',  ( -22.81625015709510507, 31.40387420917330275, -3.424999997268813434 ) ) ;
#154442=DIRECTION ( 'NONE',  ( -1.000000000000000000, 0.000000000000000000, 0.000000000000000000 ) ) ;
#154452=( BOUNDED_CURVE ( )  B_SPLINE_CURVE ( 2, ( #11371, #133698, #9368, #89182, #177226, #55856, #72025, #132700, #197373, #195390, #100355 ),
 .UNSPECIFIED., .F., .T. ) 
 B_SPLINE_CURVE_WITH_KNOTS ( ( 3, 2, 2, 2, 2, 3 ),
 ( 0.1000000000000000056, 0.1199999999999999956, 0.1400000000000000133, 0.1600000000000000033, 0.1799999999999999933, 0.2000000000000000111 ),
 .UNSPECIFIED. ) 
 CURVE ( )  GEOMETRIC_REPRESENTATION_ITEM ( )  RATIONAL_B_SPLINE_CURVE ( ( 1.000000000000000000, 0.9510565162951535312, 1.000000000000000000, 0.9510565162951535312, 1.000000000000000000, 0.9510565162951535312, 1.000000000000000000, 0.9510565162951535312, 1.000000000000000000, 0.9510565162951535312, 1.000000000000000000 ) ) 
 REPRESENTATION_ITEM ( '' )  );
#154480=CYLINDRICAL_SURFACE ( 'NONE', #178590, 13.70000000000001528 ) ;
#154488=CARTESIAN_POINT ( 'NONE',  ( -10.10090423873405285, 9.391041506135623607, -62.54717694538948791 ) ) ;
#154602=CARTESIAN_POINT ( 'NONE',  ( 20.73749492396215288, -155.7167183371838064, 0.000000000000000000 ) ) ;
#154628=CARTESIAN_POINT ( 'NONE',  ( -20.43538597629128262, 20.43538597629122222, -49.67367017693150189 ) ) ;
#154630=CARTESIAN_POINT ( 'NONE',  ( -22.45286902209802449, 1.470710558936617840, -55.62279185774873724 ) ) ;
#154639=EDGE_LOOP ( 'NONE', ( #57794, #74662 ) ) ;
#154645=CARTESIAN_POINT ( 'NONE',  ( -2.802625768539467543, -39.09149893265183806, -33.00000000000000000 ) ) ;
#154699=VERTEX_POINT ( 'NONE', #27169 ) ;
#154704=B_SPLINE_CURVE_WITH_KNOTS ( 'NONE', 3,
 ( #48629, #6077, #80928, #36409, #158764, #110281, #81900, #67755, #142605, #171962, #111274, #96102, #33450, #143593 ),
 .UNSPECIFIED., .F., .F.,
 ( 4, 2, 2, 2, 2, 2, 4 ),
 ( 0.001176765026004452036, 0.002067183656864254610, 0.002957602287724056967, 0.003402811603153957712, 0.003848020918583858023, 0.004293230234013758334, 0.004738439549443658645 ),
 .UNSPECIFIED. ) ;
#154732=DIRECTION ( 'NONE',  ( 1.000000000000000000, 0.000000000000000000, 0.000000000000000000 ) ) ;
#154764=CARTESIAN_POINT ( 'NONE',  ( -16.49741402511618560, 0.7792920370543191533, -61.43171317168472001 ) ) ;
#154789=EDGE_CURVE ( 'NONE', #64219, #70273, #75085, .T. ) ;
#154791=FACE_OUTER_BOUND ( 'NONE', #154423, .T. ) ;
#154816=CARTESIAN_POINT ( 'NONE',  ( -11.74264578624800670, 36.14014761921585972, -4.149999994537627579 ) ) ;
#154823=CARTESIAN_POINT ( 'NONE',  ( -8.898962301217514081, 0.7565710328821524389, -63.99033069988504963 ) ) ;
#154913=DIRECTION ( 'NONE',  ( 0.000000000000000000, 0.000000000000000000, -1.000000000000000000 ) ) ;
#154915=CARTESIAN_POINT ( 'NONE',  ( -1.304248841091933035E-15, -21.30000000000002913, -56.46919128290398504 ) ) ;
#154920=FACE_BOUND ( 'NONE', #56916, .T. ) ;
#154925=CARTESIAN_POINT ( 'NONE',  ( -17.31426855362218831, 15.19424636789215910, -57.70166256124682747 ) ) ;
#154960=CARTESIAN_POINT ( 'NONE',  ( 10.08838716500822130, -37.25234734385448832, -23.84483522324828542 ) ) ;
#154964=VERTEX_POINT ( 'NONE', #125124 ) ;
#155027=DIRECTION ( 'NONE',  ( -1.000000000000000000, 0.000000000000000000, 0.000000000000000000 ) ) ;
#155029=EDGE_CURVE ( 'NONE', #177280, #50694, #186821, .T. ) ;
#155031=CARTESIAN_POINT ( 'NONE',  ( 8.945340038113744896, -0.6707077324887430470, -61.92615459704094150 ) ) ;
#155050=DIRECTION ( 'NONE',  ( 1.000000000000000000, 0.000000000000000000, 0.000000000000000000 ) ) ;
#155116=ORIENTED_EDGE ( 'NONE', *, *, #45144, .F. ) ;
#155123=AXIS2_PLACEMENT_3D ( 'NONE', #142101, #111771, #96584 ) ;
#155128=CARTESIAN_POINT ( 'NONE',  ( -20.74701606029278267, -32.99105665081369665, -17.50853973932211005 ) ) ;
#155138=EDGE_CURVE ( 'NONE', #176035, #17478, #8550, .T. ) ;
#155152=CARTESIAN_POINT ( 'NONE',  ( -38.00000000000000711, -12.34694845685042708, -9.899999999999998579 ) ) ;
#155180=DIRECTION ( 'NONE',  ( -0.000000000000000000, -0.000000000000000000, 1.000000000000000000 ) ) ;
#155190=CARTESIAN_POINT ( 'NONE',  ( 14.09403216840226669, -37.74807521950865663, -24.22002746648481875 ) ) ;
#155233=EDGE_LOOP ( 'NONE', ( #168588, #19644, #190280, #171586 ) ) ;
#155236=DIRECTION ( 'NONE',  ( 0.000000000000000000, 0.000000000000000000, 1.000000000000000000 ) ) ;
#155267=CARTESIAN_POINT ( 'NONE',  ( -3.573655867282028392E-15, 2.428612866367529932E-14, 0.000000000000000000 ) ) ;
#155384=CARTESIAN_POINT ( 'NONE',  ( -3.573655867282028392E-15, 2.428612866367529932E-14, -25.00000000000000000 ) ) ;
#155400=CARTESIAN_POINT ( 'NONE',  ( 17.33018265901952759, -17.03520690664669957, -54.21489346206826809 ) ) ;
#155403=CARTESIAN_POINT ( 'NONE',  ( -0.4052355915353688109, -16.64782025964801448, -59.15693706287432008 ) ) ;
#155409=CARTESIAN_POINT ( 'NONE',  ( 1.304248841091933035E-15, 21.30000000000002913, -58.85720012050612837 ) ) ;
#155418=ORIENTED_EDGE ( 'NONE', *, *, #150147, .T. ) ;
#155424=CARTESIAN_POINT ( 'NONE',  ( -36.91746825000000598, 2.428612866367529932E-14, -1.124999997268813390 ) ) ;
#155437=CARTESIAN_POINT ( 'NONE',  ( 5.758699013978453074, 6.837351365824950733, -61.93409818843134929 ) ) ;
#155470=CARTESIAN_POINT ( 'NONE',  ( -38.00000000000000711, -12.34694845685042708, -11.64999999453762669 ) ) ;
#155473=CARTESIAN_POINT ( 'NONE',  ( 29.86685920354754842, -21.69954338932559068, -2.324999997268813345 ) ) ;
#155474=CARTESIAN_POINT ( 'NONE',  ( 0.8113027391198349703, 24.06567881303553236, -56.94052085246004680 ) ) ;
#155597=CARTESIAN_POINT ( 'NONE',  ( 4.999999999999996447, 37.66961640367475184, -18.00000000000000355 ) ) ;
#155623=CARTESIAN_POINT ( 'NONE',  ( 6.434671708797603529, -6.434671708797564449, -61.89430850415821794 ) ) ;
#155655=EDGE_LOOP ( 'NONE', ( #3467, #87009, #61679, #44341 ) ) ;
#155659=CARTESIAN_POINT ( 'NONE',  ( -7.794582437828422528, 1.499905742985387480, -62.16226466885328961 ) ) ;
#155671=ADVANCED_FACE ( 'NONE', ( #115927 ), #192143, .F. ) ;
#155720=CARTESIAN_POINT ( 'NONE',  ( 3.503282210674365071, -48.86437366581479580, -35.00000000000000000 ) ) ;
#155745=DIRECTION ( 'NONE',  ( -1.000000000000000000, 0.000000000000000000, -3.652049423109065657E-15 ) ) ;
#155754=CARTESIAN_POINT ( 'NONE',  ( -16.64831001466044214, 0.4033639900676664891, -61.36868776158049599 ) ) ;
#155815=CARTESIAN_POINT ( 'NONE',  ( -8.788868155854840936, 0.9199430937699365485, -64.01178436185547582 ) ) ;
#155871=DIRECTION ( 'NONE',  ( 1.000000000000000000, 0.000000000000000000, 0.000000000000000000 ) ) ;
#155908=DIRECTION ( 'NONE',  ( -1.000000000000000000, 0.000000000000000000, 0.000000000000000000 ) ) ;
#155913=FACE_BOUND ( 'NONE', #37038, .T. ) ;
#155926=AXIS2_PLACEMENT_3D ( 'NONE', #89142, #123431, #108276 ) ;
#155950=CARTESIAN_POINT ( 'NONE',  ( 22.30909568230050155, -31.30078617543998476, -17.06157116626960502 ) ) ;
#155977=ORIENTED_EDGE ( 'NONE', *, *, #44393, .T. ) ;
#155981=ORIENTED_EDGE ( 'NONE', *, *, #194548, .T. ) ;
#156035=CARTESIAN_POINT ( 'NONE',  ( 11.45643923738959735, 5.000000000000007105, -15.00000000000000000 ) ) ;
#156063=CARTESIAN_POINT ( 'NONE',  ( 9.549542882988127701, 9.840250911107702336, -60.43989527633940639 ) ) ;
#156065=CARTESIAN_POINT ( 'NONE',  ( -20.56965321856878148, -22.68274384282698009, -50.73755258313430971 ) ) ;
#156105=B_SPLINE_CURVE_WITH_KNOTS ( 'NONE', 3,
 ( #63463, #90806, #152489, #125139, #93794, #153482, #155474, #61464, #30145, #137321, #16966, #76638, #74669, #13976 ),
 .UNSPECIFIED., .F., .F.,
 ( 4, 2, 2, 2, 2, 2, 4 ),
 ( 1.968491853561852430E-07, 0.0003266071820641947465, 0.0006530175149430332950, 0.0009794278478218718977, 0.001305838180700710392, 0.001958658846458394536, 0.002611479512216078464 ),
 .UNSPECIFIED. ) ;
#156108=DIRECTION ( 'NONE',  ( 1.000000000000000000, 9.445700745138859830E-17, -0.000000000000000000 ) ) ;
#156118=CARTESIAN_POINT ( 'NONE',  ( -31.84446081652459526, -20.74826690461117806, -24.63985244029139565 ) ) ;
#156141=CARTESIAN_POINT ( 'NONE',  ( -1.227931366032057224E-14, -24.30000000000003268, -56.77278709839600879 ) ) ;
#156168=CARTESIAN_POINT ( 'NONE',  ( 22.81625015709510151, -31.40387420917324590, -5.924999997268812990 ) ) ;
#156178=CARTESIAN_POINT ( 'NONE',  ( 16.14548778791511907, -40.33029071462300408, -21.07572238977685686 ) ) ;
#156197=ORIENTED_EDGE ( 'NONE', *, *, #78228, .F. ) ;
#156223=VECTOR ( 'NONE', #77441, 1000.000000000000000 ) ;
#156230=CARTESIAN_POINT ( 'NONE',  ( -36.91746825000000598, 2.428612866367529932E-14, -2.624999997268813168 ) ) ;
#156301=CARTESIAN_POINT ( 'NONE',  ( -22.55670631985108443, -22.55670631985069008, -64.92279855667830191 ) ) ;
#156319=EDGE_CURVE ( 'NONE', #42366, #186567, #169625, .T. ) ;
#156346=EDGE_LOOP ( 'NONE', ( #39646, #54740, #43738 ) ) ;
#156373=CARTESIAN_POINT ( 'NONE',  ( 4.313351365237949153, 4.313351365237946489, -64.53213882399992940 ) ) ;
#156405=VERTEX_POINT ( 'NONE', #45711 ) ;
#156407=EDGE_CURVE ( 'NONE', #9769, #193343, #82426, .T. ) ;
#156415=CARTESIAN_POINT ( 'NONE',  ( 22.81625015709509441, 31.40387420917330275, -9.824999997268811569 ) ) ;
#156455=CARTESIAN_POINT ( 'NONE',  ( -23.48529157249600985, 32.32473071737754111, -8.300000000000000711 ) ) ;
#156467=CARTESIAN_POINT ( 'NONE',  ( 36.91746824999999887, 11.99521256947799053, -2.024999997268813523 ) ) ;
#156475=CARTESIAN_POINT ( 'NONE',  ( -10.38198520235570221, 9.279464826303270186, -62.49863477660405664 ) ) ;
#156506=VERTEX_POINT ( 'NONE', #133747 ) ;
#156513=VECTOR ( 'NONE', #75693, 1000.000000000000227 ) ;
#156626=CARTESIAN_POINT ( 'NONE',  ( -23.15940025311441630, 1.498759781556387560, -55.09305739490149989 ) ) ;
#156644=VECTOR ( 'NONE', #169043, 1000.000000000000000 ) ;
#156659=CIRCLE ( 'NONE', #140483, 40.00000000000000000 ) ;
#156661=CARTESIAN_POINT ( 'NONE',  ( 32.99455490591380880, -22.60464286593626326, -23.90693389968299698 ) ) ;
#156690=CIRCLE ( 'NONE', #24218, 28.90000000000004476 ) ;
#156754=DIRECTION ( 'NONE',  ( 3.613946018757868503E-15, 0.000000000000000000, -1.000000000000000000 ) ) ;
#156762=CARTESIAN_POINT ( 'NONE',  ( -0.1985533113405554273, -9.090072183657236238, -61.89635373339110913 ) ) ;
#156776=VECTOR ( 'NONE', #49641, 1000.000000000000000 ) ;
#156783=CARTESIAN_POINT ( 'NONE',  ( -2.973862142520652174, -93.04182470242764680, -15.00000000000000178 ) ) ;
#156826=CARTESIAN_POINT ( 'NONE',  ( -20.41037832431298682, -34.40082058117823749, -25.00000000000009592 ) ) ;
#156887=EDGE_CURVE ( 'NONE', #24124, #46712, #163340, .T. ) ;
#156888=CARTESIAN_POINT ( 'NONE',  ( 15.66706267174406264, -1.428615351859153559, -61.77652290643386834 ) ) ;
#156904=CARTESIAN_POINT ( 'NONE',  ( 0.000000000000000000, 0.000000000000000000, -35.00000000000000000 ) ) ;
#156910=CARTESIAN_POINT ( 'NONE',  ( 12.39597446193840469, -43.61540881465730735, -22.87833536075120122 ) ) ;
#156922=CARTESIAN_POINT ( 'NONE',  ( -16.57870055856065861, 14.68143632974463664, -58.31140971112358073 ) ) ;
#156928=VERTEX_POINT ( 'NONE', #86485 ) ;
#156953=CARTESIAN_POINT ( 'NONE',  ( 22.27567441219162703, -30.36413145305563788, -19.29304740692434805 ) ) ;
#156957=ORIENTED_EDGE ( 'NONE', *, *, #115666, .F. ) ;
#156968=CIRCLE ( 'NONE', #105299, 2.500000000000000000 ) ;
#156979=ORIENTED_EDGE ( 'NONE', *, *, #132574, .T. ) ;
#157037=CARTESIAN_POINT ( 'NONE',  ( -4.243022077861292374, -4.383680652614605933, -62.50719930893269805 ) ) ;
#157064=AXIS2_PLACEMENT_3D ( 'NONE', #3749, #65426, #141277 ) ;
#157065=CARTESIAN_POINT ( 'NONE',  ( 9.409695640424901697, 11.43209428340594158, -59.99679127084682051 ) ) ;
#157067=DIRECTION ( 'NONE',  ( -9.445700745138859830E-17, 1.000000000000000000, 0.000000000000000000 ) ) ;
#157102=ORIENTED_EDGE ( 'NONE', *, *, #32959, .F. ) ;
#157106=ORIENTED_EDGE ( 'NONE', *, *, #192484, .T. ) ;
#157130=EDGE_CURVE ( 'NONE', #77704, #121632, #14625, .T. ) ;
#157148=CARTESIAN_POINT ( 'NONE',  ( 0.000000000000000000, 0.000000000000000000, -64.92279855667830191 ) ) ;
#157168=CARTESIAN_POINT ( 'NONE',  ( -36.91746825000000598, 2.428612866367529932E-14, -6.624999997268814056 ) ) ;
#157176=DIRECTION ( 'NONE',  ( -0.000000000000000000, -0.000000000000000000, 1.000000000000000000 ) ) ;
#157178=CARTESIAN_POINT ( 'NONE',  ( 19.41322597532352745, -37.10879518268426125, -19.41738833682490650 ) ) ;
#157214=AXIS2_PLACEMENT_3D ( 'NONE', #18711, #104999, #104007 ) ;
#157218=CARTESIAN_POINT ( 'NONE',  ( -11.45643923738960268, -4.999999999999992006, -18.00000000000000000 ) ) ;
#157227=CARTESIAN_POINT ( 'NONE',  ( -17.06066397988011829, -17.30472558578613729, -54.21489346206830362 ) ) ;
#157231=CARTESIAN_POINT ( 'NONE',  ( 22.81625015709510151, -31.40387420917324590, -10.42499999726881477 ) ) ;
#157416=CARTESIAN_POINT ( 'NONE',  ( 36.91746825000000598, -11.99521256947793546, -8.224999997268810148 ) ) ;
#157424=DIRECTION ( 'NONE',  ( -0.000000000000000000, -0.000000000000000000, 1.000000000000000000 ) ) ;
#157466=CARTESIAN_POINT ( 'NONE',  ( 11.40812507854754365, 35.11059874428196537, -3.724999997268813701 ) ) ;
#157474=CARTESIAN_POINT ( 'NONE',  ( 8.969129508634463122, -36.34711360786827328, -31.52745775292089547 ) ) ;
#157482=ORIENTED_EDGE ( 'NONE', *, *, #138326, .T. ) ;
#157490=EDGE_LOOP ( 'NONE', ( #41588, #179188, #22881, #183846 ) ) ;
#157534=ORIENTED_EDGE ( 'NONE', *, *, #11291, .F. ) ;
#157599=B_SPLINE_CURVE_WITH_KNOTS ( 'NONE', 3,
 ( #34676, #142839, #84151, #190354, #114491, #4318, #160009 ),
 .UNSPECIFIED., .F., .F.,
 ( 4, 3, 4 ),
 ( -4.032110379226884939E-05, 0.000000000000000000, 0.006882574723720362095 ),
 .UNSPECIFIED. ) ;
#157616=CARTESIAN_POINT ( 'NONE',  ( 5.374011537017776341, 5.374011537017758577, -64.92279855667830191 ) ) ;
#157618=CIRCLE ( 'NONE', #96249, 2.500000000000000000 ) ;
#157619=CARTESIAN_POINT ( 'NONE',  ( -9.285066906530433428, -10.36274924941840681, -60.36157103788103484 ) ) ;
#157636=CARTESIAN_POINT ( 'NONE',  ( -29.77433414031400716, 1.366177905283920024, -51.67655205196553680 ) ) ;
#157648=VERTEX_POINT ( 'NONE', #144910 ) ;
#157652=CARTESIAN_POINT ( 'NONE',  ( -11.74264578624800670, 36.14014761921585972, -6.149999994537627579 ) ) ;
#157654=ADVANCED_FACE ( 'NONE', ( #141921 ), #3412, .F. ) ;
#157655=CARTESIAN_POINT ( 'NONE',  ( 23.48529157249600630, -32.32473071737749137, -3.049999994537627490 ) ) ;
#157668=CARTESIAN_POINT ( 'NONE',  ( 32.09281931051394565, -20.34824190692416934, -24.99999999999997868 ) ) ;
#157722=DIRECTION ( 'NONE',  ( -1.000000000000000000, -8.921435019309295657E-15, 0.000000000000000000 ) ) ;
#157741=DIRECTION ( 'NONE',  ( 0.000000000000000000, 0.000000000000000000, 1.000000000000000000 ) ) ;
#157747=CARTESIAN_POINT ( 'NONE',  ( -15.06137443927361019, -15.06137443927335440, -56.46919128290398504 ) ) ;
#157756=CARTESIAN_POINT ( 'NONE',  ( -16.70000000000002416, 0.1032682159775897418, -61.34707691135562868 ) ) ;
#157781=CARTESIAN_POINT ( 'NONE',  ( -13.29753078558959878, -35.33598341332324821, -29.59763579011278978 ) ) ;
#157791=CARTESIAN_POINT ( 'NONE',  ( 21.23184647844206197, -181.1785498424364675, 0.000000000000000000 ) ) ;
#157819=CARTESIAN_POINT ( 'NONE',  ( 1.500000000000020872, 22.80000000000002913, -55.36297086913598520 ) ) ;
#157868=EDGE_LOOP ( 'NONE', ( #2417, #157106, #128732, #100225, #44637 ) ) ;
#157871=ORIENTED_EDGE ( 'NONE', *, *, #26840, .F. ) ;
#157873=FACE_OUTER_BOUND ( 'NONE', #148985, .T. ) ;
#157899=LINE ( 'NONE', #19388, #8828 ) ;
#157909=CARTESIAN_POINT ( 'NONE',  ( 0.000000000000000000, 0.000000000000000000, -25.00000000000000000 ) ) ;
#157914=CARTESIAN_POINT ( 'NONE',  ( 4.647474457565486646E-15, -28.90000000000004476, -49.67367017693150189 ) ) ;
#157945=CARTESIAN_POINT ( 'NONE',  ( 27.86627820654178223, -25.72419401237037562, -16.61045157393441940 ) ) ;
#157973=VERTEX_POINT ( 'NONE', #126746 ) ;
#158005=AXIS2_PLACEMENT_3D ( 'NONE', #48453, #126269, #80753 ) ;
#158006=LINE ( 'NONE', #144817, #149597 ) ;
#158030=DIRECTION ( 'NONE',  ( 0.000000000000000000, 0.000000000000000000, 1.000000000000000000 ) ) ;
#158092=EDGE_LOOP ( 'NONE', ( #84052, #37345, #152992, #118469 ) ) ;
#158096=VERTEX_POINT ( 'NONE', #115592 ) ;
#158105=ORIENTED_EDGE ( 'NONE', *, *, #84631, .F. ) ;
#158107=CARTESIAN_POINT ( 'NONE',  ( -31.73299246115864136, -20.69072564976222850, -20.42656251076715535 ) ) ;
#158129=CARTESIAN_POINT ( 'NONE',  ( -31.48176515315801538, 1.054302444750109702, -46.25693415911323569 ) ) ;
#158137=CARTESIAN_POINT ( 'NONE',  ( 6.575215748390261794, -6.294127669204910625, -63.95112321872122152 ) ) ;
#158154=CARTESIAN_POINT ( 'NONE',  ( -11.40812507854754720, -35.11059874428192273, -2.224999997268813701 ) ) ;
#158164=CARTESIAN_POINT ( 'NONE',  ( 16.41350681615404739, -36.34403388527339729, -28.23867313180933536 ) ) ;
#158176=EDGE_CURVE ( 'NONE', #167693, #117777, #191407, .T. ) ;
#158185=ORIENTED_EDGE ( 'NONE', *, *, #53802, .F. ) ;
#158212=CARTESIAN_POINT ( 'NONE',  ( 37.99999999999999289, 2.428612866367529932E-14, -25.00000000000000000 ) ) ;
#158216=CARTESIAN_POINT ( 'NONE',  ( 36.91746825000000598, -11.99521256947793546, -1.724999997268813479 ) ) ;
#158246=EDGE_CURVE ( 'NONE', #64113, #77120, #124434, .T. ) ;
#158329=ORIENTED_EDGE ( 'NONE', *, *, #34682, .F. ) ;
#158396=PLANE ( 'NONE',  #194848 ) ;
#158400=CARTESIAN_POINT ( 'NONE',  ( 3.556970738554033499E-15, -38.81732327939057825, -6.624999997268814056 ) ) ;
#158416=EDGE_CURVE ( 'NONE', #35769, #165759, #180288, .T. ) ;
#158448=CARTESIAN_POINT ( 'NONE',  ( 36.91746824999999887, 11.99521256947799053, -4.024999997268814411 ) ) ;
#158455=DIRECTION ( 'NONE',  ( -0.000000000000000000, -0.000000000000000000, 1.000000000000000000 ) ) ;
#158459=CARTESIAN_POINT ( 'NONE',  ( 15.06137443927350361, 15.06137443927346098, -58.85720012050613548 ) ) ;
#158463=ORIENTED_EDGE ( 'NONE', *, *, #83102, .F. ) ;
#158488=ADVANCED_FACE ( 'NONE', ( #163092 ), #24596, .F. ) ;
#158537=DIRECTION ( 'NONE',  ( 0.000000000000000000, 0.000000000000000000, 1.000000000000000000 ) ) ;
#158554=CARTESIAN_POINT ( 'NONE',  ( 0.000000000000000000, 0.000000000000000000, -18.00000000000000000 ) ) ;
#158625=EDGE_LOOP ( 'NONE', ( #72457, #144917, #53915 ) ) ;
#158640=DIRECTION ( 'NONE',  ( -0.000000000000000000, -0.000000000000000000, 1.000000000000000000 ) ) ;
#158642=CARTESIAN_POINT ( 'NONE',  ( 19.38985940809749309, -32.68077955211924035, -24.99999999999992895 ) ) ;
#158698=CARTESIAN_POINT ( 'NONE',  ( -15.50653001719018143, -40.92458772716549475, -21.39878705119700797 ) ) ;
#158730=CARTESIAN_POINT ( 'NONE',  ( -1.461410587780170633, -7.989781499195990122, -62.12232043736380405 ) ) ;
#158763=AXIS2_PLACEMENT_3D ( 'NONE', #17243, #156754, #155745 ) ;
#158764=CARTESIAN_POINT ( 'NONE',  ( -4.520441824858469460, -6.641858834016538538, -62.14216519528071103 ) ) ;
#158775=EDGE_CURVE ( 'NONE', #28211, #193677, #119592, .T. ) ;
#158826=CARTESIAN_POINT ( 'NONE',  ( 69.65682714487590488, -71.74905178543389184, -23.00000000000000000 ) ) ;
#158848=SPHERICAL_SURFACE ( 'NONE', #75944, 10.00000000000000000 ) ;
#158857=CARTESIAN_POINT ( 'NONE',  ( 0.5391882481685079664, 24.20369912164904491, -54.28997303946584196 ) ) ;
#158873=DIRECTION ( 'NONE',  ( 1.000000000000000000, 0.000000000000000000, 0.000000000000000000 ) ) ;
#158875=DIRECTION ( 'NONE',  ( -0.000000000000000000, -0.000000000000000000, 1.000000000000000000 ) ) ;
#158885=CARTESIAN_POINT ( 'NONE',  ( -23.48529157249599919, -32.32473071737749848, -5.449999994537626513 ) ) ;
#158925=CARTESIAN_POINT ( 'NONE',  ( 28.40128899757106495, -24.57310642927003741, -18.78835905295402853 ) ) ;
#158929=ORIENTED_EDGE ( 'NONE', *, *, #60319, .T. ) ;
#158950=ORIENTED_EDGE ( 'NONE', *, *, #72173, .T. ) ;
#158953=ORIENTED_EDGE ( 'NONE', *, *, #1893, .F. ) ;
#158985=FACE_OUTER_BOUND ( 'NONE', #127093, .T. ) ;
#159034=CARTESIAN_POINT ( 'NONE',  ( -30.14078780231637467, -23.14917332716833087, -18.99124320735420568 ) ) ;
#159086=CARTESIAN_POINT ( 'NONE',  ( -32.72233185157555369, -19.32382731393326125, -21.08582493607484665 ) ) ;
#159102=ORIENTED_EDGE ( 'NONE', *, *, #127759, .F. ) ;
#159112=CARTESIAN_POINT ( 'NONE',  ( 4.979424220691216263, 6.824450432131265565, -64.09785073354592555 ) ) ;
#159118=CARTESIAN_POINT ( 'NONE',  ( 32.05902467079202012, -23.92572825132751291, -20.04789607283224839 ) ) ;
#159131=VERTEX_POINT ( 'NONE', #137723 ) ;
#159133=CARTESIAN_POINT ( 'NONE',  ( 29.86685920354754487, 21.69954338932564752, -5.424999997268813878 ) ) ;
#159143=CARTESIAN_POINT ( 'NONE',  ( 20.09009762001922894, -36.41118502145469904, -19.08443133123336111 ) ) ;
#159157=EDGE_CURVE ( 'NONE', #89664, #106917, #81543, .T. ) ;
#159163=ORIENTED_EDGE ( 'NONE', *, *, #173288, .F. ) ;
#159191=CARTESIAN_POINT ( 'NONE',  ( -14.71331571979865949, -16.70575312364977094, -55.79855980662914305 ) ) ;
#159195=CARTESIAN_POINT ( 'NONE',  ( -29.86685920354755552, 21.69954338932564397, -0.8249999972688133454 ) ) ;
#159199=CARTESIAN_POINT ( 'NONE',  ( 193.3062444957835453, -155.7167183371837496, -15.00000000000000178 ) ) ;
#159202=VECTOR ( 'NONE', #138024, 1000.000000000000000 ) ;
#159252=DIRECTION ( 'NONE',  ( -0.000000000000000000, 0.000000000000000000, 1.000000000000000000 ) ) ;
#159310=ORIENTED_EDGE ( 'NONE', *, *, #179291, .T. ) ;
#159313=CARTESIAN_POINT ( 'NONE',  ( 0.000000000000000000, 0.000000000000000000, -61.89430850415821794 ) ) ;
#159327=ORIENTED_EDGE ( 'NONE', *, *, #96802, .F. ) ;
#159343=CARTESIAN_POINT ( 'NONE',  ( 22.02608267474400350, 22.90350128981412325, -45.83983912514963066 ) ) ;
#159367=CARTESIAN_POINT ( 'NONE',  ( 1.531793102469823607E-14, -74.04165629597446241, -24.99410988461188055 ) ) ;
#159369=CARTESIAN_POINT ( 'NONE',  ( 22.81625015709509441, 31.40387420917330275, -1.324999997268813123 ) ) ;
#159375=CARTESIAN_POINT ( 'NONE',  ( 5.000000000000000000, 0.000000000000000000, -15.00000000000000000 ) ) ;
#159380=AXIS2_PLACEMENT_3D ( 'NONE', #115131, #178820, #27138 ) ;
#159385=CARTESIAN_POINT ( 'NONE',  ( 29.86685920354754842, -21.69954338932559068, -10.32499999726881335 ) ) ;
#159431=CARTESIAN_POINT ( 'NONE',  ( -22.81625015709509441, -31.40387420917324590, -2.824999997268812901 ) ) ;
#159432=CARTESIAN_POINT ( 'NONE',  ( -22.32700255269489276, 20.23564678862942401, -51.30755147637197666 ) ) ;
#159435=CIRCLE ( 'NONE', #85259, 31.90000000000003411 ) ;
#159466=AXIS2_PLACEMENT_3D ( 'NONE', #149997, #176348, #71160 ) ;
#159472=B_SPLINE_CURVE_WITH_KNOTS ( 'NONE', 3,
 ( #139842, #108524, #172187, #142828, #33672, #155031, #127660, #31696, #34666, #63011, #3328, #79174, #16526, #78173, #124690, #109517, #126659, #171199, #65991, #188363, #189360, #93345, #32689, #96324, #17516, #140845 ),
 .UNSPECIFIED., .F., .F.,
 ( 4, 2, 2, 2, 2, 2, 2, 2, 2, 2, 2, 2, 4 ),
 ( 1.971390913921884457E-07, 0.0002963316798228788642, 0.0005924662205543656125, 0.0008886007612858520897, 0.001184735302017338784, 0.001777004383480311955, 0.002369273464943285126, 0.002665408005674770736, 0.002961542546406256346, 0.003257677087137742390, 0.003553811627869227566, 0.004146080709332196183, 0.004738349790795163934 ),
 .UNSPECIFIED. ) ;
#159517=DIRECTION ( 'NONE',  ( -9.445700745138859830E-17, 1.000000000000000000, 0.000000000000000000 ) ) ;
#159521=CARTESIAN_POINT ( 'NONE',  ( 20.13687146691633245, -33.41269836094259205, -11.07851503421889561 ) ) ;
#159534=ADVANCED_FACE ( 'NONE', ( #16379 ), #158848, .T. ) ;
#159541=FACE_OUTER_BOUND ( 'NONE', #99250, .T. ) ;
#159579=CARTESIAN_POINT ( 'NONE',  ( -4.562484170633083203, -48.30423733477558557, -22.99999999999999645 ) ) ;
#159583=LINE ( 'NONE', #18119, #4670 ) ;
#159601=CARTESIAN_POINT ( 'NONE',  ( -28.90000000000004476, 2.980639576201346218E-13, -52.65483682830183199 ) ) ;
#159613=ADVANCED_FACE ( 'NONE', ( #157873 ), #96184, .T. ) ;
#159620=DIRECTION ( 'NONE',  ( -0.000000000000000000, -0.000000000000000000, 1.000000000000000000 ) ) ;
#159633=CARTESIAN_POINT ( 'NONE',  ( 11.45643923738960446, -4.999999999999992895, -18.00000000000000000 ) ) ;
#159636=CARTESIAN_POINT ( 'NONE',  ( 31.34482716061813434, -21.47441072263943695, -23.96158720469882653 ) ) ;
#159648=CARTESIAN_POINT ( 'NONE',  ( -20.05760019694261587, -21.05943304104360791, -49.45823509044233646 ) ) ;
#159671=CARTESIAN_POINT ( 'NONE',  ( -29.86685920354755552, 21.69954338932564397, -1.324999997268813345 ) ) ;
#159675=ORIENTED_EDGE ( 'NONE', *, *, #48406, .T. ) ;
#159691=CARTESIAN_POINT ( 'NONE',  ( -7.095528360789167266, -39.96100899395969464, -25.59277598900286321 ) ) ;
#159714=ADVANCED_FACE ( 'NONE', ( #113340 ), #19362, .T. ) ;
#159716=CARTESIAN_POINT ( 'NONE',  ( -11.74264578624799782, -36.14014761921581709, -9.349999994537627757 ) ) ;
#159720=DIRECTION ( 'NONE',  ( 1.000000000000000000, 0.000000000000000000, 0.000000000000000000 ) ) ;
#159804=ADVANCED_FACE ( 'NONE', ( #187237 ), #189218, .F. ) ;
#159806=ORIENTED_EDGE ( 'NONE', *, *, #77897, .F. ) ;
#159828=CARTESIAN_POINT ( 'NONE',  ( -3.573655867282028392E-15, 2.428612866367529932E-14, -18.00000000000000000 ) ) ;
#159839=VECTOR ( 'NONE', #114046, 1000.000000000000000 ) ;
#159845=ORIENTED_EDGE ( 'NONE', *, *, #40503, .F. ) ;
#159851=CARTESIAN_POINT ( 'NONE',  ( 20.41037832431316090, -34.40082058117813801, -24.99999999999991829 ) ) ;
#159862=CARTESIAN_POINT ( 'NONE',  ( 14.30340603398756016, -1.218621689577097822, -62.33590500446656790 ) ) ;
#159887=DIRECTION ( 'NONE',  ( 0.8660254037844392627, 0.000000000000000000, 0.4999999999999988898 ) ) ;
#159898=CARTESIAN_POINT ( 'NONE',  ( 4.313351365237961588, -4.313351365237934942, -64.53213882399992940 ) ) ;
#159929=CARTESIAN_POINT ( 'NONE',  ( 0.000000000000000000, 0.000000000000000000, -25.00000000000000000 ) ) ;
#159932=CARTESIAN_POINT ( 'NONE',  ( 25.66183622254818175, -27.84411637527792749, -16.56099493762766883 ) ) ;
#159960=ORIENTED_EDGE ( 'NONE', *, *, #76322, .F. ) ;
#159989=AXIS2_PLACEMENT_3D ( 'NONE', #188089, #157741, #80879 ) ;
#159994=CARTESIAN_POINT ( 'NONE',  ( 69.65682714487590488, -71.74905178543389184, 0.000000000000000000 ) ) ;
#160009=CARTESIAN_POINT ( 'NONE',  ( -6.856101608890801443E-16, -71.74905178543389184, -22.99263613531268291 ) ) ;
#160018=LINE ( 'NONE', #173210, #121020 ) ;
#160043=CARTESIAN_POINT ( 'NONE',  ( 1.227931366032057224E-14, 24.30000000000003268, -56.77278709839600879 ) ) ;
#160082=ADVANCED_FACE ( 'NONE', ( #65844 ), #182498, .T. ) ;
#160088=ORIENTED_EDGE ( 'NONE', *, *, #130640, .T. ) ;
#160098=CARTESIAN_POINT ( 'NONE',  ( -26.12775673971868784, -26.86876869530775380, -18.42961048235722288 ) ) ;
#160116=CARTESIAN_POINT ( 'NONE',  ( -1.221313414957698099E-14, 31.90000000000003411, -45.64921306006598201 ) ) ;
#160121=CARTESIAN_POINT ( 'NONE',  ( -29.56482114129869743, 1.249513161672317851, -48.84067647644815224 ) ) ;
#160124=CARTESIAN_POINT ( 'NONE',  ( 0.000000000000000000, -105.0000000000000000, 12.00000000000000355 ) ) ;
#160146=CARTESIAN_POINT ( 'NONE',  ( -22.81625015709509441, -31.40387420917324590, -4.324999997268812457 ) ) ;
#160152=EDGE_CURVE ( 'NONE', #88773, #193461, #63335, .T. ) ;
#160157=CARTESIAN_POINT ( 'NONE',  ( 29.18329815487453160, -27.17471096552231202, -17.01306446742700018 ) ) ;
#160165=EDGE_CURVE ( 'NONE', #106382, #197536, #101794, .T. ) ;
#160192=VECTOR ( 'NONE', #126308, 1000.000000000000000 ) ;
#160209=CARTESIAN_POINT ( 'NONE',  ( 36.91746824999999177, 2.880721459617395097E-14, -8.124999997268814056 ) ) ;
#160217=CYLINDRICAL_SURFACE ( 'NONE', #154131, 38.00000000000000000 ) ;
#160240=AXIS2_PLACEMENT_3D ( 'NONE', #73410, #134074, #148240 ) ;
#160245=CARTESIAN_POINT ( 'NONE',  ( 30.58708291193884676, -1.497147075633630919, -50.73425184351845729 ) ) ;
#160248=DIRECTION ( 'NONE',  ( 0.000000000000000000, 0.000000000000000000, 1.000000000000000000 ) ) ;
#160266=FACE_OUTER_BOUND ( 'NONE', #7445, .T. ) ;
#160324=ADVANCED_FACE ( 'NONE', ( #24359 ), #86010, .T. ) ;
#160343=EDGE_LOOP ( 'NONE', ( #116662, #73963, #78560, #120103 ) ) ;
#160371=CARTESIAN_POINT ( 'NONE',  ( 11.30153831258469843, -180.0000000000000000, -25.00000000000000000 ) ) ;
#160372=CARTESIAN_POINT ( 'NONE',  ( 0.5380129132520025115, 21.39578437401996425, -56.39973404422107706 ) ) ;
#160384=CARTESIAN_POINT ( 'NONE',  ( -29.86685920354755552, 21.69954338932564397, -4.824999997268814234 ) ) ;
#160394=CARTESIAN_POINT ( 'NONE',  ( -31.98945468063500641, -20.51126642791109944, -24.61382517110271806 ) ) ;
#160441=DIRECTION ( 'NONE',  ( -0.000000000000000000, -0.000000000000000000, -1.000000000000000000 ) ) ;
#160445=CARTESIAN_POINT ( 'NONE',  ( -22.89469264416805316, 22.04895058596750701, -49.28358967601001694 ) ) ;
#160480=VECTOR ( 'NONE', #126867, 1000.000000000000000 ) ;
#160537=LINE ( 'NONE', #7839, #112823 ) ;
#160562=ADVANCED_FACE ( 'NONE', ( #179045 ), #53680, .F. ) ;
#160596=CARTESIAN_POINT ( 'NONE',  ( -0.9453496423218898936, -14.01879992551668153, -62.45159313300390380 ) ) ;
#160612=CARTESIAN_POINT ( 'NONE',  ( 17.03646098637157280, -14.90092349631553859, -55.52600481601552218 ) ) ;
#160627=CARTESIAN_POINT ( 'NONE',  ( 21.02068080879936218, -34.03872152684782293, -24.45646120681608338 ) ) ;
#160629=CARTESIAN_POINT ( 'NONE',  ( -38.00000000000001421, 12.34694845685046438, -1.849999994537626424 ) ) ;
#160641=CARTESIAN_POINT ( 'NONE',  ( 0.000000000000000000, 0.000000000000000000, -60.44446360152740283 ) ) ;
#160644=CARTESIAN_POINT ( 'NONE',  ( -0.2515199893712041779, -31.88380457335792428, -49.15318026754364666 ) ) ;
#160679=CARTESIAN_POINT ( 'NONE',  ( -193.3062444957834884, -155.7167183371838064, -25.00000000000000000 ) ) ;
#160700=CARTESIAN_POINT ( 'NONE',  ( -14.29384609392722183, -37.08231061483268576, -29.62140346006266967 ) ) ;
#160701=ORIENTED_EDGE ( 'NONE', *, *, #6641, .F. ) ;
#160712=CARTESIAN_POINT ( 'NONE',  ( 9.822853212439058623, 11.94381442052172204, -61.89036147510174146 ) ) ;
#160727=FACE_OUTER_BOUND ( 'NONE', #135379, .T. ) ;
#160759=CARTESIAN_POINT ( 'NONE',  ( -11.19179774862103116, -35.88147526272305043, -30.64906824478842751 ) ) ;
#160774=ADVANCED_FACE ( 'NONE', ( #98151 ), #102184, .F. ) ;
#160858=DIRECTION ( 'NONE',  ( -1.000000000000000000, 0.000000000000000000, 0.000000000000000000 ) ) ;
#160901=CARTESIAN_POINT ( 'NONE',  ( -14.02111363790005250, 0.9482109960936973003, -60.30654223653039736 ) ) ;
#160908=ORIENTED_EDGE ( 'NONE', *, *, #150187, .F. ) ;
#160960=DIRECTION ( 'NONE',  ( 1.000000000000000000, 6.391086490440868450E-16, 0.000000000000000000 ) ) ;
#160994=ORIENTED_EDGE ( 'NONE', *, *, #126809, .F. ) ;
#161100=EDGE_CURVE ( 'NONE', #167327, #153996, #126003, .T. ) ;
#161111=ORIENTED_EDGE ( 'NONE', *, *, #195501, .T. ) ;
#161121=FACE_OUTER_BOUND ( 'NONE', #189446, .T. ) ;
#161143=CARTESIAN_POINT ( 'NONE',  ( -38.00000000000001421, 12.34694845685046438, -0.09999999999999989453 ) ) ;
#161162=DIRECTION ( 'NONE',  ( 0.000000000000000000, 0.000000000000000000, 1.000000000000000000 ) ) ;
#161177=ADVANCED_FACE ( 'NONE', ( #184000, #45483, #180055 ), #44498, .F. ) ;
#161207=CARTESIAN_POINT ( 'NONE',  ( 11.40812507854754365, 35.11059874428196537, -7.224999997268813701 ) ) ;
#161215=CARTESIAN_POINT ( 'NONE',  ( -3.573655867282028392E-15, 2.428612866367529932E-14, -25.00000000000000000 ) ) ;
#161221=ORIENTED_EDGE ( 'NONE', *, *, #85188, .T. ) ;
#161242=CARTESIAN_POINT ( 'NONE',  ( 31.90000000000003411, 0.000000000000000000, -49.13275782002545355 ) ) ;
#161245=DIRECTION ( 'NONE',  ( -0.000000000000000000, -0.000000000000000000, 1.000000000000000000 ) ) ;
#161301=ADVANCED_FACE ( 'NONE', ( #26363 ), #43506, .F. ) ;
#161345=ADVANCED_FACE ( 'NONE', ( #10361 ), #25545, .T. ) ;
#161356=DIRECTION ( 'NONE',  ( 1.000000000000000000, 0.000000000000000000, 0.000000000000000000 ) ) ;
#161402=LINE ( 'NONE', #145223, #37219 ) ;
#161460=VERTEX_POINT ( 'NONE', #118537 ) ;
#161479=EDGE_CURVE ( 'NONE', #128045, #138940, #115156, .T. ) ;
#161609=CARTESIAN_POINT ( 'NONE',  ( 17.52032980918965066, -15.56136713261939875, -54.91505165737924443 ) ) ;
#161623=ORIENTED_EDGE ( 'NONE', *, *, #171883, .F. ) ;
#161628=CARTESIAN_POINT ( 'NONE',  ( -38.00000000000001421, 12.34694845685046438, -7.849999994537626868 ) ) ;
#161635=CARTESIAN_POINT ( 'NONE',  ( 5.687983883489459380, -3.878490454473807247, -62.37234731589995107 ) ) ;
#161656=CARTESIAN_POINT ( 'NONE',  ( -20.16212008049412319, -20.78213278888862448, -49.60977668010092856 ) ) ;
#161694=DIRECTION ( 'NONE',  ( 1.000000000000000000, 0.000000000000000000, 0.000000000000000000 ) ) ;
#161831=DIRECTION ( 'NONE',  ( 1.000000000000000000, 0.000000000000000000, 0.000000000000000000 ) ) ;
#161848=ORIENTED_EDGE ( 'NONE', *, *, #103351, .F. ) ;
#161891=DIRECTION ( 'NONE',  ( -0.000000000000000000, -0.000000000000000000, 1.000000000000000000 ) ) ;
#161932=CARTESIAN_POINT ( 'NONE',  ( 32.19332086309600527, -20.18834286810123047, -25.14458231473971850 ) ) ;
#161958=DIRECTION ( 'NONE',  ( -0.000000000000000000, 0.000000000000000000, -1.000000000000000000 ) ) ;
#161959=EDGE_LOOP ( 'NONE', ( #100729, #139414, #115354, #65509 ) ) ;
#161993=ORIENTED_EDGE ( 'NONE', *, *, #116496, .F. ) ;
#162089=ORIENTED_EDGE ( 'NONE', *, *, #133615, .F. ) ;
#162090=CARTESIAN_POINT ( 'NONE',  ( -11.74264578624799782, -36.14014761921581709, -3.600000000000000533 ) ) ;
#162099=CARTESIAN_POINT ( 'NONE',  ( 0.4854043096289403225, 28.97561840829192903, -52.57160608660437617 ) ) ;
#162127=CARTESIAN_POINT ( 'NONE',  ( -193.3062444957834884, -155.7167183371838064, -25.00000000000000000 ) ) ;
#162129=CARTESIAN_POINT ( 'NONE',  ( 33.21859846492400692, -22.28383573948690710, -23.19796227011728007 ) ) ;
#162136=CYLINDRICAL_SURFACE ( 'NONE', #133633, 1.500000000000001332 ) ;
#162145=CARTESIAN_POINT ( 'NONE',  ( -11.40812507854754720, -35.11059874428192273, -10.22499999726881548 ) ) ;
#162150=DIRECTION ( 'NONE',  ( -0.000000000000000000, -0.000000000000000000, 1.000000000000000000 ) ) ;
#162154=CARTESIAN_POINT ( 'NONE',  ( 32.73422133880311691, -23.92350924394424183, -17.85299461212022365 ) ) ;
#162199=ORIENTED_EDGE ( 'NONE', *, *, #84003, .T. ) ;
#162204=CARTESIAN_POINT ( 'NONE',  ( 11.40812507854754365, 35.11059874428196537, -9.224999997268813701 ) ) ;
#162238=CYLINDRICAL_SURFACE ( 'NONE', #94731, 1.499999999999997780 ) ;
#162243=DIRECTION ( 'NONE',  ( 1.000000000000000000, 1.776356839400250465E-15, 0.000000000000000000 ) ) ;
#162247=B_SPLINE_CURVE_WITH_KNOTS ( 'NONE', 3,
 ( #102427, #194447, #191431, #87256, #52908, #88245, #131764, #164114 ),
 .UNSPECIFIED., .F., .F.,
 ( 4, 2, 2, 4 ),
 ( 2.787258272608875357E-07, 0.0002976023950119189546, 0.0005949260641965769441, 0.001189573402565897910 ),
 .UNSPECIFIED. ) ;
#162272=EDGE_LOOP ( 'NONE', ( #133097, #176327, #44782, #111468 ) ) ;
#162324=DIRECTION ( 'NONE',  ( 1.000000000000000000, 0.000000000000000000, 0.000000000000000000 ) ) ;
#162338=ORIENTED_EDGE ( 'NONE', *, *, #24130, .F. ) ;
#162356=CARTESIAN_POINT ( 'NONE',  ( -3.874011537017815421, -5.374011537017722162, -62.41807096325323556 ) ) ;
#162365=CARTESIAN_POINT ( 'NONE',  ( -27.33089735363342498, -28.79505088701986537, -20.09366309423209174 ) ) ;
#162375=CARTESIAN_POINT ( 'NONE',  ( -29.86685920354755552, 21.69954338932564397, -2.824999997268813345 ) ) ;
#162382=ORIENTED_EDGE ( 'NONE', *, *, #981, .T. ) ;
#162384=CARTESIAN_POINT ( 'NONE',  ( -31.22445544967866837, -21.66088859369465425, -21.91603554745442040 ) ) ;
#162386=DIRECTION ( 'NONE',  ( -0.3041824702427711746, 0.9526137857479314297, 1.533086186985162281E-15 ) ) ;
#162432=CIRCLE ( 'NONE', #49423, 38.00000000000000000 ) ;
#162448=CARTESIAN_POINT ( 'NONE',  ( 14.65320595882614896, 15.80137536867085046, -58.69884337265980179 ) ) ;
#162525=CARTESIAN_POINT ( 'NONE',  ( -4.647474457565486646E-15, 28.90000000000004476, -49.67367017693150189 ) ) ;
#162581=FACE_OUTER_BOUND ( 'NONE', #195982, .T. ) ;
#162604=CARTESIAN_POINT ( 'NONE',  ( 0.000000000000000000, 0.000000000000000000, -61.89430850415821794 ) ) ;
#162618=ORIENTED_EDGE ( 'NONE', *, *, #105416, .T. ) ;
#162624=CARTESIAN_POINT ( 'NONE',  ( 11.74264578624800315, -36.14014761921581709, -9.149999994537626691 ) ) ;
#162633=CARTESIAN_POINT ( 'NONE',  ( 22.63886992172671597, -22.47454271797507985, -45.64921306006598201 ) ) ;
#162637=AXIS2_PLACEMENT_3D ( 'NONE', #105215, #70898, #12238 ) ;
#162638=LINE ( 'NONE', #159633, #37976 ) ;
#162641=DIRECTION ( 'NONE',  ( -0.000000000000000000, -0.000000000000000000, 1.000000000000000000 ) ) ;
#162642=ORIENTED_EDGE ( 'NONE', *, *, #191015, .F. ) ;
#162643=DIRECTION ( 'NONE',  ( -0.000000000000000000, -0.000000000000000000, 1.000000000000000000 ) ) ;
#162677=CARTESIAN_POINT ( 'NONE',  ( 11.40812507854754365, 35.11059874428196537, -1.724999997268813479 ) ) ;
#162687=LINE ( 'NONE', #115183, #107943 ) ;
#162692=CARTESIAN_POINT ( 'NONE',  ( -2.500000000000000000, -165.0000000000000000, 12.00000000000000355 ) ) ;
#162698=ADVANCED_FACE ( 'NONE', ( #127 ), #124474, .F. ) ;
#162700=CARTESIAN_POINT ( 'NONE',  ( -22.60381889853074711, -32.71308136366489094, -20.00853410803858523 ) ) ;
#162710=ORIENTED_EDGE ( 'NONE', *, *, #129082, .T. ) ;
#162711=CARTESIAN_POINT ( 'NONE',  ( 10.52174046232667060, 12.24387616833794468, -61.59812483265029925 ) ) ;
#162715=CARTESIAN_POINT ( 'NONE',  ( 21.53159096656794347, -0.8285391498303859015, -56.30101842015765357 ) ) ;
#162735=CARTESIAN_POINT ( 'NONE',  ( -3.735172737399431091E-16, -6.100000000000006750, -62.50719930893269805 ) ) ;
#162767=DIRECTION ( 'NONE',  ( 1.000000000000000000, 0.000000000000000000, 0.000000000000000000 ) ) ;
#162809=CYLINDRICAL_SURFACE ( 'NONE', #50644, 9.100000000000001421 ) ;
#162827=FACE_OUTER_BOUND ( 'NONE', #175640, .T. ) ;
#162842=EDGE_CURVE ( 'NONE', #168486, #122419, #82802, .T. ) ;
#162852=CARTESIAN_POINT ( 'NONE',  ( 2.802625768539491968, -39.09149893265183806, -33.00000000000000000 ) ) ;
#162890=CARTESIAN_POINT ( 'NONE',  ( -69.65682714487590488, -71.74905178543390605, -25.00000000000000000 ) ) ;
#162899=CARTESIAN_POINT ( 'NONE',  ( 37.99999999999999289, 2.893978650043524126E-14, -8.749999994537628112 ) ) ;
#162904=ORIENTED_EDGE ( 'NONE', *, *, #80939, .T. ) ;
#162929=DIRECTION ( 'NONE',  ( 0.000000000000000000, 0.000000000000000000, -1.000000000000000000 ) ) ;
#162948=VECTOR ( 'NONE', #116184, 1000.000000000000000 ) ;
#163021=VECTOR ( 'NONE', #133681, 1000.000000000000000 ) ;
#163038=CARTESIAN_POINT ( 'NONE',  ( -5.374011537017813644, -5.374011537017721274, -64.92279855667830191 ) ) ;
#163046=AXIS2_PLACEMENT_3D ( 'NONE', #130012, #38040, #21872 ) ;
#163088=EDGE_CURVE ( 'NONE', #70701, #167830, #32565, .T. ) ;
#163092=FACE_OUTER_BOUND ( 'NONE', #145907, .T. ) ;
#163128=DIRECTION ( 'NONE',  ( 1.000000000000000000, 1.790682297782510931E-15, 0.000000000000000000 ) ) ;
#163130=CARTESIAN_POINT ( 'NONE',  ( 16.49581645235994642, -0.7820921006973431400, -59.22453004090981210 ) ) ;
#163149=CARTESIAN_POINT ( 'NONE',  ( 29.86685920354754842, -21.69954338932559068, -7.824999997268813345 ) ) ;
#163158=CARTESIAN_POINT ( 'NONE',  ( 28.32820575348571168, -27.54591730359781820, -18.54425385668479365 ) ) ;
#163166=DIRECTION ( 'NONE',  ( -1.000000000000000000, 0.000000000000000000, 0.000000000000000000 ) ) ;
#163171=ORIENTED_EDGE ( 'NONE', *, *, #111459, .F. ) ;
#163194=TOROIDAL_SURFACE ( 'NONE', #76002, 206.0437394197456911, 8.000000000000000000 ) ;
#163209=CARTESIAN_POINT ( 'NONE',  ( -36.91746825000000598, 2.428612866367529932E-14, -8.624999997268814056 ) ) ;
#163221=EDGE_CURVE ( 'NONE', #74970, #189816, #183185, .T. ) ;
#163292=B_SPLINE_CURVE_WITH_KNOTS ( 'NONE', 3,
 ( #113919, #4748, #37093, #66437, #174628, #3763, #98752, #159432, #145265, #33131, #20928, #82586, #64458, #144267, #190787, #52261, #17968, #160445, #21935, #130079, #79623, #38105 ),
 .UNSPECIFIED., .F., .F.,
 ( 4, 2, 2, 2, 2, 2, 2, 2, 2, 2, 4 ),
 ( 2.778238173776314926E-07, 0.0007557225233028439957, 0.001511167222788310479, 0.002266611922273776419, 0.003022056621759243011, 0.003777501321244709602, 0.004532946020730175760, 0.004910668370472912742, 0.005288390720215648856, 0.005666113069958384971, 0.006043835419701121953 ),
 .UNSPECIFIED. ) ;
#163337=( BOUNDED_SURFACE ( )  B_SPLINE_SURFACE ( 1, 2, ( 
 ( #152488, #170647, #88832, #66436, #97743, #142281, #35107, #5753, #50292, #156467, #17967, #4747, #155473, #2780, #33130, #16965, #96758, #159431, #187821, #174627, #3762, #128097, #79622, #52260, #112933, #144266, #157466, #1784, #113918, #158448, #65439, #173638, #78618, #20927, #18959, #141290, #36092, #19936, #67429, #172633, #64456, #81578, #49290, #82585, #80604, #129086, #143263, #32135, #190786, #93793, #110948, #189801, #140293, #51273, #63462, #125138, #34121, #126126, #188809, #111949, #186836, #48304, #109961, #95780, #171640, #94786, #127100, #67196, #189567, #49060, #160209, #6511, #68190, #141058, #2544, #4510, #190554, #33886, #173401, #113685, #191541, #35863, #52027, #127863, #66200, #64226, #51039, #96526, #125891, #17731, #174393, #5516, #80370, #157231, #82345, #143032, #112701, #188573, #97509, #98515, #128854 ),
 ( #129842, #126866, #159195, #142043, #20690, #34872, #144034, #53018, #50053, #175380, #36849, #158216, #19706, #176392, #21699, #83353, #37866, #18723, #145029, #114698, #156230, #79389, #187591, #110715, #172397, #95543, #3531, #65207, #111715, #81348, #70205, #100525, #22702, #102538, #165216, #55029, #41874, #71204, #195565, #147043, #119703, #180402, #11548, #24713, #69194, #181386, #25718, #9537, #40864, #84349, #26711, #86362, #8527, #103541, #164221, #73215, #39853, #131872, #87364, #116699, #88350, #148047, #150043, #149049, #99525, #134886, #161207, #178389, #133875, #146027, #10537, #72201, #7510, #101519, #193557, #56026, #117704, #196562, #130861, #58033, #163209, #192552, #132867, #179400, #57039, #194556, #162204, #118712, #54035, #115709, #177397, #38869, #23702, #85350, #60985, #139804, #124650, #59008, #169159, #27712, #105517 ) ),
 .UNSPECIFIED., .F., .F., .T. ) 
 B_SPLINE_SURFACE_WITH_KNOTS ( ( 2, 2 ),
 ( 3, 2, 2, 2, 2, 2, 2, 2, 2, 2, 2, 2, 2, 2, 2, 2, 2, 2, 2, 2, 2, 2, 2, 2, 2, 2, 2, 2, 2, 2, 2, 2, 2, 2, 2, 2, 2, 2, 2, 2, 2, 2, 2, 2, 2, 2, 2, 2, 2, 2, 3 ),
 ( 0.000000000000000000, 1.000000000000000000 ),
 ( 0.000000000000000000, 0.02000000000000000042, 0.04000000000000000083, 0.05999999999999999778, 0.08000000000000000167, 0.1000000000000000056, 0.1199999999999999956, 0.1400000000000000133, 0.1600000000000000033, 0.1799999999999999933, 0.2000000000000000111, 0.2200000000000000011, 0.2399999999999999911, 0.2600000000000000089, 0.2800000000000000266, 0.2999999999999999889, 0.3200000000000000067, 0.3400000000000000244, 0.3599999999999999867, 0.3800000000000000044, 0.4000000000000000222, 0.4199999999999999845, 0.4400000000000000022, 0.4600000000000000200, 0.4799999999999999822, 0.5000000000000000000, 0.5200000000000000178, 0.5400000000000000355, 0.5600000000000000533, 0.5799999999999999600, 0.5999999999999999778, 0.6199999999999999956, 0.6400000000000000133, 0.6600000000000000311, 0.6800000000000000488, 0.6999999999999999556, 0.7199999999999999734, 0.7399999999999999911, 0.7600000000000000089, 0.7800000000000000266, 0.8000000000000000444, 0.8199999999999999512, 0.8399999999999999689, 0.8599999999999999867, 0.8800000000000000044, 0.9000000000000000222, 0.9200000000000000400, 0.9399999999999999467, 0.9599999999999999645, 0.9799999999999999822, 1.000000000000000000 ),
 .UNSPECIFIED. ) 
 GEOMETRIC_REPRESENTATION_ITEM ( )  RATIONAL_B_SPLINE_SURFACE ( (
 ( 1.000000000000000000, 0.9510565162951535312, 1.000000000000000000, 0.9510565162951535312, 1.000000000000000000, 0.9510565162951535312, 1.000000000000000000, 0.9510565162951535312, 1.000000000000000000, 0.9510565162951535312, 1.000000000000000000, 0.9510565162951535312, 1.000000000000000000, 0.9510565162951535312, 1.000000000000000000, 0.9510565162951535312, 1.000000000000000000, 0.9510565162951535312, 1.000000000000000000, 0.9510565162951535312, 1.000000000000000000, 0.9510565162951535312, 1.000000000000000000, 0.9510565162951535312, 1.000000000000000000, 0.9510565162951535312, 1.000000000000000000, 0.9510565162951535312, 1.000000000000000000, 0.9510565162951535312, 1.000000000000000000, 0.9510565162951535312, 1.000000000000000000, 0.9510565162951535312, 1.000000000000000000, 0.9510565162951535312, 1.000000000000000000, 0.9510565162951535312, 1.000000000000000000, 0.9510565162951535312, 1.000000000000000000, 0.9510565162951535312, 1.000000000000000000, 0.9510565162951535312, 1.000000000000000000, 0.9510565162951535312, 1.000000000000000000, 0.9510565162951535312, 1.000000000000000000, 0.9510565162951535312, 1.000000000000000000, 0.9510565162951535312, 1.000000000000000000, 0.9510565162951535312, 1.000000000000000000, 0.9510565162951535312, 1.000000000000000000, 0.9510565162951535312, 1.000000000000000000, 0.9510565162951535312, 1.000000000000000000, 0.9510565162951535312, 1.000000000000000000, 0.9510565162951535312, 1.000000000000000000, 0.9510565162951535312, 1.000000000000000000, 0.9510565162951535312, 1.000000000000000000, 0.9510565162951535312, 1.000000000000000000, 0.9510565162951535312, 1.000000000000000000, 0.9510565162951535312, 1.000000000000000000, 0.9510565162951535312, 1.000000000000000000, 0.9510565162951535312, 1.000000000000000000, 0.9510565162951535312, 1.000000000000000000, 0.9510565162951535312, 1.000000000000000000, 0.9510565162951535312, 1.000000000000000000, 0.9510565162951535312, 1.000000000000000000, 0.9510565162951535312, 1.000000000000000000, 0.9510565162951535312, 1.000000000000000000, 0.9510565162951535312, 1.000000000000000000, 0.9510565162951535312, 1.000000000000000000, 0.9510565162951535312, 1.000000000000000000, 0.9510565162951535312, 1.000000000000000000, 0.9510565162951535312, 1.000000000000000000),
 ( 1.000000000000000000, 0.9510565162951535312, 1.000000000000000000, 0.9510565162951535312, 1.000000000000000000, 0.9510565162951535312, 1.000000000000000000, 0.9510565162951535312, 1.000000000000000000, 0.9510565162951535312, 1.000000000000000000, 0.9510565162951535312, 1.000000000000000000, 0.9510565162951535312, 1.000000000000000000, 0.9510565162951535312, 1.000000000000000000, 0.9510565162951535312, 1.000000000000000000, 0.9510565162951535312, 1.000000000000000000, 0.9510565162951535312, 1.000000000000000000, 0.9510565162951535312, 1.000000000000000000, 0.9510565162951535312, 1.000000000000000000, 0.9510565162951535312, 1.000000000000000000, 0.9510565162951535312, 1.000000000000000000, 0.9510565162951535312, 1.000000000000000000, 0.9510565162951535312, 1.000000000000000000, 0.9510565162951535312, 1.000000000000000000, 0.9510565162951535312, 1.000000000000000000, 0.9510565162951535312, 1.000000000000000000, 0.9510565162951535312, 1.000000000000000000, 0.9510565162951535312, 1.000000000000000000, 0.9510565162951535312, 1.000000000000000000, 0.9510565162951535312, 1.000000000000000000, 0.9510565162951535312, 1.000000000000000000, 0.9510565162951535312, 1.000000000000000000, 0.9510565162951535312, 1.000000000000000000, 0.9510565162951535312, 1.000000000000000000, 0.9510565162951535312, 1.000000000000000000, 0.9510565162951535312, 1.000000000000000000, 0.9510565162951535312, 1.000000000000000000, 0.9510565162951535312, 1.000000000000000000, 0.9510565162951535312, 1.000000000000000000, 0.9510565162951535312, 1.000000000000000000, 0.9510565162951535312, 1.000000000000000000, 0.9510565162951535312, 1.000000000000000000, 0.9510565162951535312, 1.000000000000000000, 0.9510565162951535312, 1.000000000000000000, 0.9510565162951535312, 1.000000000000000000, 0.9510565162951535312, 1.000000000000000000, 0.9510565162951535312, 1.000000000000000000, 0.9510565162951535312, 1.000000000000000000, 0.9510565162951535312, 1.000000000000000000, 0.9510565162951535312, 1.000000000000000000, 0.9510565162951535312, 1.000000000000000000, 0.9510565162951535312, 1.000000000000000000, 0.9510565162951535312, 1.000000000000000000, 0.9510565162951535312, 1.000000000000000000, 0.9510565162951535312, 1.000000000000000000, 0.9510565162951535312, 1.000000000000000000) ) ) 
 REPRESENTATION_ITEM ( '' )  SURFACE ( )  );
#163340=LINE ( 'NONE', #164347, #146969 ) ;
#163370=CARTESIAN_POINT ( 'NONE',  ( -14.65663629173027793, -15.74606964832901390, -58.72366780613685222 ) ) ;
#163386=EDGE_LOOP ( 'NONE', ( #5211, #198946, #8412, #117668 ) ) ;
#163398=EDGE_LOOP ( 'NONE', ( #162710, #103184, #40929, #54666 ) ) ;
#163403=CARTESIAN_POINT ( 'NONE',  ( 30.20036327792367814, -26.22857331006468584, -17.18026671435356434 ) ) ;
#163462=DIRECTION ( 'NONE',  ( -1.000000000000000000, 0.000000000000000000, 0.000000000000000000 ) ) ;
#163540=CARTESIAN_POINT ( 'NONE',  ( 0.000000000000000000, 0.000000000000000000, -64.92279855667830191 ) ) ;
#163595=CARTESIAN_POINT ( 'NONE',  ( -13.57915378923026317, -35.22819508409138933, -29.39033328705865245 ) ) ;
#163634=CARTESIAN_POINT ( 'NONE',  ( 20.41037832431316090, -34.40082058117813801, -24.99999999999991829 ) ) ;
#163638=CARTESIAN_POINT ( 'NONE',  ( -23.48529157249599919, -32.32473071737750558, -9.449999994537623849 ) ) ;
#163645=CARTESIAN_POINT ( 'NONE',  ( 6.874011537017774565, -5.225144896384527726, -62.00632993653601233 ) ) ;
#163651=CARTESIAN_POINT ( 'NONE',  ( -10.87998047749161046, 9.250641775538069211, -60.21451611132643222 ) ) ;
#163690=CARTESIAN_POINT ( 'NONE',  ( 3.556970738554034288E-15, -38.81732327939057114, -4.624999997268814056 ) ) ;
#163713=CARTESIAN_POINT ( 'NONE',  ( -21.14397880779349137, -35.31393329058855102, -18.60109459635327767 ) ) ;
#163714=EDGE_LOOP ( 'NONE', ( #78446, #107198, #32080, #10973 ) ) ;
#163727=VECTOR ( 'NONE', #9012, 1000.000000000000000 ) ;
#163730=CARTESIAN_POINT ( 'NONE',  ( -1.461319442807290869, -7.990187535671176455, -64.16708268805476223 ) ) ;
#163849=CARTESIAN_POINT ( 'NONE',  ( -30.07467525274877218, -23.10311534983929249, -22.45479934155870083 ) ) ;
#163869=ORIENTED_EDGE ( 'NONE', *, *, #134694, .T. ) ;
#163881=VECTOR ( 'NONE', #71599, 1000.000000000000000 ) ;
#163905=CARTESIAN_POINT ( 'NONE',  ( -10.85402516922718874, -12.25173339339350775, -59.29444586289682206 ) ) ;
#163921=CARTESIAN_POINT ( 'NONE',  ( 3.503282210674363295, -48.86437366581479580, -23.00000000000000000 ) ) ;
#163939=EDGE_LOOP ( 'NONE', ( #55934, #55284, #67905, #104709, #43500 ) ) ;
#163998=EDGE_CURVE ( 'NONE', #149545, #106915, #74774, .T. ) ;
#164114=CARTESIAN_POINT ( 'NONE',  ( -9.248023074035629065, -10.74802307403544077, -62.40259441833023857 ) ) ;
#164138=DIRECTION ( 'NONE',  ( -0.000000000000000000, -0.000000000000000000, 1.000000000000000000 ) ) ;
#164141=CARTESIAN_POINT ( 'NONE',  ( 4.000000000000000888, -105.0000000000000000, 12.00000000000000355 ) ) ;
#164148=VERTEX_POINT ( 'NONE', #59584 ) ;
#164162=CARTESIAN_POINT ( 'NONE',  ( -22.81625015709510507, 31.40387420917330275, -6.924999997268812990 ) ) ;
#164167=CARTESIAN_POINT ( 'NONE',  ( 1.491173228115779237, 15.38774048274545159, -59.71317227968791030 ) ) ;
#164171=CARTESIAN_POINT ( 'NONE',  ( 33.12942481080231971, -22.41379292486335117, -24.08540372093460746 ) ) ;
#164187=CARTESIAN_POINT ( 'NONE',  ( -4.000000000000000888, -105.0000000000000000, 12.00000000000000355 ) ) ;
#164191=ORIENTED_EDGE ( 'NONE', *, *, #179533, .T. ) ;
#164197=CARTESIAN_POINT ( 'NONE',  ( -4.215739103160454526, -48.58376198229541387, -25.00000000000007105 ) ) ;
#164208=ADVANCED_FACE ( 'NONE', ( #5863 ), #97852, .F. ) ;
#164218=CARTESIAN_POINT ( 'NONE',  ( 22.73749492396215288, -155.7167183371838064, 0.000000000000000000 ) ) ;
#164221=CARTESIAN_POINT ( 'NONE',  ( 11.40812507854755253, -35.11059874428192273, -6.024999997268814411 ) ) ;
#164231=B_SPLINE_CURVE_WITH_KNOTS ( 'NONE', 3,
 ( #138277, #126088, #91748, #199960, #61425, #185785 ),
 .UNSPECIFIED., .F., .F.,
 ( 4, 2, 4 ),
 ( 0.003715511750470261790, 0.004312155465044938130, 0.004908799179619614469 ),
 .UNSPECIFIED. ) ;
#164284=CARTESIAN_POINT ( 'NONE',  ( 37.66961640367472341, 5.000000000000023981, -18.00000000000000355 ) ) ;
#164346=VERTEX_POINT ( 'NONE', #50401 ) ;
#164347=CARTESIAN_POINT ( 'NONE',  ( -6.434671708797631950, -6.434671708797536027, -64.92279855667830191 ) ) ;
#164358=ORIENTED_EDGE ( 'NONE', *, *, #52799, .F. ) ;
#164373=CARTESIAN_POINT ( 'NONE',  ( -11.55487914182271147, -42.80721638308652643, -21.19679778042607410 ) ) ;
#164374=EDGE_CURVE ( 'NONE', #22185, #117961, #2145, .T. ) ;
#164379=CARTESIAN_POINT ( 'NONE',  ( 12.50000000000001066, -90.00000000000005684, -15.00000000000000178 ) ) ;
#164399=CARTESIAN_POINT ( 'NONE',  ( 22.81625015709510151, -31.40387420917324590, -7.924999997268812990 ) ) ;
#164409=CARTESIAN_POINT ( 'NONE',  ( 29.82769333492476704, -26.65767662149077211, -16.82146015663694882 ) ) ;
#164466=CARTESIAN_POINT ( 'NONE',  ( 1.486117417673710336E-14, -69.45644693201178654, -24.99410988519313648 ) ) ;
#164602=CARTESIAN_POINT ( 'NONE',  ( 1.464819237669550356, 14.82474175162738383, -59.95888713364202260 ) ) ;
#164603=ADVANCED_FACE ( 'NONE', ( #159541 ), #94898, .T. ) ;
#164623=CARTESIAN_POINT ( 'NONE',  ( 12.24802307403560953, -10.59827931221447805, -59.37567494090387044 ) ) ;
#164638=CARTESIAN_POINT ( 'NONE',  ( -38.00000000000000711, 2.428612866367529932E-14, -9.749999994537626336 ) ) ;
#164654=LINE ( 'NONE', #178829, #93083 ) ;
#164656=CARTESIAN_POINT ( 'NONE',  ( -1.114265510929671077, -29.39134536520999319, -52.10946600208642820 ) ) ;
#164668=FACE_OUTER_BOUND ( 'NONE', #64960, .T. ) ;
#164689=CARTESIAN_POINT ( 'NONE',  ( 22.81625015709510151, -31.40387420917324590, -4.424999997268812990 ) ) ;
#164712=CARTESIAN_POINT ( 'NONE',  ( -30.57338251523015771, -25.88377959333046974, -17.25078043576605680 ) ) ;
#164713=ORIENTED_EDGE ( 'NONE', *, *, #117840, .F. ) ;
#164723=EDGE_LOOP ( 'NONE', ( #40936, #118682, #195560, #134548 ) ) ;
#164727=CARTESIAN_POINT ( 'NONE',  ( 21.94965239947789826, -1.250870343808790031, -55.99511580764674790 ) ) ;
#164740=CYLINDRICAL_SURFACE ( 'NONE', #191722, 5.000000000000000000 ) ;
#164843=CARTESIAN_POINT ( 'NONE',  ( -5.184702103851166477, 3.882744257519115560, -62.44399821614915425 ) ) ;
#164860=ORIENTED_EDGE ( 'NONE', *, *, #192121, .T. ) ;
#164864=ORIENTED_EDGE ( 'NONE', *, *, #115833, .F. ) ;
#164884=ORIENTED_EDGE ( 'NONE', *, *, #1430, .T. ) ;
#164915=CARTESIAN_POINT ( 'NONE',  ( -5.070555798855037821, -6.850306330133427934, -64.08177057783885289 ) ) ;
#164970=DIRECTION ( 'NONE',  ( -3.491481338843133355E-15, 0.000000000000000000, 1.000000000000000000 ) ) ;
#165008=CARTESIAN_POINT ( 'NONE',  ( -3.573655867282028392E-15, 2.428612866367529932E-14, -15.00000000000000000 ) ) ;
#165015=EDGE_CURVE ( 'NONE', #159131, #174271, #59721, .T. ) ;
#165039=CARTESIAN_POINT ( 'NONE',  ( 2.973862142520697471, -93.04182470242777470, -15.00000000000000178 ) ) ;
#165098=ORIENTED_EDGE ( 'NONE', *, *, #119454, .F. ) ;
#165135=CARTESIAN_POINT ( 'NONE',  ( 16.52479559737576764, -14.65015464700936576, -58.35289975817769914 ) ) ;
#165143=PLANE ( 'NONE',  #169261 ) ;
#165157=CARTESIAN_POINT ( 'NONE',  ( -6.020228577223754586E-15, 39.95556452105416412, -0.4999999999999999445 ) ) ;
#165183=CARTESIAN_POINT ( 'NONE',  ( 7.282160400439392944, -46.44936954762798109, -22.53643251332693254 ) ) ;
#165213=EDGE_CURVE ( 'NONE', #123757, #132572, #21700, .T. ) ;
#165216=CARTESIAN_POINT ( 'NONE',  ( 11.40812507854755253, -35.11059874428192273, -4.024999997268814411 ) ) ;
#165220=CARTESIAN_POINT ( 'NONE',  ( 6.442614714193029890, -4.311334843530821637, -64.24190475577076143 ) ) ;
#165275=CARTESIAN_POINT ( 'NONE',  ( -27.86273085795036408, -28.69962071417357663, -15.00000000000000178 ) ) ;
#165287=ORIENTED_EDGE ( 'NONE', *, *, #135559, .T. ) ;
#165378=CARTESIAN_POINT ( 'NONE',  ( -14.62203461105316826, -15.93943620433476838, -56.24376339824761573 ) ) ;
#165391=ORIENTED_EDGE ( 'NONE', *, *, #77460, .F. ) ;
#165394=CARTESIAN_POINT ( 'NONE',  ( -31.58488912581707098, -24.54536626606730110, -19.09122180200634133 ) ) ;
#165412=CARTESIAN_POINT ( 'NONE',  ( 4.576660509524177911, -38.96431129323279663, -32.99999999890352598 ) ) ;
#165599=CARTESIAN_POINT ( 'NONE',  ( 1.323952442993630241, 14.46947684450821647, -60.11301529061759652 ) ) ;
#165634=CARTESIAN_POINT ( 'NONE',  ( -11.74264578624800670, 36.14014761921585972, -4.149999994537627579 ) ) ;
#165658=CARTESIAN_POINT ( 'NONE',  ( -23.94686256013568837, 0.9720251121417748941, -57.02522261278123494 ) ) ;
#165681=ORIENTED_EDGE ( 'NONE', *, *, #179533, .F. ) ;
#165684=CARTESIAN_POINT ( 'NONE',  ( -22.81625015709510507, 31.40387420917330275, -5.424999997268812990 ) ) ;
#165707=CARTESIAN_POINT ( 'NONE',  ( -27.14096102835633317, -28.70429377953645655, -18.51261060099007949 ) ) ;
#165708=ORIENTED_EDGE ( 'NONE', *, *, #53785, .F. ) ;
#165734=CARTESIAN_POINT ( 'NONE',  ( 11.80868324581538253, -11.80868324581533457, -59.13370768023891344 ) ) ;
#165735=CARTESIAN_POINT ( 'NONE',  ( 6.941067294099604545, -1.351053078614634639, -64.37011660792191492 ) ) ;
#165759=VERTEX_POINT ( 'NONE', #18724 ) ;
#165779=CARTESIAN_POINT ( 'NONE',  ( -38.00000000000000711, 2.428612866367529932E-14, -5.749999994537626336 ) ) ;
#165816=EDGE_CURVE ( 'NONE', #115376, #157973, #127864, .T. ) ;
#165822=DIRECTION ( 'NONE',  ( -0.000000000000000000, 0.000000000000000000, -1.000000000000000000 ) ) ;
#165839=CARTESIAN_POINT ( 'NONE',  ( -6.673813065215404627, 4.619076279717873490, -62.12322917040971504 ) ) ;
#165845=AXIS2_PLACEMENT_3D ( 'NONE', #22535, #147889, #192388 ) ;
#165878=ORIENTED_EDGE ( 'NONE', *, *, #98431, .T. ) ;
#165887=DIRECTION ( 'NONE',  ( 1.000000000000000000, 8.881784197001252323E-16, 0.000000000000000000 ) ) ;
#165913=ORIENTED_EDGE ( 'NONE', *, *, #97744, .F. ) ;
#165976=VECTOR ( 'NONE', #134335, 999.9999999999998863 ) ;
#165978=CARTESIAN_POINT ( 'NONE',  ( 0.000000000000000000, 0.000000000000000000, -52.65483682830183199 ) ) ;
#166000=LINE ( 'NONE', #12327, #88107 ) ;
#166003=EDGE_LOOP ( 'NONE', ( #10328, #14859 ) ) ;
#166005=CARTESIAN_POINT ( 'NONE',  ( 24.30000000000003268, -9.712231019420881533E-14, -64.92279855667830191 ) ) ;
#166136=CARTESIAN_POINT ( 'NONE',  ( 13.70000000000000817, -0.2077008434174363316, -60.44446360152740993 ) ) ;
#166146=CYLINDRICAL_SURFACE ( 'NONE', #172449, 7.999999999999998224 ) ;
#166152=ORIENTED_EDGE ( 'NONE', *, *, #190234, .T. ) ;
#166156=CARTESIAN_POINT ( 'NONE',  ( -38.00000000000001421, -12.34694845685042708, -3.899999999999999911 ) ) ;
#166185=VERTEX_POINT ( 'NONE', #45586 ) ;
#166206=AXIS2_PLACEMENT_3D ( 'NONE', #57571, #151568, #28245 ) ;
#166258=( GEOMETRIC_REPRESENTATION_CONTEXT ( 3 ) GLOBAL_UNCERTAINTY_ASSIGNED_CONTEXT ( ( #142968 ) ) GLOBAL_UNIT_ASSIGNED_CONTEXT ( ( #28026, #103847, #10848 ) ) REPRESENTATION_CONTEXT ( 'NONE', 'WORKASPACE' ) );
#166285=ORIENTED_EDGE ( 'NONE', *, *, #191135, .T. ) ;
#166286=( BOUNDED_CURVE ( )  B_SPLINE_CURVE ( 2, ( #104211, #195236, #146707, #180085, #23380, #69879, #41554, #26393, #8204, #54706, #147730 ),
 .UNSPECIFIED., .F., .T. ) 
 B_SPLINE_CURVE_WITH_KNOTS ( ( 3, 2, 2, 2, 2, 3 ),
 ( 0.4000000000000000222, 0.4199999999999999845, 0.4400000000000000022, 0.4600000000000000200, 0.4799999999999999822, 0.5000000000000000000 ),
 .UNSPECIFIED. ) 
 CURVE ( )  GEOMETRIC_REPRESENTATION_ITEM ( )  RATIONAL_B_SPLINE_CURVE ( ( 1.000000000000000000, 0.9510565162951535312, 1.000000000000000000, 0.9510565162951535312, 1.000000000000000000, 0.9510565162951535312, 1.000000000000000000, 0.9510565162951535312, 1.000000000000000000, 0.9510565162951535312, 1.000000000000000000 ) ) 
 REPRESENTATION_ITEM ( '' )  );
#166340=ORIENTED_EDGE ( 'NONE', *, *, #158246, .F. ) ;
#166342=AXIS2_PLACEMENT_3D ( 'NONE', #51910, #156108, #2423 ) ;
#166356=AXIS2_PLACEMENT_3D ( 'NONE', #117223, #180916, #11057 ) ;
#166374=CARTESIAN_POINT ( 'NONE',  ( -14.92453577844291424, -15.21309657316540509, -58.85011498497254934 ) ) ;
#166392=CARTESIAN_POINT ( 'NONE',  ( 36.91746824999999177, 2.880721459617395097E-14, -9.624999997268814056 ) ) ;
#166402=CARTESIAN_POINT ( 'NONE',  ( -7.656827144875921753, -71.74905178543390605, -25.00000000000000000 ) ) ;
#166452=CYLINDRICAL_SURFACE ( 'NONE', #135133, 8.000000000000000000 ) ;
#166480=VECTOR ( 'NONE', #1129, 1000.000000000000000 ) ;
#166486=ADVANCED_FACE ( 'NONE', ( #116306 ), #13135, .F. ) ;
#166578=VECTOR ( 'NONE', #140485, 1000.000000000000000 ) ;
#166599=CARTESIAN_POINT ( 'NONE',  ( 0.000000000000000000, 0.000000000000000000, -64.92279855667830191 ) ) ;
#166619=CARTESIAN_POINT ( 'NONE',  ( -11.30153831258470731, -188.0000000000000000, -25.00000000000000000 ) ) ;
#166628=ORIENTED_EDGE ( 'NONE', *, *, #52535, .T. ) ;
#166634=CARTESIAN_POINT ( 'NONE',  ( 36.91746824999999887, 11.99521256947799053, -2.024999997268813523 ) ) ;
#166647=CARTESIAN_POINT ( 'NONE',  ( -12.20125963778088796, 10.33027487414774193, -59.47400725600234495 ) ) ;
#166674=B_SPLINE_CURVE_WITH_KNOTS ( 'NONE', 3,
 ( #61608, #74818, #75791, #182996, #1935, #137469, #139446, #186986, #123277, #108112, #199149, #110114, #121304, #92940 ),
 .UNSPECIFIED., .F., .F.,
 ( 4, 2, 2, 2, 2, 2, 4 ),
 ( 0.003265479109357864295, 0.004052109043202368685, 0.004445424010124612857, 0.004838738977046857029, 0.005625368910891345373, 0.006018683877813588677, 0.006411998844735832849 ),
 .UNSPECIFIED. ) ;
#166685=CARTESIAN_POINT ( 'NONE',  ( 29.86685920354754842, -21.69954338932559068, -4.324999997268814234 ) ) ;
#166706=CARTESIAN_POINT ( 'NONE',  ( -21.50179914128360892, -34.93963825065945628, -18.44273973154475854 ) ) ;
#166721=CARTESIAN_POINT ( 'NONE',  ( 21.30000000000002913, 0.000000000000000000, -56.46919128290398504 ) ) ;
#166752=EDGE_CURVE ( 'NONE', #188843, #123761, #196022, .T. ) ;
#166806=VERTEX_POINT ( 'NONE', #55633 ) ;
#166836=CARTESIAN_POINT ( 'NONE',  ( -4.460769206500190265, 4.179973224035743229, -62.50518786092071366 ) ) ;
#166858=DIRECTION ( 'NONE',  ( -0.000000000000000000, 0.000000000000000000, -1.000000000000000000 ) ) ;
#166867=AXIS2_PLACEMENT_3D ( 'NONE', #7587, #102619, #39936 ) ;
#166875=EDGE_LOOP ( 'NONE', ( #110411, #114352, #19881, #57003 ) ) ;
#166905=CARTESIAN_POINT ( 'NONE',  ( 4.790240017743697010, -48.14548474357627583, -22.95279619250844050 ) ) ;
#166955=ADVANCED_FACE ( 'NONE', ( #57649 ), #162809, .F. ) ;
#166962=CARTESIAN_POINT ( 'NONE',  ( 69.65682714487590488, -71.74905178543389184, -15.00000000000000178 ) ) ;
#166964=EDGE_CURVE ( 'NONE', #94189, #159131, #10145, .T. ) ;
#167030=CARTESIAN_POINT ( 'NONE',  ( -8.349412516403756257, 1.313804288003871612, -64.09731636040744718 ) ) ;
#167083=EDGE_LOOP ( 'NONE', ( #143694, #58527, #38751, #834 ) ) ;
#167121=CARTESIAN_POINT ( 'NONE',  ( 17.62203461105334412, -15.97128521727769446, -57.16225127900796821 ) ) ;
#167136=CIRCLE ( 'NONE', #89622, 5.000000000000000000 ) ;
#167141=ORIENTED_EDGE ( 'NONE', *, *, #62577, .F. ) ;
#167144=CARTESIAN_POINT ( 'NONE',  ( -23.48529157249599919, -32.32473071737750558, -7.699999999999999289 ) ) ;
#167149=CARTESIAN_POINT ( 'NONE',  ( -3.573655867282028392E-15, 2.428612866367529932E-14, -25.00000000000000000 ) ) ;
#167160=VECTOR ( 'NONE', #96960, 1000.000000000000000 ) ;
#167202=CARTESIAN_POINT ( 'NONE',  ( 0.9451604965124735802, 14.01865473875232304, -62.45165202555292439 ) ) ;
#167259=DIRECTION ( 'NONE',  ( 1.000000000000000000, 0.000000000000000000, 0.000000000000000000 ) ) ;
#167287=DIRECTION ( 'NONE',  ( 0.000000000000000000, 0.000000000000000000, 1.000000000000000000 ) ) ;
#167327=VERTEX_POINT ( 'NONE', #6171 ) ;
#167336=CARTESIAN_POINT ( 'NONE',  ( -11.44429459767042090, -35.82063519324131562, -30.53178620540835553 ) ) ;
#167352=CARTESIAN_POINT ( 'NONE',  ( -27.39934578958840206, -26.16170490841989249, -16.57183124570353883 ) ) ;
#167366=CARTESIAN_POINT ( 'NONE',  ( 20.58216519391595156, -20.30265720351238201, -52.64392108347575316 ) ) ;
#167376=CARTESIAN_POINT ( 'NONE',  ( 29.86685920354754487, 21.69954338932564752, -7.424999997268813878 ) ) ;
#167395=CARTESIAN_POINT ( 'NONE',  ( 9.824205582582273166, -39.25481172344606762, -25.36904614590414297 ) ) ;
#167510=ORIENTED_EDGE ( 'NONE', *, *, #16720, .T. ) ;
#167598=CARTESIAN_POINT ( 'NONE',  ( -1.324169127979094807, -14.46985881644524063, -60.11284999819413599 ) ) ;
#167604=CARTESIAN_POINT ( 'NONE',  ( 10.79449291341264328, -9.218202637343335226, -60.25055865658766407 ) ) ;
#167613=ORIENTED_EDGE ( 'NONE', *, *, #139743, .F. ) ;
#167619=CARTESIAN_POINT ( 'NONE',  ( 36.91746824999999887, 11.99521256947799053, -6.024999997268811747 ) ) ;
#167636=SPHERICAL_SURFACE ( 'NONE', #4547, 38.00000000000002132 ) ;
#167669=CARTESIAN_POINT ( 'NONE',  ( -22.81625015709510507, 31.40387420917330275, -9.424999997268812990 ) ) ;
#167686=ORIENTED_EDGE ( 'NONE', *, *, #166752, .T. ) ;
#167693=VERTEX_POINT ( 'NONE', #52107 ) ;
#167717=CARTESIAN_POINT ( 'NONE',  ( 6.691186640346301395, -1.197302953328933883, -64.41832325557876970 ) ) ;
#167724=DIRECTION ( 'NONE',  ( -0.000000000000000000, -0.000000000000000000, -1.000000000000000000 ) ) ;
#167739=ORIENTED_EDGE ( 'NONE', *, *, #186918, .F. ) ;
#167811=AXIS2_PLACEMENT_3D ( 'NONE', #147849, #144822, #132669 ) ;
#167821=CARTESIAN_POINT ( 'NONE',  ( 0.000000000000000000, 0.000000000000000000, -64.92279855667830191 ) ) ;
#167830=VERTEX_POINT ( 'NONE', #81424 ) ;
#167845=CIRCLE ( 'NONE', #22632, 206.0437394197456911 ) ;
#167865=LINE ( 'NONE', #29365, #44482 ) ;
#167871=EDGE_CURVE ( 'NONE', #113699, #99783, #57168, .T. ) ;
#167884=CARTESIAN_POINT ( 'NONE',  ( 27.93585545099115919, -25.65867777193838606, -16.61539413803383169 ) ) ;
#167908=CARTESIAN_POINT ( 'NONE',  ( -6.131632772416347521, 4.064918688780001510, -64.31816925299780507 ) ) ;
#167919=ORIENTED_EDGE ( 'NONE', *, *, #77460, .T. ) ;
#167942=ORIENTED_EDGE ( 'NONE', *, *, #105746, .F. ) ;
#167952=DIRECTION ( 'NONE',  ( -0.000000000000000000, -0.000000000000000000, 1.000000000000000000 ) ) ;
#167976=ORIENTED_EDGE ( 'NONE', *, *, #35293, .T. ) ;
#168012=CARTESIAN_POINT ( 'NONE',  ( -6.292920404648713273, 0.7621229312825712476, -64.49503546857650349 ) ) ;
#168075=CARTESIAN_POINT ( 'NONE',  ( 16.70000000000003482, -0.1032682159774155756, -61.34707691135563579 ) ) ;
#168087=FACE_OUTER_BOUND ( 'NONE', #114100, .T. ) ;
#168090=CARTESIAN_POINT ( 'NONE',  ( 38.00000000000002842, 12.34694845685041109, -6.649999994537624914 ) ) ;
#168096=CARTESIAN_POINT ( 'NONE',  ( 8.839334217631813928, -46.13630234914187156, -24.17074550867518923 ) ) ;
#168112=VECTOR ( 'NONE', #88922, 1000.000000000000000 ) ;
#168116=ORIENTED_EDGE ( 'NONE', *, *, #116420, .F. ) ;
#168119=CARTESIAN_POINT ( 'NONE',  ( 23.48529157249600630, -32.32473071737749137, -3.300000000000000266 ) ) ;
#168129=DIRECTION ( 'NONE',  ( 0.000000000000000000, 0.000000000000000000, -1.000000000000000000 ) ) ;
#168144=CARTESIAN_POINT ( 'NONE',  ( 16.87022414722825303, -33.99382086345632104, -27.12615631800316507 ) ) ;
#168171=ORIENTED_EDGE ( 'NONE', *, *, #154300, .T. ) ;
#168172=ORIENTED_EDGE ( 'NONE', *, *, #47533, .F. ) ;
#168261=CARTESIAN_POINT ( 'NONE',  ( -21.91292544274605092, -22.94826072392755378, -49.35653942980806619 ) ) ;
#168298=ORIENTED_EDGE ( 'NONE', *, *, #72533, .T. ) ;
#168309=EDGE_CURVE ( 'NONE', #82035, #12418, #86442, .T. ) ;
#168311=CARTESIAN_POINT ( 'NONE',  ( -16.98531384170231817, -34.11756901830543143, -21.70785296103623452 ) ) ;
#168342=CARTESIAN_POINT ( 'NONE',  ( 20.74300244486288847, -20.19516923136415443, -52.60240525300990555 ) ) ;
#168352=CARTESIAN_POINT ( 'NONE',  ( 36.91746824999999177, 2.880721459617395097E-14, -5.624999997268813168 ) ) ;
#168362=CARTESIAN_POINT ( 'NONE',  ( -6.434671708797631950, -6.434671708797536027, -63.95112321872120731 ) ) ;
#168372=CARTESIAN_POINT ( 'NONE',  ( -11.69814101308375065, -11.91922547854696113, -61.34707691135562158 ) ) ;
#168427=PLANE ( 'NONE',  #8803 ) ;
#168486=VERTEX_POINT ( 'NONE', #8611 ) ;
#168575=FACE_BOUND ( 'NONE', #118359, .T. ) ;
#168581=CARTESIAN_POINT ( 'NONE',  ( -22.13758331326615902, -22.85500914106531312, -45.77467392966760684 ) ) ;
#168588=ORIENTED_EDGE ( 'NONE', *, *, #32959, .T. ) ;
#168596=CARTESIAN_POINT ( 'NONE',  ( 36.91746824999999887, 11.99521256947799053, -4.024999997268814411 ) ) ;
#168608=CARTESIAN_POINT ( 'NONE',  ( 6.293041912674292249, 6.576301504920881946, -61.89430850415822505 ) ) ;
#168618=CARTESIAN_POINT ( 'NONE',  ( -22.98313974082795141, 1.499560036715340994, -57.70434786042496000 ) ) ;
#168643=CARTESIAN_POINT ( 'NONE',  ( 29.86685920354754842, -21.69954338932559068, -8.324999997268813345 ) ) ;
#168646=CARTESIAN_POINT ( 'NONE',  ( 0.4878707274068331268, 9.021887631461126489, -63.96636194779098616 ) ) ;
#168666=ORIENTED_EDGE ( 'NONE', *, *, #39485, .T. ) ;
#168782=B_SPLINE_CURVE_WITH_KNOTS ( 'NONE', 3,
 ( #33282, #81731, #185978, #32289, #142436, #1937, #47462, #96915, #62604, #171794, #156626, #92944, #154630, #65595, #187972, #141447, #79776, #93944, #48459, #140447, #16125, #94942 ),
 .UNSPECIFIED., .F., .F.,
 ( 4, 2, 2, 2, 2, 2, 2, 2, 2, 2, 4 ),
 ( 1.967889508984713855E-07, 0.0003311341139581566229, 0.0006620714389654147689, 0.0009930087639726729691, 0.001323946088979931169, 0.002647695389008995412, 0.003309570039023526991, 0.003971444689038058570, 0.004633319339052590149, 0.004964256664059855939, 0.005295193989067121729 ),
 .UNSPECIFIED. ) ;
#168802=EDGE_LOOP ( 'NONE', ( #38304, #424, #38360, #37833 ) ) ;
#168885=CARTESIAN_POINT ( 'NONE',  ( -19.70810511599105297, -36.80807878390137944, -19.26229262562157274 ) ) ;
#168913=AXIS2_PLACEMENT_3D ( 'NONE', #24503, #86154, #118505 ) ;
#168917=EDGE_LOOP ( 'NONE', ( #46487, #42134, #191674, #185041 ) ) ;
#168945=DIRECTION ( 'NONE',  ( 3.469446951953612217E-15, 0.000000000000000000, -1.000000000000000000 ) ) ;
#168960=DIRECTION ( 'NONE',  ( -1.000000000000000000, 0.000000000000000000, 0.000000000000000000 ) ) ;
#168978=CARTESIAN_POINT ( 'NONE',  ( 23.48529157249599564, 32.32473071737754111, -4.449999994537627401 ) ) ;
#168981=EDGE_CURVE ( 'NONE', #108968, #45388, #28169, .T. ) ;
#168986=CARTESIAN_POINT ( 'NONE',  ( -7.121805330552559710, 1.425084765988153368, -64.33521149768085934 ) ) ;
#169043=DIRECTION ( 'NONE',  ( -0.8571673007021135549, 1.049727191138620175E-16, 0.5150380749100520461 ) ) ;
#169052=CARTESIAN_POINT ( 'NONE',  ( 16.09882439466104032, -1.216645939406789445, -61.59766612755957738 ) ) ;
#169069=CYLINDRICAL_SURFACE ( 'NONE', #90146, 16.70000000000002061 ) ;
#169071=CARTESIAN_POINT ( 'NONE',  ( -11.30153831258470731, -180.0000000000000000, -15.00000000000000178 ) ) ;
#169075=CARTESIAN_POINT ( 'NONE',  ( 22.72061570927962393, -33.65877872499203960, -17.91763856381927411 ) ) ;
#169077=CARTESIAN_POINT ( 'NONE',  ( 11.30153831258470731, -180.0000000000000000, -25.00000000000000000 ) ) ;
#169079=CARTESIAN_POINT ( 'NONE',  ( -0.9791052130474502402, -23.94081952771227151, -54.49391133501601558 ) ) ;
#169089=CARTESIAN_POINT ( 'NONE',  ( -16.39429727647829083, 14.63400850047063528, -58.42335914450119816 ) ) ;
#169098=CARTESIAN_POINT ( 'NONE',  ( 11.74264578624800315, -36.14014761921581709, -3.400000000000000355 ) ) ;
#169113=CIRCLE ( 'NONE', #162637, 10.00000000000000888 ) ;
#169124=ORIENTED_EDGE ( 'NONE', *, *, #91315, .T. ) ;
#169126=CARTESIAN_POINT ( 'NONE',  ( 21.18879603623556918, -31.24179269221876254, -19.75583340878575456 ) ) ;
#169159=CARTESIAN_POINT ( 'NONE',  ( -29.86685920354755197, -21.69954338932560134, -10.42499999726881299 ) ) ;
#169160=ORIENTED_EDGE ( 'NONE', *, *, #31320, .F. ) ;
#169193=DIRECTION ( 'NONE',  ( -0.000000000000000000, -0.000000000000000000, -1.000000000000000000 ) ) ;
#169243=CARTESIAN_POINT ( 'NONE',  ( 14.62261807015722859, 16.01221511231801031, -56.20577350945247730 ) ) ;
#169261=AXIS2_PLACEMENT_3D ( 'NONE', #181316, #137760, #104457 ) ;
#169294=CARTESIAN_POINT ( 'NONE',  ( -10.70342273063628014, -35.99563703666770920, -30.86961840752219288 ) ) ;
#169317=CARTESIAN_POINT ( 'NONE',  ( -23.48529157249599919, -32.32473071737749848, -9.699999999999999289 ) ) ;
#169325=CARTESIAN_POINT ( 'NONE',  ( -27.86273085795036408, -28.69962071417357663, -25.00000000000000000 ) ) ;
#169353=CARTESIAN_POINT ( 'NONE',  ( -4.647474457565486646E-15, 28.90000000000004476, -65.00100000000003320 ) ) ;
#169521=EDGE_LOOP ( 'NONE', ( #149348, #16045, #78692, #111353 ) ) ;
#169556=DIRECTION ( 'NONE',  ( -0.000000000000000000, -0.000000000000000000, 1.000000000000000000 ) ) ;
#169574=CARTESIAN_POINT ( 'NONE',  ( -0.7844626028949902574, -13.90528855463213631, -60.35633530387644896 ) ) ;
#169580=DIRECTION ( 'NONE',  ( 1.000000000000000000, 0.000000000000000000, 0.000000000000000000 ) ) ;
#169595=CARTESIAN_POINT ( 'NONE',  ( -36.91746825000001309, 11.99521256947798342, -5.224999997268811924 ) ) ;
#169620=CARTESIAN_POINT ( 'NONE',  ( -21.35939100396076995, 0.4315818942740129449, -58.81718527612538594 ) ) ;
#169625=CIRCLE ( 'NONE', #21101, 31.90000000000003411 ) ;
#169641=ORIENTED_EDGE ( 'NONE', *, *, #67633, .T. ) ;
#169648=DIRECTION ( 'NONE',  ( -0.000000000000000000, -0.000000000000000000, 1.000000000000000000 ) ) ;
#169656=CARTESIAN_POINT ( 'NONE',  ( -11.95480631804128002, 11.66256017358944064, -61.34707691135564289 ) ) ;
#169699=AXIS2_PLACEMENT_3D ( 'NONE', #109216, #1031, #62703 ) ;
#169763=EDGE_LOOP ( 'NONE', ( #87095, #42289, #133998, #176295 ) ) ;
#169772=CARTESIAN_POINT ( 'NONE',  ( 0.7625336781875722281, 6.293144983425331240, -62.46804555434153627 ) ) ;
#169796=CARTESIAN_POINT ( 'NONE',  ( -22.34286686445884840, 20.24680444626648068, -48.12863666802710583 ) ) ;
#169810=( BOUNDED_CURVE ( )  B_SPLINE_CURVE ( 2, ( #65242, #126902, #18759, #5551, #188608, #128888, #80406, #67230, #99560, #50089, #176428 ),
 .UNSPECIFIED., .F., .T. ) 
 B_SPLINE_CURVE_WITH_KNOTS ( ( 3, 2, 2, 2, 2, 3 ),
 ( 0.1000000000000000056, 0.1199999999999999956, 0.1400000000000000133, 0.1600000000000000033, 0.1799999999999999933, 0.2000000000000000111 ),
 .UNSPECIFIED. ) 
 CURVE ( )  GEOMETRIC_REPRESENTATION_ITEM ( )  RATIONAL_B_SPLINE_CURVE ( ( 1.000000000000000000, 0.9510565162951535312, 1.000000000000000000, 0.9510565162951535312, 1.000000000000000000, 0.9510565162951535312, 1.000000000000000000, 0.9510565162951535312, 1.000000000000000000, 0.9510565162951535312, 1.000000000000000000 ) ) 
 REPRESENTATION_ITEM ( '' )  );
#169845=CARTESIAN_POINT ( 'NONE',  ( 22.44763431097445761, -1.469699867061888376, -58.07555020237585097 ) ) ;
#169863=CIRCLE ( 'NONE', #111699, 216.0437394197456911 ) ;
#169890=CARTESIAN_POINT ( 'NONE',  ( -4.384086992840744657, 4.242615737635153650, -64.53213882399992940 ) ) ;
#169896=CARTESIAN_POINT ( 'NONE',  ( -8.839334217631824586, -46.13630234914189288, -24.17074550867520344 ) ) ;
#169936=DIRECTION ( 'NONE',  ( -0.000000000000000000, 0.000000000000000000, 1.000000000000000000 ) ) ;
#169954=CARTESIAN_POINT ( 'NONE',  ( -28.90000000000004476, 2.980639576201346218E-13, -64.92279855667830191 ) ) ;
#169968=DIRECTION ( 'NONE',  ( -0.000000000000000000, -0.000000000000000000, -1.000000000000000000 ) ) ;
#170016=EDGE_CURVE ( 'NONE', #196503, #14377, #37692, .T. ) ;
#170086=CARTESIAN_POINT ( 'NONE',  ( 15.38830714838548452, -1.491100297015996556, -59.71292413584865244 ) ) ;
#170096=CARTESIAN_POINT ( 'NONE',  ( -17.06172130128252462, 14.93915603648724399, -57.95097928225586514 ) ) ;
#170098=EDGE_CURVE ( 'NONE', #22834, #44025, #88188, .T. ) ;
#170131=CARTESIAN_POINT ( 'NONE',  ( 12.97112549082123678, -41.39484261838032353, -20.61933656601679132 ) ) ;
#170223=CARTESIAN_POINT ( 'NONE',  ( 0.5037075166051908637, 31.83037104268352024, -49.22065939777928634 ) ) ;
#170238=DIRECTION ( 'NONE',  ( 1.000000000000000000, 0.000000000000000000, 0.000000000000000000 ) ) ;
#170250=CARTESIAN_POINT ( 'NONE',  ( 2.500000000000000000, 0.000000000000000000, -64.92179855667829713 ) ) ;
#170287=VERTEX_POINT ( 'NONE', #47564 ) ;
#170299=CARTESIAN_POINT ( 'NONE',  ( -19.65168359646841978, -34.19331532915863647, -17.88087567707375314 ) ) ;
#170347=EDGE_LOOP ( 'NONE', ( #93302, #141756, #103721, #28585, #42985 ) ) ;
#170359=CARTESIAN_POINT ( 'NONE',  ( 25.17999522921048694, -30.53243704067885034, -18.89073929087368597 ) ) ;
#170379=ORIENTED_EDGE ( 'NONE', *, *, #73495, .F. ) ;
#170417=CARTESIAN_POINT ( 'NONE',  ( -6.020228577223754586E-15, 39.95556452105416412, -2.500000000000000000 ) ) ;
#170466=DIRECTION ( 'NONE',  ( -0.000000000000000000, -0.000000000000000000, 1.000000000000000000 ) ) ;
#170492=B_SPLINE_CURVE_WITH_KNOTS ( 'NONE', 3,
 ( #183555, #45041, #152215, #140004, #106699, #185532, #62170, #13699, #91505, #124850, #186550, #61182, #77351, #139018, #168372, #121863 ),
 .UNSPECIFIED., .F., .F.,
 ( 4, 2, 2, 2, 2, 2, 2, 4 ),
 ( 0.001189573402565897910, 0.002113295908917162298, 0.002575157162092795576, 0.003037018415268428854, 0.003498879668444062133, 0.003960740921619694543, 0.004422602174795328689, 0.004884463427970961967 ),
 .UNSPECIFIED. ) ;
#170515=EDGE_CURVE ( 'NONE', #198657, #22834, #167136, .T. ) ;
#170526=ORIENTED_EDGE ( 'NONE', *, *, #158176, .T. ) ;
#170549=B_SPLINE_CURVE_WITH_KNOTS ( 'NONE', 3,
 ( #153081, #61069, #142873, #50882, #19547, #190392, #6350, #84184, #96369, #35703 ),
 .UNSPECIFIED., .F., .F.,
 ( 4, 2, 2, 2, 4 ),
 ( 2.778238173776314926E-07, 0.0003233481720886709990, 0.0006464185203599643768, 0.0009694888686312577546, 0.001292559216902551241 ),
 .UNSPECIFIED. ) ;
#170574=FACE_BOUND ( 'NONE', #194805, .T. ) ;
#170580=CARTESIAN_POINT ( 'NONE',  ( -7.600000000000007638, 7.873841278763511268E-14, -64.92279855667830191 ) ) ;
#170585=ADVANCED_FACE ( 'NONE', ( #16228 ), #77880, .T. ) ;
#170592=DIRECTION ( 'NONE',  ( -0.000000000000000000, -0.000000000000000000, 1.000000000000000000 ) ) ;
#170596=CARTESIAN_POINT ( 'NONE',  ( 29.86685920354754487, 21.69954338932564752, -3.924999997268812990 ) ) ;
#170633=CARTESIAN_POINT ( 'NONE',  ( -38.00000000000000711, 2.428612866367529932E-14, -8.000000000000000000 ) ) ;
#170640=ORIENTED_EDGE ( 'NONE', *, *, #103959, .F. ) ;
#170644=CARTESIAN_POINT ( 'NONE',  ( -30.74264578624800492, -22.33583958711396278, -11.54999999453762527 ) ) ;
#170647=CARTESIAN_POINT ( 'NONE',  ( -36.91746825000001309, 11.99521256947798342, -1.224999997268813035 ) ) ;
#170670=CARTESIAN_POINT ( 'NONE',  ( -33.17138627372819570, -22.14683228596885911, -20.77970695691874070 ) ) ;
#170772=CARTESIAN_POINT ( 'NONE',  ( 1.490396665426041878, 7.404744102125047966, -62.24188859777813576 ) ) ;
#170797=CARTESIAN_POINT ( 'NONE',  ( 6.575277882517920780, -6.294065535077253415, -61.89430850415822505 ) ) ;
#170825=ADVANCED_FACE ( 'NONE', ( #37351 ), #94553, .F. ) ;
#170834=CARTESIAN_POINT ( 'NONE',  ( -8.516083024820087388, 1.203758653825318881, -62.01440738234571626 ) ) ;
#170841=AXIS2_PLACEMENT_3D ( 'NONE', #109163, #198205, #59676 ) ;
#170866=ORIENTED_EDGE ( 'NONE', *, *, #98810, .T. ) ;
#170929=DIRECTION ( 'NONE',  ( 1.000000000000000000, 0.000000000000000000, 0.000000000000000000 ) ) ;
#170949=CYLINDRICAL_SURFACE ( 'NONE', #146256, 38.00000000000000000 ) ;
#171043=ORIENTED_EDGE ( 'NONE', *, *, #182123, .F. ) ;
#171076=FACE_OUTER_BOUND ( 'NONE', #8976, .T. ) ;
#171093=CYLINDRICAL_SURFACE ( 'NONE', #30294, 38.00000000000000000 ) ;
#171129=CARTESIAN_POINT ( 'NONE',  ( 21.90755247610641021, -31.73190472514349381, -17.16613178567241960 ) ) ;
#171133=VERTEX_POINT ( 'NONE', #64480 ) ;
#171147=CIRCLE ( 'NONE', #138810, 8.000000000000000000 ) ;
#171162=ORIENTED_EDGE ( 'NONE', *, *, #60543, .F. ) ;
#171199=CARTESIAN_POINT ( 'NONE',  ( 6.941592873960390264, -1.351304681146071829, -62.33628431810817716 ) ) ;
#171215=CARTESIAN_POINT ( 'NONE',  ( 0.000000000000000000, 0.000000000000000000, -52.65483682830183199 ) ) ;
#171243=CARTESIAN_POINT ( 'NONE',  ( 30.74264578624800137, -22.33583958711395212, -7.200000000000001066 ) ) ;
#171245=CARTESIAN_POINT ( 'NONE',  ( -20.10096181552316708, -22.06460587353105751, -51.62975016085093927 ) ) ;
#171282=EDGE_CURVE ( 'NONE', #16960, #179364, #128273, .T. ) ;
#171283=VERTEX_POINT ( 'NONE', #129746 ) ;
#171299=CARTESIAN_POINT ( 'NONE',  ( -28.03896471500539889, -25.30868469084938965, -20.82118626251310189 ) ) ;
#171317=CARTESIAN_POINT ( 'NONE',  ( 0.000000000000000000, 0.000000000000000000, -64.92279855667830191 ) ) ;
#171321=CARTESIAN_POINT ( 'NONE',  ( 20.51075850018421676, -20.36001345239828808, -49.67367017693149478 ) ) ;
#171329=CARTESIAN_POINT ( 'NONE',  ( 6.434671708797586653, 6.434671708797580436, -61.89430850415821794 ) ) ;
#171338=DIRECTION ( 'NONE',  ( 1.000000000000000000, 0.000000000000000000, 0.000000000000000000 ) ) ;
#171347=CARTESIAN_POINT ( 'NONE',  ( 36.91746824999999887, 11.99521256947799053, -3.524999997268813079 ) ) ;
#171356=DIRECTION ( 'NONE',  ( -0.000000000000000000, -0.000000000000000000, 1.000000000000000000 ) ) ;
#171358=CARTESIAN_POINT ( 'NONE',  ( 27.19415581439775664, -28.92630772671044070, -20.12198987529614058 ) ) ;
#171372=ADVANCED_FACE ( 'NONE', ( #6413 ), #50787, .T. ) ;
#171378=ORIENTED_EDGE ( 'NONE', *, *, #78423, .F. ) ;
#171407=PLANE ( 'NONE',  #51241 ) ;
#171551=CARTESIAN_POINT ( 'NONE',  ( -30.74264578624800492, -22.33583958711396278, -5.800000000000000711 ) ) ;
#171564=( BOUNDED_SURFACE ( )  B_SPLINE_SURFACE ( 3, 2, ( 
 ( #28891, #92509, #27906 ),
 ( #90531, #30862, #165412 ),
 ( #61180, #495, #122852 ),
 ( #182565, #184540, #59196 ),
 ( #152213, #88548, #44048 ),
 ( #46020, #154198, #15688 ),
 ( #77349, #62168, #196755 ),
 ( #123832, #103732, #42068 ),
 ( #119891, #167395, #43054 ),
 ( #104720, #89549, #151235 ),
 ( #12724, #13697, #75364 ),
 ( #137034, #4459, #142981 ),
 ( #33832, #155190, #158164 ),
 ( #34821, #93504, #49998 ),
 ( #156178, #49008, #5465 ),
 ( #185530, #67147, #17677 ),
 ( #32846, #110663, #48020 ),
 ( #157178, #111663, #96476 ),
 ( #159143, #16680, #47022 ),
 ( #141991, #1491, #78329 ),
 ( #20640, #35811, #82293 ),
 ( #19656, #3479, #81297 ),
 ( #173350, #140002, #79335 ),
 ( #18672, #126815, #141005 ),
 ( #143984, #172343, #66148 ),
 ( #65156, #2493, #108681 ),
 ( #95492, #170359, #31851 ),
 ( #80318, #97457, #63169 ),
 ( #124848, #188521, #186548 ),
 ( #127811, #109677, #171358 ),
 ( #125839, #189516, #94496 ),
 ( #50989, #64174, #187541 ),
 ( #112649, #174341, #117654 ),
 ( #9488, #163158, #113636 ),
 ( #160157, #193502, #38817 ),
 ( #36798, #55977, #130809 ),
 ( #70152, #98463, #131822 ),
 ( #51978, #83301, #179351 ),
 ( #162154, #24661, #7458 ),
 ( #54980, #114642, #21648 ),
 ( #85298, #8477, #40814 ),
 ( #102484, #175331, #164171 ),
 ( #25669, #86310, #177346 ),
 ( #147999, #145976, #144977 ) ),
 .UNSPECIFIED., .F., .F., .T. ) 
 B_SPLINE_SURFACE_WITH_KNOTS ( ( 4, 2, 2, 2, 2, 2, 2, 2, 2, 2, 2, 2, 2, 2, 2, 2, 2, 2, 2, 2, 2, 4 ),
 ( 3, 3 ),
 ( 0.1334715276261013994, 0.1400397817209069751, 0.1416818452446083620, 0.1433239087683097490, 0.1466080358157125230, 0.1498921628631152969, 0.1531762899105180986, 0.1564604169579209003, 0.1597445440053236743, 0.1630286710527264482, 0.1646707345764278352, 0.1663127981001292222, 0.1679548616238306091, 0.1695969251475319961, 0.1712389886712333831, 0.1720600204330841043, 0.1728810521949347978, 0.1745231157186362125, 0.1761651792423375995, 0.1794493062897403735, 0.1827334333371431474, 0.1860175603845459213 ),
 ( 0.000000000000000000, 1.000000000000000000 ),
 .UNSPECIFIED. ) 
 GEOMETRIC_REPRESENTATION_ITEM ( )  RATIONAL_B_SPLINE_SURFACE ( (
 ( 1.000000000000000000, 0.7745966692414832933, 1.000000000000000000),
 ( 1.000000000000000000, 0.7873173169476441746, 1.000000000000000000),
 ( 1.000000000000000000, 0.8012080269091598206, 1.000000000000000000),
 ( 1.000000000000000000, 0.8197272276933330604, 1.000000000000000000),
 ( 1.000000000000000000, 0.8234885421912105929, 1.000000000000000000),
 ( 1.000000000000000000, 0.8311157573376537488, 1.000000000000000000),
 ( 1.000000000000000000, 0.8349728938257902078, 1.000000000000000000),
 ( 1.000000000000000000, 0.8465302108188730301, 1.000000000000000000),
 ( 1.000000000000000000, 0.8542644918355096761, 1.000000000000000000),
 ( 1.000000000000000000, 0.8696747091110100802, 1.000000000000000000),
 ( 1.000000000000000000, 0.8773507960691678820, 1.000000000000000000),
 ( 1.000000000000000000, 0.8925002889089019842, 1.000000000000000000),
 ( 1.000000000000000000, 0.8999891582782626465, 1.000000000000000000),
 ( 1.000000000000000000, 0.9145203485640005514, 1.000000000000000000),
 ( 1.000000000000000000, 0.9215166741120213167, 1.000000000000000000),
 ( 1.000000000000000000, 0.9348196634156189511, 1.000000000000000000),
 ( 1.000000000000000000, 0.9411264847296241243, 1.000000000000000000),
 ( 1.000000000000000000, 0.9528821887672445090, 1.000000000000000000),
 ( 1.000000000000000000, 0.9583320463343933948, 1.000000000000000000),
 ( 1.000000000000000000, 0.9657141226242612619, 1.000000000000000000),
 ( 1.000000000000000000, 0.9680424144921332408, 1.000000000000000000),
 ( 1.000000000000000000, 0.9724014971077671321, 1.000000000000000000),
 ( 1.000000000000000000, 0.9744334801158450743, 1.000000000000000000),
 ( 1.000000000000000000, 0.9781204877085362126, 1.000000000000000000),
 ( 1.000000000000000000, 0.9797809101336113491, 1.000000000000000000),
 ( 1.000000000000000000, 0.9826818083352578670, 1.000000000000000000),
 ( 1.000000000000000000, 0.9839230189806438265, 1.000000000000000000),
 ( 1.000000000000000000, 0.9859013487405716702, 1.000000000000000000),
 ( 1.000000000000000000, 0.9866146582094302842, 1.000000000000000000),
 ( 1.000000000000000000, 0.9872250220265940124, 1.000000000000000000),
 ( 1.000000000000000000, 0.9873522598263766437, 1.000000000000000000),
 ( 1.000000000000000000, 0.9874472609175324322, 1.000000000000000000),
 ( 1.000000000000000000, 0.9874138636738800656, 1.000000000000000000),
 ( 1.000000000000000000, 0.9870735186574125519, 1.000000000000000000),
 ( 1.000000000000000000, 0.9865315217160959271, 1.000000000000000000),
 ( 1.000000000000000000, 0.9848873008857480515, 1.000000000000000000),
 ( 1.000000000000000000, 0.9837743821442975767, 1.000000000000000000),
 ( 1.000000000000000000, 0.9797976954002131089, 1.000000000000000000),
 ( 1.000000000000000000, 0.9763000371664239951, 1.000000000000000000),
 ( 1.000000000000000000, 0.9680363503267302994, 1.000000000000000000),
 ( 1.000000000000000000, 0.9632464763794107432, 1.000000000000000000),
 ( 1.000000000000000000, 0.9526889542240987163, 1.000000000000000000),
 ( 1.000000000000000000, 0.9469283804591228648, 1.000000000000000000),
 ( 1.000000000000000000, 0.9407878411039234390, 1.000000000000000000) ) ) 
 REPRESENTATION_ITEM ( '' )  SURFACE ( )  );
#171586=ORIENTED_EDGE ( 'NONE', *, *, #116496, .T. ) ;
#171588=CARTESIAN_POINT ( 'NONE',  ( 0.000000000000000000, 0.000000000000000000, -64.92279855667830191 ) ) ;
#171592=CARTESIAN_POINT ( 'NONE',  ( -36.91746825000001309, -11.99521256947794789, -11.02499999726881263 ) ) ;
#171640=CARTESIAN_POINT ( 'NONE',  ( -11.40812507854755609, 35.11059874428196537, -7.524999997268813523 ) ) ;
#171648=CARTESIAN_POINT ( 'NONE',  ( -9.687362902255733488, 9.687362902255692632, -62.58071313852362039 ) ) ;
#171664=VERTEX_POINT ( 'NONE', #14403 ) ;
#171681=B_SPLINE_CURVE_WITH_KNOTS ( 'NONE', 3,
 ( #147560, #40372, #196079, #134393, #88866, #43365, #9045, #72720, #104042, #132383, #55539, #163730, #148556, #195065, #56545, #12058, #197063, #135393, #41379, #58531, #95563, #19726, #143051, #172418, #80391, #81367 ),
 .UNSPECIFIED., .F., .F.,
 ( 4, 2, 2, 2, 2, 2, 2, 2, 2, 2, 2, 2, 4 ),
 ( 1.971416326048476669E-07, 0.0002960211146592905160, 0.0005918450876859761246, 0.0008876690607126617874, 0.001183493033739347559, 0.001775140979792719318, 0.002366788925846091077, 0.002662612898872771753, 0.002958436871899451995, 0.003254260844926132237, 0.003550084817952812912, 0.004141732764006173829, 0.004733380710059535181 ),
 .UNSPECIFIED. ) ;
#171723=ADVANCED_FACE ( 'NONE', ( #168087 ), #212, .T. ) ;
#171777=AXIS2_PLACEMENT_3D ( 'NONE', #68710, #192064, #69720 ) ;
#171794=CARTESIAN_POINT ( 'NONE',  ( -23.51385019162032819, 1.374935097489404123, -54.82293943248598822 ) ) ;
#171824=VERTEX_POINT ( 'NONE', #105424 ) ;
#171850=LINE ( 'NONE', #153691, #20707 ) ;
#171861=EDGE_LOOP ( 'NONE', ( #6118, #89294, #58891, #33636 ) ) ;
#171883=EDGE_CURVE ( 'NONE', #145198, #166185, #83094, .T. ) ;
#171893=DIRECTION ( 'NONE',  ( 0.9974398506828145994, 0.07151044867601362431, 4.325705812135698390E-17 ) ) ;
#171962=CARTESIAN_POINT ( 'NONE',  ( -5.801314085210285576, -6.819390806090331658, -61.93051126003076945 ) ) ;
#171991=CARTESIAN_POINT ( 'NONE',  ( -24.30000000000003268, 2.668083032619853614E-13, -56.77278709839600879 ) ) ;
#172037=ORIENTED_EDGE ( 'NONE', *, *, #80739, .F. ) ;
#172040=VERTEX_POINT ( 'NONE', #79047 ) ;
#172051=CARTESIAN_POINT ( 'NONE',  ( 1.227931366032057224E-14, 24.30000000000003268, -54.21489346206828230 ) ) ;
#172069=FACE_OUTER_BOUND ( 'NONE', #196300, .T. ) ;
#172078=CARTESIAN_POINT ( 'NONE',  ( 3.735172737399431091E-16, 6.100000000000006750, -65.00100000000003320 ) ) ;
#172082=CARTESIAN_POINT ( 'NONE',  ( 17.62203461105333702, -16.21435693443512704, -57.04011861108771342 ) ) ;
#172097=CARTESIAN_POINT ( 'NONE',  ( 30.74264578624800137, -22.33583958711395212, -9.199999999999999289 ) ) ;
#172106=ORIENTED_EDGE ( 'NONE', *, *, #58993, .T. ) ;
#172113=EDGE_CURVE ( 'NONE', #183247, #62967, #79799, .T. ) ;
#172121=CARTESIAN_POINT ( 'NONE',  ( 10.70342273063187122, -35.99563703666952819, -30.86961840751871478 ) ) ;
#172187=CARTESIAN_POINT ( 'NONE',  ( 9.090072183657238014, -0.1985533113405552330, -61.89635373339111624 ) ) ;
#172208=CARTESIAN_POINT ( 'NONE',  ( 0.000000000000000000, -165.0000000000000000, 12.00000000000000355 ) ) ;
#172232=CARTESIAN_POINT ( 'NONE',  ( 37.99999999999996447, -12.34694845685046793, -7.100000000000002309 ) ) ;
#172234=CARTESIAN_POINT ( 'NONE',  ( 4.999999999999999112, 5.000000000000000888, -18.00000000000000000 ) ) ;
#172307=CARTESIAN_POINT ( 'NONE',  ( 8.388830574159379737E-16, 13.70000000000001528, -62.58071313852362039 ) ) ;
#172310=CARTESIAN_POINT ( 'NONE',  ( 3.948644494436277075, 4.896406352259362826, -64.50244604205114740 ) ) ;
#172324=CARTESIAN_POINT ( 'NONE',  ( -37.66961640367473052, -4.999999999999976019, -25.00000000000000000 ) ) ;
#172333=CARTESIAN_POINT ( 'NONE',  ( 3.556970738554033499E-15, -38.81732327939057825, -6.124999997268812280 ) ) ;
#172343=CARTESIAN_POINT ( 'NONE',  ( 24.05628303387030797, -31.51879896406492065, -19.31700871831125710 ) ) ;
#172361=ORIENTED_EDGE ( 'NONE', *, *, #45144, .T. ) ;
#172389=AXIS2_PLACEMENT_3D ( 'NONE', #178436, #42910, #180450 ) ;
#172393=CARTESIAN_POINT ( 'NONE',  ( -17.18269478283327345, -17.18269478283298568, -54.21489346206828230 ) ) ;
#172397=CARTESIAN_POINT ( 'NONE',  ( -11.40812507854755609, 35.11059874428196537, -3.024999997268813523 ) ) ;
#172398=CARTESIAN_POINT ( 'NONE',  ( 30.74264578624799782, 22.33583958711400541, -2.549999994537626602 ) ) ;
#172418=CARTESIAN_POINT ( 'NONE',  ( -0.3964520562363653688, -6.139823915386825703, -64.52448473163052256 ) ) ;
#172432=CARTESIAN_POINT ( 'NONE',  ( 12.06170956654727355, -11.49862171186262039, -61.36395269087611126 ) ) ;
#172449=AXIS2_PLACEMENT_3D ( 'NONE', #119639, #150979, #135805 ) ;
#172509=VECTOR ( 'NONE', #87397, 1000.000000000000000 ) ;
#172517=ORIENTED_EDGE ( 'NONE', *, *, #91512, .F. ) ;
#172546=CARTESIAN_POINT ( 'NONE',  ( 23.48529157249600630, -32.32473071737748427, -5.299999999999999822 ) ) ;
#172566=CARTESIAN_POINT ( 'NONE',  ( 0.000000000000000000, 0.000000000000000000, -25.00000000000000000 ) ) ;
#172572=CARTESIAN_POINT ( 'NONE',  ( 1.500000000000335065, 22.62084519560232465, -57.95595451695638900 ) ) ;
#172580=ORIENTED_EDGE ( 'NONE', *, *, #140897, .F. ) ;
#172582=LINE ( 'NONE', #35053, #188332 ) ;
#172585=CARTESIAN_POINT ( 'NONE',  ( 22.81625015709510151, -31.40387420917324590, -8.424999997268812990 ) ) ;
#172586=AXIS2_PLACEMENT_3D ( 'NONE', #86398, #151078, #41911 ) ;
#172633=CARTESIAN_POINT ( 'NONE',  ( -36.91746825000001309, -11.99521256947794789, -5.024999997268813523 ) ) ;
#172641=CARTESIAN_POINT ( 'NONE',  ( -11.94381442052175757, 9.822853212439014214, -61.89036147510174146 ) ) ;
#172724=DIRECTION ( 'NONE',  ( 1.000000000000000000, 0.000000000000000000, 0.000000000000000000 ) ) ;
#172726=DIRECTION ( 'NONE',  ( -0.000000000000000000, -0.000000000000000000, 1.000000000000000000 ) ) ;
#172728=CIRCLE ( 'NONE', #150240, 59.99999999999998579 ) ;
#172766=AXIS2_PLACEMENT_3D ( 'NONE', #140974, #2462, #51948 ) ;
#172793=CARTESIAN_POINT ( 'NONE',  ( -9.616112110649096323, -9.758613693862333349, -60.44446360152742415 ) ) ;
#172825=CIRCLE ( 'NONE', #72676, 12.00000000000000178 ) ;
#172829=CARTESIAN_POINT ( 'NONE',  ( 38.00000000000000000, 12.34694845685046616, -2.649999994537626247 ) ) ;
#172839=CARTESIAN_POINT ( 'NONE',  ( 23.16108095314134019, -1.467328942210885279, -57.58004187413772712 ) ) ;
#172841=CARTESIAN_POINT ( 'NONE',  ( -1.355922687059376797, -31.06299995236813416, -50.16575868250043868 ) ) ;
#172861=ORIENTED_EDGE ( 'NONE', *, *, #120148, .F. ) ;
#172879=CIRCLE ( 'NONE', #14695, 10.00000000000000000 ) ;
#172896=CARTESIAN_POINT ( 'NONE',  ( 69.65682714487590488, -71.74905178543389184, -25.00000000000000000 ) ) ;
#172898=EDGE_CURVE ( 'NONE', #143487, #36546, #135131, .T. ) ;
#172930=FACE_OUTER_BOUND ( 'NONE', #91430, .T. ) ;
#172944=CIRCLE ( 'NONE', #92246, 9.100000000000001421 ) ;
#172951=CARTESIAN_POINT ( 'NONE',  ( 13.70000000000001528, -4.867217739956692332E-14, -62.58071313852362039 ) ) ;
#172993=CARTESIAN_POINT ( 'NONE',  ( -0.3431728551240714742, -71.74905178543389184, -15.00000000000000178 ) ) ;
#173047=DIRECTION ( 'NONE',  ( -1.000000000000000000, 0.000000000000000000, -5.204170427930421283E-16 ) ) ;
#173057=CARTESIAN_POINT ( 'NONE',  ( 13.74234921310041457, -0.4081324879001385630, -62.56359473395606585 ) ) ;
#173085=FACE_BOUND ( 'NONE', #14992, .T. ) ;
#173098=EDGE_LOOP ( 'NONE', ( #157102, #192252, #39816, #18904, #46768, #173909, #134388, #30423, #115591, #103611, #103511, #105399, #4228 ) ) ;
#173125=CARTESIAN_POINT ( 'NONE',  ( 29.33118895280741256, -23.95254016166647304, -21.73655181066850162 ) ) ;
#173153=VERTEX_POINT ( 'NONE', #101775 ) ;
#173185=CARTESIAN_POINT ( 'NONE',  ( -4.999999999999996447, 5.000000000000003553, -18.00000000000000000 ) ) ;
#173204=APPLICATION_CONTEXT ( 'automotive_design' ) ;
#173210=CARTESIAN_POINT ( 'NONE',  ( -19.97888994334924817, -34.65319547504298470, -5.000000000000000000 ) ) ;
#173234=CARTESIAN_POINT ( 'NONE',  ( -23.48529157249599919, -32.32473071737749848, -7.699999999999999289 ) ) ;
#173238=VECTOR ( 'NONE', #73921, 1000.000000000000000 ) ;
#173264=EDGE_CURVE ( 'NONE', #15377, #190965, #54118, .T. ) ;
#173272=ORIENTED_EDGE ( 'NONE', *, *, #90391, .T. ) ;
#173288=EDGE_CURVE ( 'NONE', #76043, #58799, #138033, .T. ) ;
#173290=CARTESIAN_POINT ( 'NONE',  ( -25.66183622254775898, -27.84411637527858119, -16.56099493762688724 ) ) ;
#173320=CARTESIAN_POINT ( 'NONE',  ( 22.84593195647081387, -20.82949652188557010, -50.38176470501583992 ) ) ;
#173339=CARTESIAN_POINT ( 'NONE',  ( -5.950531402560715689E-15, 38.81732327939063509, -3.124999997268813168 ) ) ;
#173350=CARTESIAN_POINT ( 'NONE',  ( 22.61240241994758904, -33.77560033877482937, -17.98683046886793591 ) ) ;
#173401=CARTESIAN_POINT ( 'NONE',  ( -29.86685920354755197, -21.69954338932560134, -8.924999997268812990 ) ) ;
#173402=CARTESIAN_POINT ( 'NONE',  ( -6.020228577223754586E-15, 39.95556452105416412, -2.249999994537626336 ) ) ;
#173429=DIRECTION ( 'NONE',  ( 1.000000000000000000, 0.000000000000000000, 0.000000000000000000 ) ) ;
#173437=CARTESIAN_POINT ( 'NONE',  ( 31.06299995236814837, -1.355922687059476051, -50.16575868250042447 ) ) ;
#173448=CARTESIAN_POINT ( 'NONE',  ( -3.735172737399431091E-16, -6.100000000000006750, -64.53213882399991519 ) ) ;
#173468=ORIENTED_EDGE ( 'NONE', *, *, #159157, .T. ) ;
#173564=CARTESIAN_POINT ( 'NONE',  ( 0.000000000000000000, 0.000000000000000000, -62.50719930893269805 ) ) ;
#173568=FACE_BOUND ( 'NONE', #129102, .T. ) ;
#173574=CARTESIAN_POINT ( 'NONE',  ( 7.086465707319022428E-15, -78.65691688641808810, -25.00000000000000000 ) ) ;
#173580=EDGE_LOOP ( 'NONE', ( #191709, #137263, #175803, #2512 ) ) ;
#173588=CARTESIAN_POINT ( 'NONE',  ( -22.81625015709510507, 31.40387420917330275, -7.424999997268812990 ) ) ;
#173623=CARTESIAN_POINT ( 'NONE',  ( -30.74264578624800492, 22.33583958711400186, -8.200000000000001066 ) ) ;
#173634=ADVANCED_FACE ( 'NONE', ( #2552 ), #168427, .F. ) ;
#173638=CARTESIAN_POINT ( 'NONE',  ( 36.91746825000000598, -11.99521256947793546, -4.224999997268812812 ) ) ;
#173645=FACE_OUTER_BOUND ( 'NONE', #161959, .T. ) ;
#173655=VERTEX_POINT ( 'NONE', #48078 ) ;
#173715=ORIENTED_EDGE ( 'NONE', *, *, #40462, .F. ) ;
#173787=CARTESIAN_POINT ( 'NONE',  ( -193.3062444957834884, -155.7167183371838064, -15.00000000000000178 ) ) ;
#173794=CARTESIAN_POINT ( 'NONE',  ( -9.248023074035629065, -10.55781631604391890, -60.31354024882315912 ) ) ;
#173803=EDGE_CURVE ( 'NONE', #11421, #167693, #150098, .T. ) ;
#173811=CARTESIAN_POINT ( 'NONE',  ( 15.06137443927351072, -15.06137443927345210, -56.46919128290398504 ) ) ;
#173827=CARTESIAN_POINT ( 'NONE',  ( 31.65755289763031044, -24.31906878930446680, -22.32084141216706286 ) ) ;
#173842=CARTESIAN_POINT ( 'NONE',  ( 30.07467525274878994, -23.10311534983925696, -22.45479934155872215 ) ) ;
#173896=CARTESIAN_POINT ( 'NONE',  ( -7.587788125975658993, -46.88744275388931726, -24.49805083758699098 ) ) ;
#173908=CARTESIAN_POINT ( 'NONE',  ( 9.614343725828573994, 9.760382078682853901, -62.58071313852360618 ) ) ;
#173909=ORIENTED_EDGE ( 'NONE', *, *, #191135, .F. ) ;
#173928=CARTESIAN_POINT ( 'NONE',  ( -15.38891197842625225, 1.491051326733042082, -61.89130710690761106 ) ) ;
#173989=CARTESIAN_POINT ( 'NONE',  ( -11.02000550219323216, -37.94488912280210968, -31.28304700362893698 ) ) ;
#174022=CYLINDRICAL_SURFACE ( 'NONE', #80496, 1.499999999999994449 ) ;
#174071=CARTESIAN_POINT ( 'NONE',  ( 9.687362902255724606, 9.687362902255701513, -60.44446360152740993 ) ) ;
#174073=PLANE ( 'NONE',  #12177 ) ;
#174077=CARTESIAN_POINT ( 'NONE',  ( 29.09442113371785865, -27.25731168736310295, -16.99878707713621395 ) ) ;
#174083=CARTESIAN_POINT ( 'NONE',  ( 17.43248706301297091, -16.85888939060687264, -56.81032385587572264 ) ) ;
#174095=ORIENTED_EDGE ( 'NONE', *, *, #120673, .T. ) ;
#174120=CARTESIAN_POINT ( 'NONE',  ( 27.75745401094703269, -25.59313184531724161, -20.67669038789624736 ) ) ;
#174148=ORIENTED_EDGE ( 'NONE', *, *, #144467, .T. ) ;
#174182=CIRCLE ( 'NONE', #45021, 214.0437394197456342 ) ;
#174271=VERTEX_POINT ( 'NONE', #128862 ) ;
#174284=CARTESIAN_POINT ( 'NONE',  ( -24.48191864108932592, -29.02791343562081394, -16.65471697698749409 ) ) ;
#174300=EDGE_LOOP ( 'NONE', ( #184936, #195638, #185696, #1266 ) ) ;
#174307=CARTESIAN_POINT ( 'NONE',  ( -29.03295818733087330, 0.6278704076488079711, -49.50940399778497181 ) ) ;
#174315=CARTESIAN_POINT ( 'NONE',  ( 22.44948314067158890, -20.33105923352922773, -51.12866626710398776 ) ) ;
#174325=CIRCLE ( 'NONE', #125975, 69.99999999999997158 ) ;
#174331=CARTESIAN_POINT ( 'NONE',  ( -36.91746825000001309, 11.99521256947798342, -4.724999997268811924 ) ) ;
#174341=CARTESIAN_POINT ( 'NONE',  ( 27.73791293434951655, -28.12602025316063603, -18.50562026186076992 ) ) ;
#174361=EDGE_LOOP ( 'NONE', ( #50361, #194861, #78872, #120905 ) ) ;
#174393=CARTESIAN_POINT ( 'NONE',  ( 36.91746824999999177, 2.880721459617395097E-14, -10.12499999726881583 ) ) ;
#174413=CARTESIAN_POINT ( 'NONE',  ( 28.81842663310012753, -24.98430004053103559, -10.97651405319417783 ) ) ;
#174427=CARTESIAN_POINT ( 'NONE',  ( 0.000000000000000000, -165.0000000000000000, 12.00000000000000355 ) ) ;
#174477=ADVANCED_FACE ( 'NONE', ( #6519 ), #160217, .F. ) ;
#174536=CARTESIAN_POINT ( 'NONE',  ( 3.766062262543149401E-15, -39.95556452105413570, -5.500000000000000000 ) ) ;
#174538=CARTESIAN_POINT ( 'NONE',  ( 20.13181022538189779, 20.85937581585698553, -49.56857446948049528 ) ) ;
#174564=CARTESIAN_POINT ( 'NONE',  ( 29.86685920354754842, -21.69954338932559068, -3.824999997268813345 ) ) ;
#174576=DIRECTION ( 'NONE',  ( 1.000000000000000000, 0.000000000000000000, 0.000000000000000000 ) ) ;
#174580=CARTESIAN_POINT ( 'NONE',  ( -36.91746825000000598, 2.428612866367529932E-14, -9.124999997268814056 ) ) ;
#174627=CARTESIAN_POINT ( 'NONE',  ( -36.91746825000001309, -11.99521256947794789, -3.024999997268812635 ) ) ;
#174628=CARTESIAN_POINT ( 'NONE',  ( -21.47640361312193491, 19.98428748653489961, -52.19293734151715825 ) ) ;
#174640=SHAPE_DEFINITION_REPRESENTATION ( #16244, #92179 ) ;
#174769=CARTESIAN_POINT ( 'NONE',  ( -2.802625768539475093, -39.09149893265184517, -22.99999999999999289 ) ) ;
#174795=CYLINDRICAL_SURFACE ( 'NONE', #8179, 1.500000000000001332 ) ;
#174807=CARTESIAN_POINT ( 'NONE',  ( 27.81822689058061115, -28.32190533958846856, -20.09416750255128292 ) ) ;
#174824=DIRECTION ( 'NONE',  ( -0.000000000000000000, -0.000000000000000000, 1.000000000000000000 ) ) ;
#174843=CARTESIAN_POINT ( 'NONE',  ( 0.000000000000000000, -78.67194367458512261, -23.00000000000000000 ) ) ;
#174863=( BOUNDED_CURVE ( )  B_SPLINE_CURVE ( 2, ( #4351, #172232, #171243, #143871, #109562, #2380, #5350, #173234, #139887, #19545, #95379 ),
 .UNSPECIFIED., .F., .T. ) 
 B_SPLINE_CURVE_WITH_KNOTS ( ( 3, 2, 2, 2, 2, 3 ),
 ( 0.7000000000000000666, 0.7200000000000000844, 0.7400000000000001021, 0.7600000000000000089, 0.7800000000000000266, 0.8000000000000000444 ),
 .UNSPECIFIED. ) 
 CURVE ( )  GEOMETRIC_REPRESENTATION_ITEM ( )  RATIONAL_B_SPLINE_CURVE ( ( 0.9999999999999997780, 0.9510565162951537532, 1.000000000000000000, 0.9510565162951535312, 1.000000000000000000, 0.9510565162951535312, 1.000000000000000000, 0.9510565162951535312, 1.000000000000000000, 0.9510565162951535312, 1.000000000000000000 ) ) 
 REPRESENTATION_ITEM ( '' )  );
#174879=CARTESIAN_POINT ( 'NONE',  ( -19.41322597532237637, -37.10879518268991006, -19.41738833682087062 ) ) ;
#174880=EDGE_LOOP ( 'NONE', ( #106237, #28820, #57770, #139549 ) ) ;
#174891=CARTESIAN_POINT ( 'NONE',  ( 9.561620553927779653, 11.67072985713511102, -62.04564570087489983 ) ) ;
#174895=CYLINDRICAL_SURFACE ( 'NONE', #72872, 16.70000000000002061 ) ;
#174903=CARTESIAN_POINT ( 'NONE',  ( 30.74264578624800137, -22.33583958711395212, -8.949999994537627401 ) ) ;
#174904=B_SPLINE_CURVE_WITH_KNOTS ( 'NONE', 3,
 ( #1217, #27638, #152920, #91229, #74124, #93230, #183284, #169079, #46752, #89279, #150969, #29598, #124575, #184271, #42791, #135795, #60908, #30585, #136764, #120601, #45754, #154915 ),
 .UNSPECIFIED., .F., .F.,
 ( 4, 2, 2, 2, 2, 2, 2, 2, 2, 2, 4 ),
 ( 1.967889508672852735E-07, 0.0003311341139581320116, 0.0006620714389653966627, 0.0009930087639726614766, 0.001323946088979925748, 0.002647695389008988473, 0.003309570039023513113, 0.003971444689038037754, 0.004633319339052562394, 0.004964256664059822979, 0.005295193989067083565 ),
 .UNSPECIFIED. ) ;
#174924=EDGE_CURVE ( 'NONE', #166806, #63287, #31445, .T. ) ;
#174937=CARTESIAN_POINT ( 'NONE',  ( -2.662494480112493012, -37.13692398601925504, -32.59999999999999432 ) ) ;
#175010=CARTESIAN_POINT ( 'NONE',  ( -16.47688973148989788, -17.58748242838617060, -56.92523117286675927 ) ) ;
#175049=ORIENTED_EDGE ( 'NONE', *, *, #24639, .F. ) ;
#175073=CARTESIAN_POINT ( 'NONE',  ( -16.37811251030163717, 0.9487569900775056908, -59.27680374464310376 ) ) ;
#175105=CARTESIAN_POINT ( 'NONE',  ( 36.30973463497186060, -18.33876584756081130, -18.81039752657306252 ) ) ;
#175123=ADVANCED_FACE ( 'NONE', ( #113662 ), #81324, .F. ) ;
#175219=CARTESIAN_POINT ( 'NONE',  ( 9.304348965730421028, 11.16651649332241192, -60.11051939825534873 ) ) ;
#175249=DIRECTION ( 'NONE',  ( 0.000000000000000000, 0.000000000000000000, 1.000000000000000000 ) ) ;
#175257=ORIENTED_EDGE ( 'NONE', *, *, #188177, .T. ) ;
#175262=ORIENTED_EDGE ( 'NONE', *, *, #21485, .F. ) ;
#175272=CARTESIAN_POINT ( 'NONE',  ( -26.39110954545251886, -27.12960848547384884, -16.54511501588637046 ) ) ;
#175295=CARTESIAN_POINT ( 'NONE',  ( -31.90000000000002700, 0.1356448107286085669, -45.64921306006598201 ) ) ;
#175298=CARTESIAN_POINT ( 'NONE',  ( 6.434671708797586653, 6.434671708797580436, -63.95112321872120731 ) ) ;
#175299=DIRECTION ( 'NONE',  ( 1.000000000000000000, 0.000000000000000000, 0.000000000000000000 ) ) ;
#175317=UNCERTAINTY_MEASURE_WITH_UNIT (LENGTH_MEASURE( 1.000000000000000082E-05 ), #66915, 'distance_accuracy_value', 'NONE');
#175321=CARTESIAN_POINT ( 'NONE',  ( -11.40812507854754720, -35.11059874428192273, -4.224999997268813701 ) ) ;
#175331=CARTESIAN_POINT ( 'NONE',  ( 34.17105881114488852, -20.77207671795054011, -21.54825371331146044 ) ) ;
#175349=ORIENTED_EDGE ( 'NONE', *, *, #48406, .F. ) ;
#175380=CARTESIAN_POINT ( 'NONE',  ( 36.91746824999999887, 11.99521256947799053, -1.524999997268813745 ) ) ;
#175384=FACE_OUTER_BOUND ( 'NONE', #35617, .T. ) ;
#175399=EDGE_CURVE ( 'NONE', #119464, #84310, #183509, .T. ) ;
#175415=FACE_OUTER_BOUND ( 'NONE', #158092, .T. ) ;
#175417=CARTESIAN_POINT ( 'NONE',  ( 29.77433414031399650, -1.366177905283701532, -51.67655205196556523 ) ) ;
#175423=AXIS2_PLACEMENT_3D ( 'NONE', #71238, #73248, #25752 ) ;
#175537=DIRECTION ( 'NONE',  ( 0.000000000000000000, 0.000000000000000000, 1.000000000000000000 ) ) ;
#175542=CARTESIAN_POINT ( 'NONE',  ( -24.54195369798066295, -31.38977029645269212, -21.36864394644175746 ) ) ;
#175546=SPHERICAL_SURFACE ( 'NONE', #141182, 40.00000000000002132 ) ;
#175552=DIRECTION ( 'NONE',  ( -0.000000000000000000, -0.000000000000000000, 1.000000000000000000 ) ) ;
#175554=CARTESIAN_POINT ( 'NONE',  ( -11.40812507854755609, 35.11059874428196537, -5.024999997268813523 ) ) ;
#175583=B_SPLINE_CURVE_WITH_KNOTS ( 'NONE', 3,
 ( #108485, #152996, #45830, #16487, #184348, #167202, #28700, #15497, #89355, #13507 ),
 .UNSPECIFIED., .F., .F.,
 ( 4, 2, 2, 2, 4 ),
 ( 0.002442800151708459776, 0.003053169662661163030, 0.003663539173613866284, 0.004273908684566569971, 0.004884278195519273225 ),
 .UNSPECIFIED. ) ;
#175629=CARTESIAN_POINT ( 'NONE',  ( 15.34147874640870590, 17.41603567004569797, -57.57865799245707450 ) ) ;
#175640=EDGE_LOOP ( 'NONE', ( #99398, #162382, #153702, #54726 ) ) ;
#175652=AXIS2_PLACEMENT_3D ( 'NONE', #135596, #105241, #27431 ) ;
#175759=AXIS2_PLACEMENT_3D ( 'NONE', #138118, #139104, #153280 ) ;
#175764=CARTESIAN_POINT ( 'NONE',  ( -6.310639553376649502, -38.36010752037731208, -23.94295717419116443 ) ) ;
#175771=CARTESIAN_POINT ( 'NONE',  ( -0.4033639900674926282, -16.64831001466045279, -61.36868776158050309 ) ) ;
#175788=CARTESIAN_POINT ( 'NONE',  ( 2.500000000000000000, -105.0000000000000000, 7.000000000000003553 ) ) ;
#175803=ORIENTED_EDGE ( 'NONE', *, *, #46060, .T. ) ;
#175806=CYLINDRICAL_SURFACE ( 'NONE', #182735, 1.499999999999997780 ) ;
#175808=LINE ( 'NONE', #6932, #191645 ) ;
#175822=CARTESIAN_POINT ( 'NONE',  ( -0.1282610754043937429, -31.90000000000003411, -49.13275782002543934 ) ) ;
#175852=AXIS2_PLACEMENT_3D ( 'NONE', #145557, #7035, #43386 ) ;
#175867=CARTESIAN_POINT ( 'NONE',  ( 4.647474457565486646E-15, -28.90000000000004476, -49.67367017693150189 ) ) ;
#175879=CARTESIAN_POINT ( 'NONE',  ( -9.816778487192582503, -45.49549017958077712, -23.86159105743509556 ) ) ;
#175941=CARTESIAN_POINT ( 'NONE',  ( -26.46959431505283789, -27.26463967846487435, -10.00000000000000000 ) ) ;
#175951=DIRECTION ( 'NONE',  ( 0.000000000000000000, 0.000000000000000000, 1.000000000000000000 ) ) ;
#176016=CARTESIAN_POINT ( 'NONE',  ( -14.93859650326285227, -17.05398664991142255, -57.95493304017681169 ) ) ;
#176035=VERTEX_POINT ( 'NONE', #78864 ) ;
#176059=MECHANICAL_DESIGN_GEOMETRIC_PRESENTATION_REPRESENTATION('',(#124365),#166258);
#176074=CARTESIAN_POINT ( 'NONE',  ( 37.99999999999998579, -12.34694845685043951, -4.849999994537626868 ) ) ;
#176088=ORIENTED_EDGE ( 'NONE', *, *, #168309, .F. ) ;
#176100=EDGE_LOOP ( 'NONE', ( #177044, #2292, #6416, #108147 ) ) ;
#176109=( NAMED_UNIT ( * ) SI_UNIT ( $, .STERADIAN. ) SOLID_ANGLE_UNIT ( ) );
#176113=CARTESIAN_POINT ( 'NONE',  ( 31.73299246115101724, -20.69072564976797324, -20.42656251077089991 ) ) ;
#176171=CIRCLE ( 'NONE', #89013, 13.70000000000001528 ) ;
#176177=CARTESIAN_POINT ( 'NONE',  ( -3.573655867282028392E-15, 2.428612866367529932E-14, -25.00000000000000000 ) ) ;
#176217=DIRECTION ( 'NONE',  ( -1.000000000000000000, 0.000000000000000000, 0.000000000000000000 ) ) ;
#176257=CARTESIAN_POINT ( 'NONE',  ( 0.000000000000000000, -165.0000000000000000, 12.00000000000000355 ) ) ;
#176274=CIRCLE ( 'NONE', #21240, 24.30000000000003268 ) ;
#176292=DIRECTION ( 'NONE',  ( -1.000000000000000000, 0.000000000000000000, 0.000000000000000000 ) ) ;
#176295=ORIENTED_EDGE ( 'NONE', *, *, #76288, .T. ) ;
#176297=DIRECTION ( 'NONE',  ( -1.000000000000000000, 0.000000000000000000, -4.336808689942016750E-16 ) ) ;
#176302=CARTESIAN_POINT ( 'NONE',  ( -31.20457203169703675, 1.278449583442399451, -46.64972497815392671 ) ) ;
#176306=DIRECTION ( 'NONE',  ( 0.000000000000000000, 0.000000000000000000, 1.000000000000000000 ) ) ;
#176309=EDGE_CURVE ( 'NONE', #71928, #84310, #109090, .T. ) ;
#176327=ORIENTED_EDGE ( 'NONE', *, *, #83071, .F. ) ;
#176330=CARTESIAN_POINT ( 'NONE',  ( 29.86685920354754487, 21.69954338932564752, -7.424999997268813878 ) ) ;
#176348=DIRECTION ( 'NONE',  ( -0.000000000000000000, 0.000000000000000000, -1.000000000000000000 ) ) ;
#176392=CARTESIAN_POINT ( 'NONE',  ( 22.81625015709510151, -31.40387420917324590, -1.924999997268813434 ) ) ;
#176413=AXIS2_PLACEMENT_3D ( 'NONE', #29620, #76105, #185284 ) ;
#176427=FACE_OUTER_BOUND ( 'NONE', #28465, .T. ) ;
#176428=CARTESIAN_POINT ( 'NONE',  ( -38.00000000000000711, 2.428612866367529932E-14, -2.000000000000000000 ) ) ;
#176431=CARTESIAN_POINT ( 'NONE',  ( 0.000000000000000000, 0.000000000000000000, -54.21489346206828230 ) ) ;
#176565=DIRECTION ( 'NONE',  ( -0.000000000000000000, -0.000000000000000000, 1.000000000000000000 ) ) ;
#176675=CARTESIAN_POINT ( 'NONE',  ( -11.30153831258470731, -190.0000000000000000, -15.00000000000000178 ) ) ;
#176701=ORIENTED_EDGE ( 'NONE', *, *, #28409, .F. ) ;
#176720=CARTESIAN_POINT ( 'NONE',  ( -11.57021340674615928, -12.01197775448600247, -59.14478828020191514 ) ) ;
#176775=CYLINDRICAL_SURFACE ( 'NONE', #187332, 1.499999999999997780 ) ;
#176797=CARTESIAN_POINT ( 'NONE',  ( -31.42649584489976178, 1.097581692000625386, -49.72218688481379445 ) ) ;
#176812=DIRECTION ( 'NONE',  ( 1.000000000000000000, 0.000000000000000000, 0.000000000000000000 ) ) ;
#176814=CARTESIAN_POINT ( 'NONE',  ( -8.673617379884035472E-16, 7.600000000000007638, -65.00100000000003320 ) ) ;
#176816=CARTESIAN_POINT ( 'NONE',  ( 23.48529157249599919, 32.32473071737754111, -8.449999994537625625 ) ) ;
#176823=CARTESIAN_POINT ( 'NONE',  ( 4.313351365237961588, -4.313351365237934054, -62.50719930893269805 ) ) ;
#176825=CARTESIAN_POINT ( 'NONE',  ( 22.71027669145893668, -22.38345232661798079, -45.66972496404596882 ) ) ;
#176829=CARTESIAN_POINT ( 'NONE',  ( 0.000000000000000000, 0.000000000000000000, -18.00000000000000000 ) ) ;
#176834=CARTESIAN_POINT ( 'NONE',  ( 27.03637221620040876, -26.30952996081074957, -20.42959548696013528 ) ) ;
#176850=CIRCLE ( 'NONE', #54160, 28.90000000000004476 ) ;
#176868=CARTESIAN_POINT ( 'NONE',  ( -0.2180554607492796448, -24.28797299941338395, -56.78142080721293894 ) ) ;
#176888=CARTESIAN_POINT ( 'NONE',  ( -16.14548778791224137, -40.33029071462993187, -21.07572238977526169 ) ) ;
#176889=VERTEX_POINT ( 'NONE', #24197 ) ;
#176900=CARTESIAN_POINT ( 'NONE',  ( 9.295088167215988406, 11.16688150046370964, -62.26853652665833749 ) ) ;
#176945=VECTOR ( 'NONE', #147537, 1000.000000000000000 ) ;
#176962=DIRECTION ( 'NONE',  ( -0.000000000000000000, -0.000000000000000000, 1.000000000000000000 ) ) ;
#177024=CARTESIAN_POINT ( 'NONE',  ( -16.63275618507867293, -17.54166085810596343, -56.86956483720373257 ) ) ;
#177044=ORIENTED_EDGE ( 'NONE', *, *, #28742, .T. ) ;
#177047=CARTESIAN_POINT ( 'NONE',  ( 19.23457310888372973, -35.06695140040304182, -26.03237767043686546 ) ) ;
#177090=CARTESIAN_POINT ( 'NONE',  ( -15.38830714838546854, 1.491100297016104470, -59.71292413584863823 ) ) ;
#177121=CARTESIAN_POINT ( 'NONE',  ( 30.74264578624799782, 22.33583958711400541, -10.54999999453762705 ) ) ;
#177124=CARTESIAN_POINT ( 'NONE',  ( 26.39110954545158805, -27.12960848547524151, -16.54511501588457634 ) ) ;
#177186=CARTESIAN_POINT ( 'NONE',  ( -5.000000000000003553, -4.999999999999996447, -15.00000000000000000 ) ) ;
#177226=CARTESIAN_POINT ( 'NONE',  ( 11.74264578624800315, -36.14014761921581709, -3.149999994537626247 ) ) ;
#177278=VERTEX_POINT ( 'NONE', #26200 ) ;
#177280=VERTEX_POINT ( 'NONE', #85847 ) ;
#177305=ORIENTED_EDGE ( 'NONE', *, *, #115703, .F. ) ;
#177328=CARTESIAN_POINT ( 'NONE',  ( -4.313351365237979351, -4.313351365237916291, -64.53213882399992940 ) ) ;
#177337=CARTESIAN_POINT ( 'NONE',  ( -36.91746825000001309, -11.99521256947794789, -8.524999997268812635 ) ) ;
#177342=DIRECTION ( 'NONE',  ( 1.000000000000000000, 0.000000000000000000, 0.000000000000000000 ) ) ;
#177346=CARTESIAN_POINT ( 'NONE',  ( 33.52048507002423605, -21.84028095222489796, -24.62089730557384826 ) ) ;
#177397=CARTESIAN_POINT ( 'NONE',  ( 36.91746824999999177, 2.880721459617395097E-14, -9.624999997268814056 ) ) ;
#177432=LINE ( 'NONE', #89390, #111231 ) ;
#177434=EDGE_CURVE ( 'NONE', #12418, #100015, #50929, .T. ) ;
#177460=EDGE_CURVE ( 'NONE', #93735, #40506, #38086, .T. ) ;
#177464=VERTEX_POINT ( 'NONE', #72696 ) ;
#177498=CIRCLE ( 'NONE', #141943, 59.99999999999998579 ) ;
#177522=CIRCLE ( 'NONE', #190338, 69.99999999999998579 ) ;
#177545=CARTESIAN_POINT ( 'NONE',  ( 19.98452092126598245, 21.51070015259071155, -49.12424573582180898 ) ) ;
#177568=CARTESIAN_POINT ( 'NONE',  ( -1.304248841091933035E-15, -21.30000000000002913, -56.46919128290398504 ) ) ;
#177570=CARTESIAN_POINT ( 'NONE',  ( -36.91746825000000598, -11.99521256947794789, -2.524999997268813523 ) ) ;
#177633=CIRCLE ( 'NONE', #61417, 40.00000000000000000 ) ;
#177642=CARTESIAN_POINT ( 'NONE',  ( 14.63400850047069213, 16.39429727647822688, -58.42335914450117684 ) ) ;
#177665=EDGE_CURVE ( 'NONE', #111207, #58211, #69686, .T. ) ;
#177771=FACE_OUTER_BOUND ( 'NONE', #55997, .T. ) ;
#177800=VECTOR ( 'NONE', #159252, 1000.000000000000000 ) ;
#177813=CARTESIAN_POINT ( 'NONE',  ( -11.74264578624800670, 36.14014761921585972, -8.149999994537626691 ) ) ;
#177822=CARTESIAN_POINT ( 'NONE',  ( 69.65682714487590488, -71.74905178543389184, -23.00000000000000000 ) ) ;
#177826=CARTESIAN_POINT ( 'NONE',  ( -24.30000000000003268, 2.668083032619853614E-13, -64.92279855667830191 ) ) ;
#177831=ORIENTED_EDGE ( 'NONE', *, *, #74445, .F. ) ;
#177864=CARTESIAN_POINT ( 'NONE',  ( -36.91746825000000598, -11.99521256947794789, -3.024999997268813079 ) ) ;
#177869=ORIENTED_EDGE ( 'NONE', *, *, #79473, .T. ) ;
#177875=CARTESIAN_POINT ( 'NONE',  ( 0.000000000000000000, 0.000000000000000000, -59.13370768023891344 ) ) ;
#177887=CARTESIAN_POINT ( 'NONE',  ( -9.128739734652899784, -39.45218800495356248, -25.46847458086992333 ) ) ;
#177888=ORIENTED_EDGE ( 'NONE', *, *, #135199, .F. ) ;
#177903=CARTESIAN_POINT ( 'NONE',  ( 23.94081952771230704, -0.9791052130474939830, -54.49391133501600137 ) ) ;
#178013=CARTESIAN_POINT ( 'NONE',  ( -15.23577778804332539, -17.33993248393032616, -57.66841858811282862 ) ) ;
#178016=CARTESIAN_POINT ( 'NONE',  ( -23.31485601308163780, -29.82028178163005450, -21.55021174911970050 ) ) ;
#178029=ORIENTED_EDGE ( 'NONE', *, *, #144097, .T. ) ;
#178036=CARTESIAN_POINT ( 'NONE',  ( 4.521720347981165844, -38.96825017273093295, -33.00000000000000711 ) ) ;
#178058=DIRECTION ( 'NONE',  ( 1.000000000000000000, 0.000000000000000000, 0.000000000000000000 ) ) ;
#178062=CARTESIAN_POINT ( 'NONE',  ( 22.36433501015068259, 22.72511982729788471, -49.15411784021381436 ) ) ;
#178101=B_SPLINE_CURVE_WITH_KNOTS ( 'NONE', 3,
 ( #63055, #48896, #156063, #124735, #128693, #51865, #113525, #96367, #79221, #175219, #140891, #157065, #3371, #36684, #64059, #125729, #97348, #18561, #187428, #126702, #188406, #49884, #111549, #23537 ),
 .UNSPECIFIED., .F., .F.,
 ( 4, 2, 2, 2, 2, 2, 2, 2, 2, 2, 2, 4 ),
 ( 2.787091051215036154E-07, 0.0003070612385125908827, 0.0006138437679200602071, 0.001227408826735002434, 0.001534191356142473005, 0.001840973885549943576, 0.002147756414957414147, 0.002454538944364884935, 0.003068104003179817837, 0.003681669061994749872, 0.004295234120809682775, 0.004908799179624614810 ),
 .UNSPECIFIED. ) ;
#178142=DIRECTION ( 'NONE',  ( -0.000000000000000000, -0.000000000000000000, 1.000000000000000000 ) ) ;
#178145=CARTESIAN_POINT ( 'NONE',  ( 4.999999999999996447, 5.000000000000003553, -15.00000000000000000 ) ) ;
#178146=VERTEX_POINT ( 'NONE', #145992 ) ;
#178184=CARTESIAN_POINT ( 'NONE',  ( 0.3963287095611701671, 6.139799388069159036, -64.52448944440712353 ) ) ;
#178238=ADVANCED_FACE ( 'NONE', ( #6474, #116665, #178356 ), #143998, .F. ) ;
#178269=ORIENTED_EDGE ( 'NONE', *, *, #52114, .T. ) ;
#178273=EDGE_LOOP ( 'NONE', ( #182493, #114692, #15803, #7263 ) ) ;
#178283=CARTESIAN_POINT ( 'NONE',  ( 0.8806672422397930911, 29.18146119162907581, -52.34378264204461573 ) ) ;
#178300=CARTESIAN_POINT ( 'NONE',  ( -193.3062444957834884, -155.7167183371838064, -25.00000000000000000 ) ) ;
#178310=CARTESIAN_POINT ( 'NONE',  ( 0.000000000000000000, 0.000000000000000000, -62.50719930893269805 ) ) ;
#178316=ORIENTED_EDGE ( 'NONE', *, *, #121295, .T. ) ;
#178331=CARTESIAN_POINT ( 'NONE',  ( -30.74264578624800492, -22.33583958711396278, -1.800000000000000044 ) ) ;
#178340=CARTESIAN_POINT ( 'NONE',  ( 17.18269478283316332, -17.18269478283309226, -54.21489346206828230 ) ) ;
#178348=CARTESIAN_POINT ( 'NONE',  ( 4.313351365237961588, -4.313351365237934942, -64.92279855667830191 ) ) ;
#178356=FACE_OUTER_BOUND ( 'NONE', #38121, .T. ) ;
#178389=CARTESIAN_POINT ( 'NONE',  ( 22.81625015709509441, 31.40387420917330275, -7.324999997268812457 ) ) ;
#178423=CARTESIAN_POINT ( 'NONE',  ( 37.99999999999999289, 2.893978650043524126E-14, -6.749999994537627224 ) ) ;
#178426=LINE ( 'NONE', #117741, #24079 ) ;
#178429=CARTESIAN_POINT ( 'NONE',  ( 10.59477242850415024, -90.60836494048558620, -15.00000000000000178 ) ) ;
#178436=CARTESIAN_POINT ( 'NONE',  ( 0.000000000000000000, 0.000000000000000000, -10.00000000000000000 ) ) ;
#178537=CARTESIAN_POINT ( 'NONE',  ( 20.34442274205741796, 22.47021661561673156, -47.91864530057671345 ) ) ;
#178551=CARTESIAN_POINT ( 'NONE',  ( -27.00987238947304547, -29.10436634937588707, -20.14159902729970852 ) ) ;
#178558=ORIENTED_EDGE ( 'NONE', *, *, #174924, .T. ) ;
#178562=CARTESIAN_POINT ( 'NONE',  ( 36.91746824999999177, 11.99521256947799230, -3.524999997268813079 ) ) ;
#178570=ORIENTED_EDGE ( 'NONE', *, *, #195656, .T. ) ;
#178572=CARTESIAN_POINT ( 'NONE',  ( -37.66961640367473052, -4.999999999999976019, -18.00000000000000355 ) ) ;
#178574=CARTESIAN_POINT ( 'NONE',  ( 28.66576453816018244, -27.89900116845191391, -15.73147987472289167 ) ) ;
#178590=AXIS2_PLACEMENT_3D ( 'NONE', #199001, #91787, #62451 ) ;
#178599=ORIENTED_EDGE ( 'NONE', *, *, #119036, .T. ) ;
#178686=EDGE_CURVE ( 'NONE', #126933, #23953, #199452, .T. ) ;
#178697=VERTEX_POINT ( 'NONE', #12506 ) ;
#178752=CARTESIAN_POINT ( 'NONE',  ( -17.34149035984848553, 17.02389920581777005, -54.21489346206831073 ) ) ;
#178759=AXIS2_PLACEMENT_3D ( 'NONE', #173185, #19497, #81142 ) ;
#178809=CARTESIAN_POINT ( 'NONE',  ( 1.227931366032057224E-14, 24.30000000000003268, -54.21489346206828230 ) ) ;
#178813=CARTESIAN_POINT ( 'NONE',  ( -23.48529157249599919, -32.32473071737750558, -7.449999994537624737 ) ) ;
#178820=DIRECTION ( 'NONE',  ( 0.000000000000000000, 0.000000000000000000, -1.000000000000000000 ) ) ;
#178829=CARTESIAN_POINT ( 'NONE',  ( -14.62203461105344005, -16.12203461105316649, -64.92279855667830191 ) ) ;
#178831=CARTESIAN_POINT ( 'NONE',  ( -1.399641368455697865, -29.85394078251579941, -51.58569050288881641 ) ) ;
#178866=CARTESIAN_POINT ( 'NONE',  ( 22.81625015709509441, 31.40387420917330275, -3.824999997268813345 ) ) ;
#178867=DIRECTION ( 'NONE',  ( 0.000000000000000000, 0.000000000000000000, -1.000000000000000000 ) ) ;
#178876=CARTESIAN_POINT ( 'NONE',  ( 2.662494480112515660, -37.13692398601924793, -32.59999999999999432 ) ) ;
#178882=CARTESIAN_POINT ( 'NONE',  ( 11.30153831258470731, -180.0000000000000000, 0.000000000000000000 ) ) ;
#178888=CARTESIAN_POINT ( 'NONE',  ( -20.47811964340476365, -34.28713832285652785, -21.14919058558906784 ) ) ;
#178900=ORIENTED_EDGE ( 'NONE', *, *, #47633, .F. ) ;
#178904=DIRECTION ( 'NONE',  ( 1.000000000000000000, 0.000000000000000000, 0.000000000000000000 ) ) ;
#178917=CARTESIAN_POINT ( 'NONE',  ( 1.491112435928470425, 15.38843874529032618, -61.89150209872707364 ) ) ;
#179020=CARTESIAN_POINT ( 'NONE',  ( -6.020228577223754586E-15, 39.95556452105416412, -6.500000000000000000 ) ) ;
#179023=CARTESIAN_POINT ( 'NONE',  ( -28.61453998622349104, -24.72048905145116038, -21.14736193440031897 ) ) ;
#179029=VECTOR ( 'NONE', #176306, 1000.000000000000000 ) ;
#179045=FACE_OUTER_BOUND ( 'NONE', #94515, .T. ) ;
#179076=CARTESIAN_POINT ( 'NONE',  ( -9.669289179520820454, -11.80006683339779805, -59.80355761763873801 ) ) ;
#179085=CYLINDRICAL_SURFACE ( 'NONE', #56719, 59.99999999999998579 ) ;
#179090=CARTESIAN_POINT ( 'NONE',  ( 8.388830574159379737E-16, 13.70000000000001528, -65.00100000000003320 ) ) ;
#179188=ORIENTED_EDGE ( 'NONE', *, *, #182692, .T. ) ;
#179194=DIRECTION ( 'NONE',  ( -0.000000000000000000, -0.000000000000000000, -1.000000000000000000 ) ) ;
#179291=EDGE_CURVE ( 'NONE', #138197, #85313, #132834, .T. ) ;
#179317=CARTESIAN_POINT ( 'NONE',  ( 193.3062444957835453, -155.7167183371837496, -15.00000000000000178 ) ) ;
#179323=DIRECTION ( 'NONE',  ( 0.000000000000000000, 0.000000000000000000, 1.000000000000000000 ) ) ;
#179342=CARTESIAN_POINT ( 'NONE',  ( 29.86685920354754487, 21.69954338932564752, -9.424999997268814766 ) ) ;
#179351=CARTESIAN_POINT ( 'NONE',  ( 30.36026264928092999, -25.76863830327009453, -21.12575414591866974 ) ) ;
#179352=CARTESIAN_POINT ( 'NONE',  ( 2.500000000000000000, 0.000000000000000000, -62.91767397929362460 ) ) ;
#179364=VERTEX_POINT ( 'NONE', #164187 ) ;
#179372=VERTEX_POINT ( 'NONE', #71170 ) ;
#179396=EDGE_LOOP ( 'NONE', ( #58510, #79131 ) ) ;
#179400=CARTESIAN_POINT ( 'NONE',  ( -22.81625015709510507, 31.40387420917330275, -8.924999997268814766 ) ) ;
#179456=ADVANCED_FACE ( 'NONE', ( #151990 ), #19573, .T. ) ;
#179471=VERTEX_POINT ( 'NONE', #99246 ) ;
#179484=AXIS2_PLACEMENT_3D ( 'NONE', #121743, #58110, #59082 ) ;
#179524=ORIENTED_EDGE ( 'NONE', *, *, #125471, .F. ) ;
#179533=EDGE_CURVE ( 'NONE', #22834, #198657, #102625, .T. ) ;
#179550=CARTESIAN_POINT ( 'NONE',  ( -4.158454644149600199, -48.51789971941261825, -23.00000000000039435 ) ) ;
#179575=CARTESIAN_POINT ( 'NONE',  ( -33.78191506369886810, -21.41920200728862511, -24.99999999999999289 ) ) ;
#179646=DIRECTION ( 'NONE',  ( -9.445700745138859830E-17, 1.000000000000000000, 0.000000000000000000 ) ) ;
#179717=AXIS2_PLACEMENT_3D ( 'NONE', #165039, #181214, #11365 ) ;
#179725=CARTESIAN_POINT ( 'NONE',  ( -3.573655867282028392E-15, 2.428612866367529932E-14, -25.00000000000000000 ) ) ;
#179762=AXIS2_PLACEMENT_3D ( 'NONE', #3999, #97979, #144505 ) ;
#179785=CARTESIAN_POINT ( 'NONE',  ( 12.14253177836985564, -10.17673712963189381, -61.72896360825912865 ) ) ;
#179802=CARTESIAN_POINT ( 'NONE',  ( -5.000000000000003553, 37.66961640367474473, -25.00000000000000000 ) ) ;
#179823=CARTESIAN_POINT ( 'NONE',  ( 23.48529157249600630, -32.32473071737749137, -7.049999994537626158 ) ) ;
#179829=CARTESIAN_POINT ( 'NONE',  ( 6.703997108180972830, -4.665206786362193547, -62.11218654135820572 ) ) ;
#179835=CARTESIAN_POINT ( 'NONE',  ( -10.58667710475869939, 9.243954752495751492, -60.30599866924266905 ) ) ;
#179874=CARTESIAN_POINT ( 'NONE',  ( -36.91746825000000598, 2.428612866367529932E-14, -7.124999997268813168 ) ) ;
#179875=CARTESIAN_POINT ( 'NONE',  ( -1.340157125434632501, -22.10131684062752555, -58.31342218742629768 ) ) ;
#179898=CARTESIAN_POINT ( 'NONE',  ( -29.51469970000582066, -26.64072072720978923, -20.60124869738260855 ) ) ;
#179925=DIRECTION ( 'NONE',  ( -0.07151044867601408228, 0.9974398506828143773, 0.000000000000000000 ) ) ;
#179963=B_SPLINE_CURVE_WITH_KNOTS ( 'NONE', 3,
 ( #180878, #42353, #76644, #75648, #183839, #198016, #134365, #45328, #87834, #106978, #74674, #120169 ),
 .UNSPECIFIED., .F., .F.,
 ( 4, 2, 2, 2, 2, 4 ),
 ( 0.000000000000000000, 0.002596730589505801597, 0.003895095884258703480, 0.005193461179011606664, 0.007790191768517405226, 0.01038692235802320812 ),
 .UNSPECIFIED. ) ;
#180033=CARTESIAN_POINT ( 'NONE',  ( -31.73029476377070424, -20.92000799991019022, -24.48145274275711003 ) ) ;
#180055=FACE_OUTER_BOUND ( 'NONE', #53273, .T. ) ;
#180063=CIRCLE ( 'NONE', #138014, 28.90000000000004476 ) ;
#180080=CARTESIAN_POINT ( 'NONE',  ( 22.04895058596758517, 22.89469264416797856, -49.28358967601002405 ) ) ;
#180085=CARTESIAN_POINT ( 'NONE',  ( -23.48529157249600985, 32.32473071737754111, -4.299999999999999822 ) ) ;
#180102=CARTESIAN_POINT ( 'NONE',  ( 6.613545406318523945, -46.94410406412048786, -22.68594355512400895 ) ) ;
#180120=ORIENTED_EDGE ( 'NONE', *, *, #103099, .F. ) ;
#180288=LINE ( 'NONE', #54913, #46953 ) ;
#180322=CARTESIAN_POINT ( 'NONE',  ( 17.62203461105333702, -16.12203461105326951, -57.08650645001478097 ) ) ;
#180329=DIRECTION ( 'NONE',  ( 0.000000000000000000, 0.000000000000000000, 1.000000000000000000 ) ) ;
#180343=CARTESIAN_POINT ( 'NONE',  ( -36.91746825000001309, -11.99521256947794789, -10.52499999726881441 ) ) ;
#180348=CARTESIAN_POINT ( 'NONE',  ( 0.000000000000000000, 0.000000000000000000, 0.000000000000000000 ) ) ;
#180370=CARTESIAN_POINT ( 'NONE',  ( 4.562484170618506418, -48.30423733473406145, -23.00000000000000355 ) ) ;
#180374=ORIENTED_EDGE ( 'NONE', *, *, #67646, .T. ) ;
#180402=CARTESIAN_POINT ( 'NONE',  ( -36.91746825000001309, 11.99521256947798342, -4.724999997268811924 ) ) ;
#180406=DIRECTION ( 'NONE',  ( 0.000000000000000000, 0.000000000000000000, 1.000000000000000000 ) ) ;
#180450=DIRECTION ( 'NONE',  ( 1.000000000000000000, 0.000000000000000000, 0.000000000000000000 ) ) ;
#180474=( BOUNDED_CURVE ( )  B_SPLINE_CURVE ( 2, ( #67916, #191266, #51750, #70928, #190274, #84072, #69927, #129569, #177121, #130580, #131592 ),
 .UNSPECIFIED., .F., .F. ) 
 B_SPLINE_CURVE_WITH_KNOTS ( ( 3, 2, 2, 2, 2, 3 ),
 ( 0.8000000000000000444, 0.8199999999999999512, 0.8399999999999999689, 0.8599999999999999867, 0.8800000000000000044, 0.9000000000000000222 ),
 .UNSPECIFIED. ) 
 CURVE ( )  GEOMETRIC_REPRESENTATION_ITEM ( )  RATIONAL_B_SPLINE_CURVE ( ( 1.000000000000000000, 0.9510565162951535312, 1.000000000000000000, 0.9510565162951535312, 1.000000000000000000, 0.9510565162951535312, 1.000000000000000000, 0.9510565162951535312, 1.000000000000000000, 0.9510565162951535312, 1.000000000000000000 ) ) 
 REPRESENTATION_ITEM ( '' )  );
#180576=CARTESIAN_POINT ( 'NONE',  ( 22.81625015709510151, -31.40387420917324590, -9.924999997268814766 ) ) ;
#180612=ORIENTED_EDGE ( 'NONE', *, *, #23142, .T. ) ;
#180672=ADVANCED_FACE ( 'NONE', ( #134517 ), #196203, .F. ) ;
#180711=SURFACE_SIDE_STYLE ('',( #133174 ) ) ;
#180767=ADVANCED_FACE ( 'NONE', ( #12178 ), #28345, .F. ) ;
#180781=CARTESIAN_POINT ( 'NONE',  ( -36.91746825000000598, 2.428612866367529932E-14, -10.62499999726881406 ) ) ;
#180782=CARTESIAN_POINT ( 'NONE',  ( 26.46959431505284499, -27.26463967846488146, -10.00000000000000000 ) ) ;
#180816=CARTESIAN_POINT ( 'NONE',  ( -6.020228577223754586E-15, 39.95556452105416412, -8.249999994537628112 ) ) ;
#180822=VECTOR ( 'NONE', #55191, 1000.000000000000000 ) ;
#180823=CARTESIAN_POINT ( 'NONE',  ( 5.381136069153227730, -3.845012989623188382, -62.42122758075691280 ) ) ;
#180841=CARTESIAN_POINT ( 'NONE',  ( -23.66491666289338980, 1.240847218223332327, -57.22545927231451657 ) ) ;
#180868=CARTESIAN_POINT ( 'NONE',  ( -29.86685920354755552, 21.69954338932564397, -3.324999997268813345 ) ) ;
#180876=PRODUCT_DEFINITION ( 'UNKNOWN', '', #108208, #94919 ) ;
#180878=CARTESIAN_POINT ( 'NONE',  ( 28.47622644277404191, -25.16156846422445881, -16.68312038616162241 ) ) ;
#180890=CARTESIAN_POINT ( 'NONE',  ( -28.61471831746303707, -27.54183658529284529, -20.22090314798039401 ) ) ;
#180904=CARTESIAN_POINT ( 'NONE',  ( 21.39623730026196924, -0.5392447798056823061, -56.39940532337662660 ) ) ;
#180916=DIRECTION ( 'NONE',  ( -0.000000000000000000, -0.000000000000000000, 1.000000000000000000 ) ) ;
#180925=LINE ( 'NONE', #12078, #156513 ) ;
#180954=CARTESIAN_POINT ( 'NONE',  ( -21.30000000000002913, 2.244099063931684814E-13, -58.85720012050612837 ) ) ;
#180996=B_SPLINE_CURVE_WITH_KNOTS ( 'NONE', 3,
 ( #119338, #55655, #85989, #40491, #197180, #26342, #104162, #149670, #118340, #148678, #87982, #181024 ),
 .UNSPECIFIED., .F., .F.,
 ( 4, 2, 2, 2, 2, 4 ),
 ( 1.969502665979568066E-07, 0.0004083572201530094635, 0.0008165174900394210449, 0.001632838029812235317, 0.002449158569585050023, 0.003265479109357864295 ),
 .UNSPECIFIED. ) ;
#181024=CARTESIAN_POINT ( 'NONE',  ( 1.500000000000003553, 30.40000000000004476, -47.75060438757614634 ) ) ;
#181058=EDGE_LOOP ( 'NONE', ( #57163, #53193, #104077 ) ) ;
#181068=DIRECTION ( 'NONE',  ( -1.000000000000000000, 0.000000000000000000, 0.000000000000000000 ) ) ;
#181089=CARTESIAN_POINT ( 'NONE',  ( -5.945206945974415014, -6.768871089493145199, -63.97253992123162902 ) ) ;
#181094=ORIENTED_EDGE ( 'NONE', *, *, #15986, .F. ) ;
#181113=CARTESIAN_POINT ( 'NONE',  ( -6.837149423127150349, 5.759383325533883990, -63.98874707071205847 ) ) ;
#181177=DIRECTION ( 'NONE',  ( 1.000000000000000000, 0.000000000000000000, 3.469446951953612217E-15 ) ) ;
#181196=EDGE_CURVE ( 'NONE', #182074, #117961, #119342, .T. ) ;
#181214=DIRECTION ( 'NONE',  ( -0.3041824702427698979, 0.9526137857479317628, -0.000000000000000000 ) ) ;
#181223=CARTESIAN_POINT ( 'NONE',  ( -2.500000000000000000, 3.061616997868383141E-16, -64.92179855667829713 ) ) ;
#181316=CARTESIAN_POINT ( 'NONE',  ( -19.99999999999998224, -188.0000000000000000, -25.00000000000000000 ) ) ;
#181327=ORIENTED_EDGE ( 'NONE', *, *, #53259, .F. ) ;
#181330=CARTESIAN_POINT ( 'NONE',  ( 30.74264578624799782, 22.33583958711400541, -4.800000000000000711 ) ) ;
#181335=CARTESIAN_POINT ( 'NONE',  ( 1.315892071381018269, 15.92644080175540466, -59.47647726036166915 ) ) ;
#181340=DIRECTION ( 'NONE',  ( 0.000000000000000000, 0.000000000000000000, 1.000000000000000000 ) ) ;
#181346=DIRECTION ( 'NONE',  ( 0.000000000000000000, 0.000000000000000000, -1.000000000000000000 ) ) ;
#181354=EDGE_CURVE ( 'NONE', #73091, #53519, #25268, .T. ) ;
#181360=ORIENTED_EDGE ( 'NONE', *, *, #9668, .T. ) ;
#181386=CARTESIAN_POINT ( 'NONE',  ( -5.950531402560715689E-15, 38.81732327939063509, -5.124999997268813168 ) ) ;
#181419=CARTESIAN_POINT ( 'NONE',  ( -4.000000000000000888, -105.0000000000000000, -23.00000000000000000 ) ) ;
#181441=B_SPLINE_CURVE_WITH_KNOTS ( 'NONE', 3,
 ( #64385, #49220, #66366, #3690, #142207, #36020, #126053, #160372, #37018, #95706, #129016, #87275 ),
 .UNSPECIFIED., .F., .F.,
 ( 4, 2, 2, 2, 2, 4 ),
 ( 0.002654191900342570219, 0.003314442422523698230, 0.003974692944704825807, 0.004634943466885954252, 0.004965068727976518909, 0.005295193989067083565 ),
 .UNSPECIFIED. ) ;
#181464=LINE ( 'NONE', #29749, #53430 ) ;
#181510=ORIENTED_EDGE ( 'NONE', *, *, #183088, .T. ) ;
#181556=VERTEX_POINT ( 'NONE', #150680 ) ;
#181559=CARTESIAN_POINT ( 'NONE',  ( -29.86685920354755552, 21.69954338932564397, -8.824999997268815122 ) ) ;
#181578=CYLINDRICAL_SURFACE ( 'NONE', #160240, 1.499999999999997780 ) ;
#181589=EDGE_CURVE ( 'NONE', #165759, #179372, #146944, .T. ) ;
#181594=VERTEX_POINT ( 'NONE', #77780 ) ;
#181731=ORIENTED_EDGE ( 'NONE', *, *, #1190, .T. ) ;
#181747=B_SPLINE_CURVE_WITH_KNOTS ( 'NONE', 3,
 ( #86038, #120354, #41549, #9212, #43532, #54701, #102211, #72890, #118386, #134558, #146702, #196246, #12220, #39530, #119385, #103212, #42543, #180080, #23376, #178062, #104206, #88027 ),
 .UNSPECIFIED., .F., .F.,
 ( 4, 2, 2, 2, 2, 2, 2, 2, 2, 2, 4 ),
 ( 2.778238173776314926E-07, 0.0007557225233028428031, 0.001511167222788308093, 0.002266611922273773384, 0.003022056621759238240, 0.003777501321244703530, 0.004532946020730169688, 0.004910668370472905803, 0.005288390720215642785, 0.005666113069958378899, 0.006043835419701115881 ),
 .UNSPECIFIED. ) ;
#181761=DIRECTION ( 'NONE',  ( 1.000000000000000000, 0.000000000000000000, 0.000000000000000000 ) ) ;
#181762=AXIS2_PLACEMENT_3D ( 'NONE', #107961, #169648, #121152 ) ;
#181791=ORIENTED_EDGE ( 'NONE', *, *, #105844, .F. ) ;
#181793=ORIENTED_EDGE ( 'NONE', *, *, #47633, .T. ) ;
#181800=CARTESIAN_POINT ( 'NONE',  ( -29.86685920354755197, -21.69954338932560134, -2.924999997268813878 ) ) ;
#181804=EDGE_CURVE ( 'NONE', #123761, #118127, #168782, .T. ) ;
#181814=CARTESIAN_POINT ( 'NONE',  ( -11.95556478057400973, 11.66180171105670027, -59.13370768023891344 ) ) ;
#181818=CARTESIAN_POINT ( 'NONE',  ( -1.282731051913078346, -29.61737564226529074, -51.85482277101433368 ) ) ;
#181825=CARTESIAN_POINT ( 'NONE',  ( -21.94104750614014065, 1.245073757423197369, -58.42286556281733567 ) ) ;
#181851=CARTESIAN_POINT ( 'NONE',  ( 11.40812507854754365, 35.11059874428196537, -3.724999997268813701 ) ) ;
#181852=CARTESIAN_POINT ( 'NONE',  ( -0.9841389949900990475, -21.65131445265850019, -58.61993113718296655 ) ) ;
#181872=CARTESIAN_POINT ( 'NONE',  ( -23.17010908001108405, -32.51358278116562417, -22.50838357034306014 ) ) ;
#181873=ORIENTED_EDGE ( 'NONE', *, *, #55568, .T. ) ;
#181887=CARTESIAN_POINT ( 'NONE',  ( 24.11542121825894114, -0.7284999611695349708, -54.35861002160293509 ) ) ;
#181899=CARTESIAN_POINT ( 'NONE',  ( 7.794767548047360606, -1.499903966022425816, -64.20498622968423774 ) ) ;
#181969=EDGE_LOOP ( 'NONE', ( #106986, #44912 ) ) ;
#181984=DIRECTION ( 'NONE',  ( 0.000000000000000000, 0.000000000000000000, -1.000000000000000000 ) ) ;
#182000=CARTESIAN_POINT ( 'NONE',  ( -5.773958127069001911, 3.915344532211590067, -62.35465819465156301 ) ) ;
#182004=CARTESIAN_POINT ( 'NONE',  ( -25.05471026796672618, -28.22563722313813983, -20.55515279800755479 ) ) ;
#182008=CARTESIAN_POINT ( 'NONE',  ( -9.687362902255795660, -9.687362902255630459, -60.44446360152740993 ) ) ;
#182042=LINE ( 'NONE', #26381, #185145 ) ;
#182051=CARTESIAN_POINT ( 'NONE',  ( -7.656827144875921753, -71.74905178543390605, -15.00000000000000178 ) ) ;
#182069=CARTESIAN_POINT ( 'NONE',  ( 7.776400214313169634, -46.08030136692364920, -22.42299576004354833 ) ) ;
#182074=VERTEX_POINT ( 'NONE', #128251 ) ;
#182123=EDGE_CURVE ( 'NONE', #120381, #27708, #91413, .T. ) ;
#182137=CARTESIAN_POINT ( 'NONE',  ( 17.62203461105334767, -16.12203461105336189, -54.55577602037946150 ) ) ;
#182196=CARTESIAN_POINT ( 'NONE',  ( -9.090093023806474548, 0.1983487321477290510, -63.95305636720455311 ) ) ;
#182251=ORIENTED_EDGE ( 'NONE', *, *, #120148, .T. ) ;
#182283=COLOUR_RGB ( '', 0.31764706, 0.68627451, 0.89019608) ;
#182295=CARTESIAN_POINT ( 'NONE',  ( 13.90528855463211677, -0.7844626028950130170, -60.35633530387646317 ) ) ;
#182299=LINE ( 'NONE', #88277, #101872 ) ;
#182315=CARTESIAN_POINT ( 'NONE',  ( -11.74264578624800670, 36.14014761921585972, -4.400000000000000355 ) ) ;
#182320=EDGE_CURVE ( 'NONE', #139989, #161460, #18478, .T. ) ;
#182321=FACE_OUTER_BOUND ( 'NONE', #61858, .T. ) ;
#182326=DIRECTION ( 'NONE',  ( -0.000000000000000000, -0.000000000000000000, 1.000000000000000000 ) ) ;
#182346=VERTEX_POINT ( 'NONE', #114071 ) ;
#182422=VECTOR ( 'NONE', #87282, 1000.000000000000000 ) ;
#182457=CARTESIAN_POINT ( 'NONE',  ( 17.02389920581777716, 17.34149035984847131, -54.21489346206828230 ) ) ;
#182492=EDGE_CURVE ( 'NONE', #196503, #144904, #9440, .T. ) ;
#182493=ORIENTED_EDGE ( 'NONE', *, *, #48581, .F. ) ;
#182498=TOROIDAL_SURFACE ( 'NONE', #8114, 206.0437394197456911, 10.00000000000000000 ) ;
#182506=CARTESIAN_POINT ( 'NONE',  ( -23.38845648566745794, -29.41134498177912704, -18.89001425235596088 ) ) ;
#182512=ORIENTED_EDGE ( 'NONE', *, *, #5788, .F. ) ;
#182523=CARTESIAN_POINT ( 'NONE',  ( -20.28159948851298822, -33.49867931359609941, -17.64937754809734827 ) ) ;
#182537=CARTESIAN_POINT ( 'NONE',  ( -3.573655867282028392E-15, 2.428612866367529932E-14, -25.00000000000000000 ) ) ;
#182543=VERTEX_POINT ( 'NONE', #180782 ) ;
#182546=CARTESIAN_POINT ( 'NONE',  ( -36.91746825000000598, 2.428612866367529932E-14, -6.624999997268814056 ) ) ;
#182565=CARTESIAN_POINT ( 'NONE',  ( 7.587788125977466436, -46.88744275388935989, -24.49805083758646873 ) ) ;
#182605=ORIENTED_EDGE ( 'NONE', *, *, #147752, .T. ) ;
#182679=EDGE_LOOP ( 'NONE', ( #161111, #4160, #91481, #82958 ) ) ;
#182692=EDGE_CURVE ( 'NONE', #44348, #47952, #138227, .T. ) ;
#182724=ADVANCED_FACE ( 'NONE', ( #87740 ), #12911, .F. ) ;
#182735=AXIS2_PLACEMENT_3D ( 'NONE', #176814, #40279, #8956 ) ;
#182755=DIRECTION ( 'NONE',  ( 1.000000000000000000, 0.000000000000000000, 0.000000000000000000 ) ) ;
#182785=ORIENTED_EDGE ( 'NONE', *, *, #8030, .T. ) ;
#182793=CARTESIAN_POINT ( 'NONE',  ( 11.40812507854754365, 35.11059874428196537, -5.724999997268812812 ) ) ;
#182806=CARTESIAN_POINT ( 'NONE',  ( -10.97788116290294447, 9.262594875851808851, -60.18097545586277874 ) ) ;
#182810=CARTESIAN_POINT ( 'NONE',  ( 0.000000000000000000, 0.000000000000000000, -25.00000000000000000 ) ) ;
#182818=CARTESIAN_POINT ( 'NONE',  ( -24.20670376297026749, 0.5310992180249298755, -56.83968087238906719 ) ) ;
#182833=CARTESIAN_POINT ( 'NONE',  ( 0.000000000000000000, 0.000000000000000000, -49.13275782002545355 ) ) ;
#182843=CARTESIAN_POINT ( 'NONE',  ( -36.91746825000000598, -11.99521256947794789, -9.024999997268812635 ) ) ;
#182860=ORIENTED_EDGE ( 'NONE', *, *, #40254, .F. ) ;
#182866=CARTESIAN_POINT ( 'NONE',  ( -27.73791293435188621, -28.12602025316166632, -18.50562026185692943 ) ) ;
#182880=DIRECTION ( 'NONE',  ( -1.000000000000000000, 0.000000000000000000, 0.000000000000000000 ) ) ;
#182887=CARTESIAN_POINT ( 'NONE',  ( -5.000000000000003553, -4.999999999999996447, -18.00000000000000000 ) ) ;
#182996=CARTESIAN_POINT ( 'NONE',  ( 1.398757915179067002, 29.85213727369407266, -48.47147718930269633 ) ) ;
#183033=CARTESIAN_POINT ( 'NONE',  ( -6.691772886347780336, 1.197744245042939859, -62.38710104649955923 ) ) ;
#183061=CARTESIAN_POINT ( 'NONE',  ( 9.444085519387883210, -44.71325174467972374, -21.93802053968663657 ) ) ;
#183088=EDGE_CURVE ( 'NONE', #125361, #59792, #199187, .T. ) ;
#183130=DIRECTION ( 'NONE',  ( 1.000000000000000000, 0.000000000000000000, 0.000000000000000000 ) ) ;
#183153=ORIENTED_EDGE ( 'NONE', *, *, #26840, .T. ) ;
#183185=LINE ( 'NONE', #153821, #108663 ) ;
#183191=CARTESIAN_POINT ( 'NONE',  ( -9.051314012904519757, 0.3916721525566201900, -63.96062167512634034 ) ) ;
#183247=VERTEX_POINT ( 'NONE', #135268 ) ;
#183262=EDGE_CURVE ( 'NONE', #125394, #120381, #29077, .T. ) ;
#183279=CARTESIAN_POINT ( 'NONE',  ( 21.71309667856398917, -34.72214947970702781, -18.33762378602110843 ) ) ;
#183284=CARTESIAN_POINT ( 'NONE',  ( -0.8180345313831235421, -24.06132300323554674, -54.40060964255545173 ) ) ;
#183300=ORIENTED_EDGE ( 'NONE', *, *, #66112, .T. ) ;
#183303=CARTESIAN_POINT ( 'NONE',  ( -23.48529157249600985, 32.32473071737754111, -4.299999999999999822 ) ) ;
#183329=CARTESIAN_POINT ( 'NONE',  ( 18.37348032456297275, -33.26197007282152640, -21.07589179612142161 ) ) ;
#183353=EDGE_CURVE ( 'NONE', #114628, #120796, #130078, .T. ) ;
#183362=ORIENTED_EDGE ( 'NONE', *, *, #119482, .F. ) ;
#183417=DIRECTION ( 'NONE',  ( 0.000000000000000000, 0.000000000000000000, 1.000000000000000000 ) ) ;
#183443=VECTOR ( 'NONE', #122293, 1000.000000000000000 ) ;
#183444=CARTESIAN_POINT ( 'NONE',  ( -20.67563680669853099, -22.75846771606805063, -50.58532599174672129 ) ) ;
#183446=DIRECTION ( 'NONE',  ( -0.000000000000000000, 0.000000000000000000, 1.000000000000000000 ) ) ;
#183494=CARTESIAN_POINT ( 'NONE',  ( -9.554919064904160209, -36.23455639189580069, -31.31948065624796840 ) ) ;
#183499=EDGE_CURVE ( 'NONE', #99831, #41082, #91698, .T. ) ;
#183509=B_SPLINE_CURVE_WITH_KNOTS ( 'NONE', 3,
 ( #56003, #24689, #139541, #109211, #25695, #199248, #77874, #194532, #108216, #47558, #86338, #168885, #102513, #123374, #122389, #124381, #184077, #1026, #30391, #169896, #31389, #73194, #93039, #62698, #164197, #60715 ),
 .UNSPECIFIED., .F., .F.,
 ( 4, 2, 2, 2, 2, 2, 2, 2, 2, 2, 2, 2, 4 ),
 ( 4.906538933386797396E-18, 0.002279955776188823027, 0.004559911552377641716, 0.006839867328566459105, 0.009119823104755278229, 0.01367973465713291821, 0.01823964620951055646, 0.02279955776188819991, 0.02735946931426583642, 0.02963942509045465468, 0.03191938086664347640, 0.03419933664283229119, 0.03647929241902110598 ),
 .UNSPECIFIED. ) ;
#183526=DIRECTION ( 'NONE',  ( 0.000000000000000000, 0.000000000000000000, 1.000000000000000000 ) ) ;
#183535=CARTESIAN_POINT ( 'NONE',  ( 3.556970738554034288E-15, -38.81732327939057114, -8.124999997268814056 ) ) ;
#183545=DIRECTION ( 'NONE',  ( 1.000000000000000000, 0.000000000000000000, 0.000000000000000000 ) ) ;
#183553=LINE ( 'NONE', #169353, #91684 ) ;
#183555=CARTESIAN_POINT ( 'NONE',  ( -9.248023074035629065, -10.74802307403544077, -62.40259441833023857 ) ) ;
#183596=ORIENTED_EDGE ( 'NONE', *, *, #15852, .F. ) ;
#183613=CIRCLE ( 'NONE', #18926, 216.0437394197456342 ) ;
#183716=ORIENTED_EDGE ( 'NONE', *, *, #74445, .T. ) ;
#183743=CYLINDRICAL_SURFACE ( 'NONE', #59540, 40.00000000000000000 ) ;
#183762=CARTESIAN_POINT ( 'NONE',  ( -1.500078752102835811, -15.01195240492206651, -59.87740586969341905 ) ) ;
#183775=ORIENTED_EDGE ( 'NONE', *, *, #188269, .T. ) ;
#183777=ORIENTED_EDGE ( 'NONE', *, *, #186584, .T. ) ;
#183783=CARTESIAN_POINT ( 'NONE',  ( -36.91746825000001309, -11.99521256947794789, -3.024999997268812635 ) ) ;
#183795=CARTESIAN_POINT ( 'NONE',  ( 4.704316316549549626, 6.719756334737494896, -62.10423353180173933 ) ) ;
#183829=CARTESIAN_POINT ( 'NONE',  ( -22.81625015709509441, -31.40387420917324590, -8.824999997268811569 ) ) ;
#183839=CARTESIAN_POINT ( 'NONE',  ( 30.11859102234670615, -23.17191052982427735, -18.99406613714113234 ) ) ;
#183846=ORIENTED_EDGE ( 'NONE', *, *, #39485, .F. ) ;
#183852=CARTESIAN_POINT ( 'NONE',  ( -34.63261191445433695, -20.08610687336648581, -21.92908410841864608 ) ) ;
#183901=CARTESIAN_POINT ( 'NONE',  ( 1.350817277425566232, 6.940587957980362432, -64.37020913546857059 ) ) ;
#183972=CIRCLE ( 'NONE', #96760, 9.100000000000001421 ) ;
#183975=CARTESIAN_POINT ( 'NONE',  ( -6.687054376293257718, 6.125853549498580186, -61.90253133708612410 ) ) ;
#183981=EDGE_CURVE ( 'NONE', #60353, #25387, #57185, .T. ) ;
#183999=FACE_OUTER_BOUND ( 'NONE', #193431, .T. ) ;
#184000=FACE_BOUND ( 'NONE', #116432, .T. ) ;
#184016=ORIENTED_EDGE ( 'NONE', *, *, #76288, .F. ) ;
#184077=CARTESIAN_POINT ( 'NONE',  ( -12.39597446193840291, -43.61540881465732156, -22.87833536075119767 ) ) ;
#184107=B_SPLINE_CURVE_WITH_KNOTS ( 'NONE', 3,
 ( #176823, #85790, #119142, #42301, #117126, #180823, #161635, #101964, #134311, #150478, #40290, #179829, #147476, #193993, #163645, #133293 ),
 .UNSPECIFIED., .F., .F.,
 ( 4, 2, 2, 2, 2, 2, 2, 4 ),
 ( 2.788259402197439630E-07, 0.0004455515445239860992, 0.0008908242631077525116, 0.001781369700275286854, 0.002226642418859052074, 0.002671915137442817077, 0.003117187856026582514, 0.003562460574610347517 ),
 .UNSPECIFIED. ) ;
#184140=CARTESIAN_POINT ( 'NONE',  ( 22.96887126817271607, -21.84138762001119716, -49.40150514669699078 ) ) ;
#184144=EDGE_LOOP ( 'NONE', ( #149977, #191957, #148457, #92289 ) ) ;
#184229=ORIENTED_EDGE ( 'NONE', *, *, #31655, .T. ) ;
#184230=DIRECTION ( 'NONE',  ( 1.000000000000000000, -1.776356839400250465E-15, 0.000000000000000000 ) ) ;
#184235=ORIENTED_EDGE ( 'NONE', *, *, #92250, .T. ) ;
#184246=CARTESIAN_POINT ( 'NONE',  ( 16.49741402511621757, -0.7792920370541633890, -61.43171317168471290 ) ) ;
#184268=CARTESIAN_POINT ( 'NONE',  ( 24.78074900657736990, -31.51706519598950607, -17.29086010071286950 ) ) ;
#184271=CARTESIAN_POINT ( 'NONE',  ( -1.344113590474603992, -22.10945809693575725, -55.87741762761908149 ) ) ;
#184292=CARTESIAN_POINT ( 'NONE',  ( 11.74264578624800315, -36.14014761921581709, -5.400000000000000355 ) ) ;
#184318=CARTESIAN_POINT ( 'NONE',  ( 20.47606263882783040, -31.78721852328014918, -20.08103504831379027 ) ) ;
#184344=ORIENTED_EDGE ( 'NONE', *, *, #7609, .T. ) ;
#184345=ORIENTED_EDGE ( 'NONE', *, *, #147079, .F. ) ;
#184348=CARTESIAN_POINT ( 'NONE',  ( 1.218433102416749181, 14.30315789272851390, -62.33600599370836193 ) ) ;
#184406=CARTESIAN_POINT ( 'NONE',  ( -1.221313414957698099E-14, 31.90000000000003411, -49.13275782002545355 ) ) ;
#184425=CYLINDRICAL_SURFACE ( 'NONE', #79266, 10.00000000000000000 ) ;
#184432=CARTESIAN_POINT ( 'NONE',  ( 15.66972982126930702, 17.56366054824405865, -54.83331888096113005 ) ) ;
#184469=ORIENTED_EDGE ( 'NONE', *, *, #51668, .F. ) ;
#184483=CARTESIAN_POINT ( 'NONE',  ( -10.65591991698828700, -43.63381331855018885, -21.52219975116658190 ) ) ;
#184505=CARTESIAN_POINT ( 'NONE',  ( 22.64533781646232669, -20.52407392197266489, -47.58305834096859854 ) ) ;
#184508=CARTESIAN_POINT ( 'NONE',  ( 37.99999999999999289, 2.428612866367529932E-14, -25.00000000000000000 ) ) ;
#184513=LINE ( 'NONE', #169325, #64604 ) ;
#184532=DIRECTION ( 'NONE',  ( 0.000000000000000000, 0.000000000000000000, 1.000000000000000000 ) ) ;
#184540=CARTESIAN_POINT ( 'NONE',  ( 6.767138868728925338, -40.03474714072476814, -25.59093536067049612 ) ) ;
#184580=B_SPLINE_CURVE_WITH_KNOTS ( 'NONE', 3,
 ( #16413, #78060, #153923, #139728, #15417, #77075, #28624, #59921, #13433, #75097 ),
 .UNSPECIFIED., .F., .F.,
 ( 4, 2, 2, 2, 4 ),
 ( 2.788292365864085830E-07, 0.0002942923369301741164, 0.0005883058446237618942, 0.0008823193523173495636, 0.001176332860010937233 ),
 .UNSPECIFIED. ) ;
#184630=VECTOR ( 'NONE', #29440, 1000.000000000000000 ) ;
#184713=EDGE_CURVE ( 'NONE', #181594, #145515, #101082, .T. ) ;
#184754=CYLINDRICAL_SURFACE ( 'NONE', #124348, 1.499999999999997780 ) ;
#184769=CARTESIAN_POINT ( 'NONE',  ( 11.40812507854754365, 35.11059874428196537, -1.724999997268813479 ) ) ;
#184782=CARTESIAN_POINT ( 'NONE',  ( 2.500000000000000000, 0.000000000000000000, -65.00100000000003320 ) ) ;
#184792=CARTESIAN_POINT ( 'NONE',  ( -23.88070017481512508, 1.044764468832944493, -57.07230391339724207 ) ) ;
#184821=CARTESIAN_POINT ( 'NONE',  ( 0.7567881333757656703, 8.898838318008483128, -63.99035486850526411 ) ) ;
#184844=ORIENTED_EDGE ( 'NONE', *, *, #103523, .T. ) ;
#184936=ORIENTED_EDGE ( 'NONE', *, *, #36648, .T. ) ;
#184971=DIRECTION ( 'NONE',  ( 0.000000000000000000, 0.000000000000000000, -1.000000000000000000 ) ) ;
#184994=ADVANCED_FACE ( 'NONE', ( #68337 ), #53168, .F. ) ;
#185030=DIRECTION ( 'NONE',  ( 1.000000000000000000, 0.000000000000000000, 0.000000000000000000 ) ) ;
#185041=ORIENTED_EDGE ( 'NONE', *, *, #47644, .T. ) ;
#185061=CARTESIAN_POINT ( 'NONE',  ( -4.896406352259377925, 3.948644494436257979, -64.50244604205114740 ) ) ;
#185073=VERTEX_POINT ( 'NONE', #194707 ) ;
#185106=DIRECTION ( 'NONE',  ( 0.000000000000000000, 0.000000000000000000, -1.000000000000000000 ) ) ;
#185145=VECTOR ( 'NONE', #132541, 1000.000000000000000 ) ;
#185158=DIRECTION ( 'NONE',  ( 0.000000000000000000, 0.000000000000000000, 1.000000000000000000 ) ) ;
#185168=CARTESIAN_POINT ( 'NONE',  ( -8.636255518948912524, -38.40306468563544939, -32.12764100183819949 ) ) ;
#185218=ORIENTED_EDGE ( 'NONE', *, *, #191742, .F. ) ;
#185221=EDGE_LOOP ( 'NONE', ( #166340, #103843, #86007, #48374, #15915, #196326, #81059, #63098, #20704, #149020, #13738, #19588, #22401, #89851 ) ) ;
#185223=CARTESIAN_POINT ( 'NONE',  ( 30.74264578624799782, 22.33583958711400541, -8.549999994537627046 ) ) ;
#185245=B_SPLINE_CURVE_WITH_KNOTS ( 'NONE', 3,
 ( #94976, #96948, #156661, #64646, #173827, #82771, #35291, #20119, #81763, #36272, #66619, #128283, #174807, #10952, #70624, #6930, #25136, #24127, #26129, #133282, #71616, #56451, #160627, #163634 ),
 .UNSPECIFIED., .F., .F.,
 ( 4, 2, 2, 2, 2, 2, 2, 2, 2, 2, 2, 4 ),
 ( 0.000000000000000000, 0.002690955612256999523, 0.005381911224513999045, 0.008072866836771004639, 0.009418344642899506569, 0.01009108354596376447, 0.01076382244902802238, 0.01210930025515653992, 0.01345477806128506093, 0.01614573367354209601, 0.01883668928579913110, 0.02152764489805616965 ),
 .UNSPECIFIED. ) ;
#185246=CARTESIAN_POINT ( 'NONE',  ( 0.000000000000000000, 0.000000000000000000, -56.46919128290398504 ) ) ;
#185257=B_SPLINE_CURVE_WITH_KNOTS ( 'NONE', 3,
 ( #157668, #79826, #159636, #22136, #173842, #98954, #189997, #52462, #3962, #176834, #37295, #68627, #81779, #126321, #38305, #82787, #66635, #21132, #141496, #6947, #96962, #114120, #51472, #158642 ),
 .UNSPECIFIED., .F., .F.,
 ( 4, 2, 2, 2, 2, 2, 2, 2, 2, 2, 2, 4 ),
 ( 0.000000000000000000, 0.002556407831644171621, 0.005112815663288348446, 0.007669223494932524837, 0.008947427410754611732, 0.009586529368665658649, 0.01022563132657670557, 0.01150383524239879246, 0.01278203915822087589, 0.01533844698986504620, 0.01789485482150921652, 0.02045126265315338338 ),
 .UNSPECIFIED. ) ;
#185265=CARTESIAN_POINT ( 'NONE',  ( 17.62203461105333702, -16.12203461105326951, -57.08650645001478097 ) ) ;
#185279=CARTESIAN_POINT ( 'NONE',  ( -23.48529157249600985, 32.32473071737754111, -6.300000000000000711 ) ) ;
#185284=DIRECTION ( 'NONE',  ( 1.000000000000000000, 0.000000000000000000, 0.000000000000000000 ) ) ;
#185304=CARTESIAN_POINT ( 'NONE',  ( 15.59283147534792136, -34.52683219100885026, -28.07673947522060232 ) ) ;
#185322=CIRCLE ( 'NONE', #17465, 24.30000000000003268 ) ;
#185336=ORIENTED_EDGE ( 'NONE', *, *, #133615, .T. ) ;
#185345=ADVANCED_FACE ( 'NONE', ( #73365 ), #56176, .T. ) ;
#185389=CARTESIAN_POINT ( 'NONE',  ( -4.313351365237978463, -4.313351365237916291, -62.50719930893269805 ) ) ;
#185422=EDGE_CURVE ( 'NONE', #29006, #197049, #106126, .T. ) ;
#185472=CARTESIAN_POINT ( 'NONE',  ( -19.06840828309120184, -32.80151167437442439, -20.74459427421103896 ) ) ;
#185497=CARTESIAN_POINT ( 'NONE',  ( 4.313351365237949153, 4.313351365237946489, -64.53213882399992940 ) ) ;
#185530=CARTESIAN_POINT ( 'NONE',  ( 17.43506102071334496, -39.09281690108636553, -20.41854293743994120 ) ) ;
#185532=CARTESIAN_POINT ( 'NONE',  ( -9.889834268056119981, -11.98662851468406920, -61.85832361008505842 ) ) ;
#185549=ORIENTED_EDGE ( 'NONE', *, *, #111459, .T. ) ;
#185570=AXIS2_PLACEMENT_3D ( 'NONE', #43607, #164970, #26463 ) ;
#185647=ORIENTED_EDGE ( 'NONE', *, *, #189654, .T. ) ;
#185696=ORIENTED_EDGE ( 'NONE', *, *, #468, .T. ) ;
#185718=CIRCLE ( 'NONE', #50049, 206.0437394197456911 ) ;
#185724=CIRCLE ( 'NONE', #40390, 59.99999999999998579 ) ;
#185745=CARTESIAN_POINT ( 'NONE',  ( 17.44323487119282134, -16.85911479061552143, -54.24972394154876554 ) ) ;
#185748=CARTESIAN_POINT ( 'NONE',  ( -1.151164073136592192, -16.16661445520355755, -59.37042179516132023 ) ) ;
#185754=CARTESIAN_POINT ( 'NONE',  ( -21.27150294653347729, -22.98525001747979601, -46.52314187507937504 ) ) ;
#185763=VERTEX_POINT ( 'NONE', #1450 ) ;
#185772=CARTESIAN_POINT ( 'NONE',  ( 36.91746824999999177, 2.880721459617395097E-14, -2.124999997268813168 ) ) ;
#185780=DIRECTION ( 'NONE',  ( 1.000000000000000000, 0.000000000000000000, 0.000000000000000000 ) ) ;
#185785=CARTESIAN_POINT ( 'NONE',  ( 11.80868324581538253, -11.80868324581533457, -59.13370768023891344 ) ) ;
#185822=CARTESIAN_POINT ( 'NONE',  ( -22.81625015709509441, -31.40387420917324590, -10.82499999726881335 ) ) ;
#185824=CARTESIAN_POINT ( 'NONE',  ( 6.100000000000006750, 0.000000000000000000, -62.50719930893269805 ) ) ;
#185825=CARTESIAN_POINT ( 'NONE',  ( 1.314058473856374532, 8.348982836029733789, -64.09739989910906388 ) ) ;
#185826=VERTEX_POINT ( 'NONE', #186505 ) ;
#185833=CARTESIAN_POINT ( 'NONE',  ( -11.80868324581538253, 11.80868324581533457, -61.34707691135562868 ) ) ;
#185848=ORIENTED_EDGE ( 'NONE', *, *, #199458, .F. ) ;
#185866=ADVANCED_FACE ( 'NONE', ( #95451 ), #141949, .T. ) ;
#185946=CIRCLE ( 'NONE', #76088, 214.0437394197456342 ) ;
#185952=CARTESIAN_POINT ( 'NONE',  ( 1.351073136246558226, 6.941121712480402550, -62.33638022162458725 ) ) ;
#185972=DIRECTION ( 'NONE',  ( 1.000000000000000000, 0.000000000000000000, 0.000000000000000000 ) ) ;
#185978=CARTESIAN_POINT ( 'NONE',  ( -24.28759355007370857, 0.2213677808129483893, -54.22458008397516949 ) ) ;
#185979=ADVANCED_FACE ( 'NONE', ( #96437 ), #113596, .F. ) ;
#186014=ADVANCED_FACE ( 'NONE', ( #23613 ), #21603, .F. ) ;
#186027=CARTESIAN_POINT ( 'NONE',  ( 22.62413958104535183, -1.500431131851388766, -57.95367621771160316 ) ) ;
#186043=AXIS2_PLACEMENT_3D ( 'NONE', #171317, #80278, #14651 ) ;
#186104=DIRECTION ( 'NONE',  ( 0.000000000000000000, 0.000000000000000000, 1.000000000000000000 ) ) ;
#186116=CYLINDRICAL_SURFACE ( 'NONE', #108006, 38.00000000000000000 ) ;
#186137=DIRECTION ( 'NONE',  ( 0.000000000000000000, 0.000000000000000000, 1.000000000000000000 ) ) ;
#186171=CARTESIAN_POINT ( 'NONE',  ( 11.74264578624799427, 36.14014761921585972, -4.349999994537626868 ) ) ;
#186190=VECTOR ( 'NONE', #198117, 1000.000000000000000 ) ;
#186227=EDGE_CURVE ( 'NONE', #111780, #177280, #50374, .T. ) ;
#186290=CARTESIAN_POINT ( 'NONE',  ( 23.48529157249600630, -32.32473071737749137, -9.300000000000002487 ) ) ;
#186300=DIRECTION ( 'NONE',  ( -1.000000000000000000, 0.000000000000000000, 0.000000000000000000 ) ) ;
#186314=CARTESIAN_POINT ( 'NONE',  ( 22.83040865997484303, -30.22555755525017673, -21.93998231254684583 ) ) ;
#186434=CARTESIAN_POINT ( 'NONE',  ( 14.91361452257043929, 15.22666363356478492, -56.46021433273639900 ) ) ;
#186482=AXIS2_PLACEMENT_3D ( 'NONE', #39526, #148719, #178058 ) ;
#186487=CARTESIAN_POINT ( 'NONE',  ( -33.23029939923285525, -20.96646023091586386, -17.75854212242423102 ) ) ;
#186505=CARTESIAN_POINT ( 'NONE',  ( 1.500000000000008438, 22.80000000000002913, -57.83153971412246364 ) ) ;
#186507=AXIS2_PLACEMENT_3D ( 'NONE', #61887, #32567, #65871 ) ;
#186519=CARTESIAN_POINT ( 'NONE',  ( 22.34691611882956863, -20.25371774921029200, -51.27624273403993982 ) ) ;
#186538=CARTESIAN_POINT ( 'NONE',  ( 36.91746824999999177, 2.880721459617395097E-14, -5.624999997268813168 ) ) ;
#186546=CARTESIAN_POINT ( 'NONE',  ( -3.573655867282028392E-15, 2.428612866367529932E-14, -15.00000000000000000 ) ) ;
#186548=CARTESIAN_POINT ( 'NONE',  ( 26.72240360495968758, -29.37940146934077035, -20.20861161914950799 ) ) ;
#186550=CARTESIAN_POINT ( 'NONE',  ( -10.85841070881430959, -12.25138988246575167, -61.49687578711335334 ) ) ;
#186567=VERTEX_POINT ( 'NONE', #160116 ) ;
#186584=EDGE_CURVE ( 'NONE', #151987, #15377, #76186, .T. ) ;
#186586=FACE_OUTER_BOUND ( 'NONE', #12187, .T. ) ;
#186664=ORIENTED_EDGE ( 'NONE', *, *, #42100, .T. ) ;
#186669=LINE ( 'NONE', #140125, #82342 ) ;
#186777=B_SPLINE_CURVE_WITH_KNOTS ( 'NONE', 3,
 ( #16652, #81271, #93473, #1462, #158137, #189486 ),
 .UNSPECIFIED., .F., .F.,
 ( 4, 2, 4 ),
 ( 0.003557987005820478950, 0.004145727928114205374, 0.004733468850407931798 ),
 .UNSPECIFIED. ) ;
#186778=EDGE_LOOP ( 'NONE', ( #64679, #77127, #164358, #118414 ) ) ;
#186784=CARTESIAN_POINT ( 'NONE',  ( -11.40812507854754720, -35.11059874428192273, -10.72499999726881548 ) ) ;
#186821=LINE ( 'NONE', #48291, #18231 ) ;
#186829=ORIENTED_EDGE ( 'NONE', *, *, #70721, .F. ) ;
#186836=CARTESIAN_POINT ( 'NONE',  ( -36.91746825000000598, 2.428612866367529932E-14, -7.124999997268813168 ) ) ;
#186837=ADVANCED_FACE ( 'NONE', ( #57947 ), #85868, .F. ) ;
#186845=CARTESIAN_POINT ( 'NONE',  ( 10.46900522708367198, -36.04764466666197364, -30.96889465344744607 ) ) ;
#186918=EDGE_CURVE ( 'NONE', #120796, #111025, #18051, .T. ) ;
#186921=CARTESIAN_POINT ( 'NONE',  ( 0.000000000000000000, 0.000000000000000000, -65.00100000000003320 ) ) ;
#186944=DIRECTION ( 'NONE',  ( 1.000000000000000000, 0.000000000000000000, 0.000000000000000000 ) ) ;
#186986=CARTESIAN_POINT ( 'NONE',  ( 1.065438805247536314, 29.32802529041667228, -49.14125557145903400 ) ) ;
#186988=CARTESIAN_POINT ( 'NONE',  ( -9.396639952208071023, -10.08966692039653523, -60.41061585848335369 ) ) ;
#187024=CARTESIAN_POINT ( 'NONE',  ( -38.00000000000000711, 2.428612866367529932E-14, -5.749999994537626336 ) ) ;
#187032=AXIS2_PLACEMENT_3D ( 'NONE', #198452, #57960, #119631 ) ;
#187058=ORIENTED_EDGE ( 'NONE', *, *, #98810, .F. ) ;
#187121=CARTESIAN_POINT ( 'NONE',  ( -0.9205664139720410866, -8.788389965099099754, -61.95844424577440179 ) ) ;
#187157=FACE_OUTER_BOUND ( 'NONE', #28130, .T. ) ;
#187237=FACE_OUTER_BOUND ( 'NONE', #199640, .T. ) ;
#187271=DIRECTION ( 'NONE',  ( -1.000000000000000000, 0.000000000000000000, 0.000000000000000000 ) ) ;
#187273=CARTESIAN_POINT ( 'NONE',  ( 22.55670631985092456, -22.55670631985084995, -45.64921306006598201 ) ) ;
#187315=CARTESIAN_POINT ( 'NONE',  ( 24.21728366753059802, -29.00647930567947341, -20.95994360447972582 ) ) ;
#187332=AXIS2_PLACEMENT_3D ( 'NONE', #143410, #4898, #55405 ) ;
#187341=ORIENTED_EDGE ( 'NONE', *, *, #130602, .F. ) ;
#187345=ORIENTED_EDGE ( 'NONE', *, *, #84741, .F. ) ;
#187355=CARTESIAN_POINT ( 'NONE',  ( 37.99999999999999289, 2.893978650043524126E-14, -10.74999999453762811 ) ) ;
#187404=CYLINDRICAL_SURFACE ( 'NONE', #32444, 1.499999999999997780 ) ;
#187428=CARTESIAN_POINT ( 'NONE',  ( 10.51869806896810822, 12.24338688535743280, -59.40202214942378589 ) ) ;
#187469=ORIENTED_EDGE ( 'NONE', *, *, #89537, .T. ) ;
#187476=CIRCLE ( 'NONE', #155123, 40.00000000000002132 ) ;
#187478=EDGE_CURVE ( 'NONE', #42359, #140931, #127287, .T. ) ;
#187504=CARTESIAN_POINT ( 'NONE',  ( -30.74264578624800492, -22.33583958711396278, -9.799999999999998934 ) ) ;
#187510=EDGE_CURVE ( 'NONE', #56919, #116695, #111137, .T. ) ;
#187532=CARTESIAN_POINT ( 'NONE',  ( 11.40812507854755253, -35.11059874428192273, -2.024999997268813079 ) ) ;
#187541=CARTESIAN_POINT ( 'NONE',  ( 27.67003201002207291, -28.46598819372293931, -20.09023003179317257 ) ) ;
#187591=CARTESIAN_POINT ( 'NONE',  ( -29.86685920354755552, 21.69954338932564397, -2.824999997268813345 ) ) ;
#187595=DIRECTION ( 'NONE',  ( -0.000000000000000000, -0.000000000000000000, 1.000000000000000000 ) ) ;
#187617=CARTESIAN_POINT ( 'NONE',  ( 3.503282210674363295, -48.86437366581479580, -23.00000000000000000 ) ) ;
#187624=CARTESIAN_POINT ( 'NONE',  ( -37.45873412500000654, 2.428612866367529932E-14, -0.3124999986344065839 ) ) ;
#187734=DIRECTION ( 'NONE',  ( 1.000000000000000000, 0.000000000000000000, 0.000000000000000000 ) ) ;
#187746=EDGE_CURVE ( 'NONE', #156506, #74887, #78806, .T. ) ;
#187759=CARTESIAN_POINT ( 'NONE',  ( 0.1103826470145124194, 21.30000000000002558, -58.85720012050614258 ) ) ;
#187772=CARTESIAN_POINT ( 'NONE',  ( -36.91746825000000598, 2.428612866367529932E-14, -7.124999997268813168 ) ) ;
#187821=CARTESIAN_POINT ( 'NONE',  ( -29.86685920354755197, -21.69954338932560134, -2.924999997268813878 ) ) ;
#187829=CARTESIAN_POINT ( 'NONE',  ( -11.16688150046374339, 9.295088167215947550, -62.26853652665834460 ) ) ;
#187837=ORIENTED_EDGE ( 'NONE', *, *, #171883, .T. ) ;
#187879=ADVANCED_FACE ( 'NONE', ( #51455 ), #60028, .F. ) ;
#187908=CARTESIAN_POINT ( 'NONE',  ( 22.55670631985092811, 22.55670631985084640, -64.92279855667830191 ) ) ;
#187947=CARTESIAN_POINT ( 'NONE',  ( 11.30153831258470731, -180.0000000000000000, 0.000000000000000000 ) ) ;
#187972=CARTESIAN_POINT ( 'NONE',  ( -21.94965239947789826, 1.250870343808954788, -55.99511580764671237 ) ) ;
#188006=CARTESIAN_POINT ( 'NONE',  ( -11.74264578624800670, 36.14014761921585972, -2.149999994537626691 ) ) ;
#188089=CARTESIAN_POINT ( 'NONE',  ( -3.573655867282028392E-15, 2.428612866367529932E-14, -25.00000000000000000 ) ) ;
#188093=CARTESIAN_POINT ( 'NONE',  ( -38.00000000000000711, -12.34694845685042708, -9.649999994537626691 ) ) ;
#188107=EDGE_CURVE ( 'NONE', #92192, #38777, #108737, .T. ) ;
#188125=DIRECTION ( 'NONE',  ( -0.1178549842436473205, -0.9930308165857339997, 6.133374237849951452E-17 ) ) ;
#188131=EDGE_CURVE ( 'NONE', #51008, #88773, #185245, .T. ) ;
#188177=EDGE_CURVE ( 'NONE', #132572, #157648, #169863, .T. ) ;
#188218=ORIENTED_EDGE ( 'NONE', *, *, #84003, .F. ) ;
#188229=CARTESIAN_POINT ( 'NONE',  ( 1.053409450988196827, 23.87225889828500058, -54.54687963008630192 ) ) ;
#188251=FACE_OUTER_BOUND ( 'NONE', #176100, .T. ) ;
#188258=FACE_OUTER_BOUND ( 'NONE', #136044, .T. ) ;
#188269=EDGE_CURVE ( 'NONE', #106915, #59419, #82664, .T. ) ;
#188271=AXIS2_PLACEMENT_3D ( 'NONE', #51579, #127417, #94095 ) ;
#188273=CARTESIAN_POINT ( 'NONE',  ( 38.00000000000000000, 12.34694845685046616, -8.899999999999996803 ) ) ;
#188296=CARTESIAN_POINT ( 'NONE',  ( 28.03958666231585184, -24.95204343637638900, -18.68191426762921736 ) ) ;
#188332=VECTOR ( 'NONE', #97690, 1000.000000000000000 ) ;
#188361=EDGE_CURVE ( 'NONE', #63287, #153996, #73052, .T. ) ;
#188363=CARTESIAN_POINT ( 'NONE',  ( 6.691772886347784777, -1.197744245042889011, -62.38710104649955213 ) ) ;
#188406=CARTESIAN_POINT ( 'NONE',  ( 11.10918730048722836, 12.21811429388709946, -59.22494048452016102 ) ) ;
#188408=DIRECTION ( 'NONE',  ( -1.000000000000000000, 0.000000000000000000, 0.000000000000000000 ) ) ;
#188417=AXIS2_PLACEMENT_3D ( 'NONE', #159994, #3323, #96319 ) ;
#188459=CARTESIAN_POINT ( 'NONE',  ( -28.03958666231389074, -24.95204343637547240, -18.68191426763402063 ) ) ;
#188468=ADVANCED_FACE ( 'NONE', ( #116121 ), #192972, .T. ) ;
#188477=AXIS2_PLACEMENT_3D ( 'NONE', #197476, #58942, #102466 ) ;
#188484=CARTESIAN_POINT ( 'NONE',  ( 20.59158986795031865, -20.29504437421338636, -49.65986060686195458 ) ) ;
#188508=ORIENTED_EDGE ( 'NONE', *, *, #146334, .F. ) ;
#188511=CARTESIAN_POINT ( 'NONE',  ( 36.91746824999999177, 2.880721459617395097E-14, -3.624999997268813168 ) ) ;
#188521=CARTESIAN_POINT ( 'NONE',  ( 26.35186391108388548, -29.45501048290770640, -18.59600737859850739 ) ) ;
#188540=ORIENTED_EDGE ( 'NONE', *, *, #76322, .T. ) ;
#188567=AXIS2_PLACEMENT_3D ( 'NONE', #159199, #81352, #6515 ) ;
#188573=CARTESIAN_POINT ( 'NONE',  ( -22.81625015709509441, -31.40387420917324590, -10.82499999726881157 ) ) ;
#188593=DIRECTION ( 'NONE',  ( -0.000000000000000000, -0.000000000000000000, -1.000000000000000000 ) ) ;
#188608=CARTESIAN_POINT ( 'NONE',  ( 11.74264578624800315, -36.14014761921581709, -1.399999999999999689 ) ) ;
#188659=CIRCLE ( 'NONE', #36779, 12.50000000000000000 ) ;
#188707=VERTEX_POINT ( 'NONE', #178809 ) ;
#188736=CARTESIAN_POINT ( 'NONE',  ( 0.6709015534586495466, 8.945245563437705272, -61.92617404244804646 ) ) ;
#188759=CARTESIAN_POINT ( 'NONE',  ( -22.81625015709510507, 31.40387420917330275, -9.424999997268812990 ) ) ;
#188809=CARTESIAN_POINT ( 'NONE',  ( -29.86685920354755197, -21.69954338932560134, -6.924999997268813878 ) ) ;
#188816=CARTESIAN_POINT ( 'NONE',  ( -9.839468975293884867, 9.550175731184090466, -62.57644703671204667 ) ) ;
#188824=ORIENTED_EDGE ( 'NONE', *, *, #132574, .F. ) ;
#188843=VERTEX_POINT ( 'NONE', #118130 ) ;
#188873=CONICAL_SURFACE ( 'NONE', #50009, 2.500000000000000000, 1.029744258676656976 ) ;
#188878=ADVANCED_FACE ( 'NONE', ( #84765 ), #175806, .F. ) ;
#188892=VECTOR ( 'NONE', #175552, 1000.000000000000000 ) ;
#188903=LINE ( 'NONE', #23026, #1280 ) ;
#188909=AXIS2_PLACEMENT_3D ( 'NONE', #160124, #128772, #84264 ) ;
#188934=VERTEX_POINT ( 'NONE', #99940 ) ;
#188944=CARTESIAN_POINT ( 'NONE',  ( 0.3967178197656787142, 6.139882670400419684, -62.49912032061806855 ) ) ;
#188962=FACE_OUTER_BOUND ( 'NONE', #186778, .T. ) ;
#188966=LINE ( 'NONE', #2931, #95041 ) ;
#188984=CARTESIAN_POINT ( 'NONE',  ( -30.58708291193883255, 1.497147075633844526, -50.73425184351846440 ) ) ;
#188996=ORIENTED_EDGE ( 'NONE', *, *, #5508, .F. ) ;
#189002=CARTESIAN_POINT ( 'NONE',  ( -38.00000000000001421, 12.34694845685046438, -3.849999994537626868 ) ) ;
#189012=CARTESIAN_POINT ( 'NONE',  ( -19.24578484527059175, -180.9428398739491684, -25.00000000000000000 ) ) ;
#189015=CARTESIAN_POINT ( 'NONE',  ( -0.7913989229878302112, -31.67901979315911021, -49.40962234820035093 ) ) ;
#189030=AXIS2_PLACEMENT_3D ( 'NONE', #1092, #124449, #136305 ) ;
#189036=ORIENTED_EDGE ( 'NONE', *, *, #80402, .T. ) ;
#189073=CARTESIAN_POINT ( 'NONE',  ( -6.300487686722341607, -38.77208804323718283, -32.75369354553867396 ) ) ;
#189095=CARTESIAN_POINT ( 'NONE',  ( 0.000000000000000000, 0.000000000000000000, -15.00000000000000000 ) ) ;
#189105=CARTESIAN_POINT ( 'NONE',  ( -40.00000000000000711, 2.918471586026471156E-14, -25.00000000000000000 ) ) ;
#189165=CARTESIAN_POINT ( 'NONE',  ( -13.99740082693642229, -37.19577201402449163, -29.83961662117135560 ) ) ;
#189218=CYLINDRICAL_SURFACE ( 'NONE', #1762, 1.500000000000001332 ) ;
#189248=ADVANCED_FACE ( 'NONE', ( #197952 ), #89772, .F. ) ;
#189257=DIRECTION ( 'NONE',  ( 1.000000000000000000, 0.000000000000000000, 3.469446951953612217E-15 ) ) ;
#189261=AXIS2_PLACEMENT_3D ( 'NONE', #55485, #83806, #191996 ) ;
#189263=CARTESIAN_POINT ( 'NONE',  ( -16.08916976210838001, 1.211883243535291088, -59.40465844715060229 ) ) ;
#189290=( NAMED_UNIT ( * ) PLANE_ANGLE_UNIT ( ) SI_UNIT ( $, .RADIAN. ) );
#189294=CARTESIAN_POINT ( 'NONE',  ( 29.42957871419392291, -23.46871120496999552, -19.15262919804625241 ) ) ;
#189360=CARTESIAN_POINT ( 'NONE',  ( 6.615873399348748407, -1.136345303629790804, -62.40252569733545585 ) ) ;
#189403=DIRECTION ( 'NONE',  ( -0.000000000000000000, -0.000000000000000000, 1.000000000000000000 ) ) ;
#189446=EDGE_LOOP ( 'NONE', ( #17038, #88665, #82278, #189036 ) ) ;
#189478=CARTESIAN_POINT ( 'NONE',  ( -29.20736712825161163, 0.9155518048966417854, -49.29216761470104302 ) ) ;
#189481=CARTESIAN_POINT ( 'NONE',  ( 6.126184129041763349, 6.686840650406337794, -63.95889547717843726 ) ) ;
#189484=FACE_OUTER_BOUND ( 'NONE', #108223, .T. ) ;
#189486=CARTESIAN_POINT ( 'NONE',  ( 6.434671708797603529, -6.434671708797564449, -63.95112321872120731 ) ) ;
#189495=CARTESIAN_POINT ( 'NONE',  ( -1.022580077288041090E-15, -16.70000000000002061, -61.34707691135562868 ) ) ;
#189504=CARTESIAN_POINT ( 'NONE',  ( -22.81625015709510507, 31.40387420917330275, -0.9249999972688132122 ) ) ;
#189508=AXIS2_PLACEMENT_3D ( 'NONE', #102918, #103919, #182755 ) ;
#189516=CARTESIAN_POINT ( 'NONE',  ( 27.14096102835587132, -28.70429377953545469, -18.51261060099296785 ) ) ;
#189567=CARTESIAN_POINT ( 'NONE',  ( 29.86685920354754487, 21.69954338932564752, -7.924999997268814766 ) ) ;
#189568=CARTESIAN_POINT ( 'NONE',  ( 17.18269478283314911, 17.18269478283310647, -64.92279855667830191 ) ) ;
#189600=CARTESIAN_POINT ( 'NONE',  ( 28.90000000000003411, -0.1280799071098031872, -52.65483682830183199 ) ) ;
#189603=CARTESIAN_POINT ( 'NONE',  ( -17.18269478283327345, -17.18269478283298568, -56.77278709839600879 ) ) ;
#189631=ORIENTED_EDGE ( 'NONE', *, *, #167871, .F. ) ;
#189654=EDGE_CURVE ( 'NONE', #70174, #91244, #44272, .T. ) ;
#189711=CARTESIAN_POINT ( 'NONE',  ( -19.99999999999998224, -188.0000000000000000, 0.000000000000000000 ) ) ;
#189731=DIRECTION ( 'NONE',  ( -0.000000000000000000, -0.000000000000000000, 1.000000000000000000 ) ) ;
#189737=CARTESIAN_POINT ( 'NONE',  ( -6.586805632895485375E-13, -76.33425854457905757, -24.99989890116611946 ) ) ;
#189749=FACE_OUTER_BOUND ( 'NONE', #182679, .T. ) ;
#189753=CARTESIAN_POINT ( 'NONE',  ( 36.91746824999999887, 11.99521256947799053, -10.02499999726881086 ) ) ;
#189801=CARTESIAN_POINT ( 'NONE',  ( 36.91746825000000598, -11.99521256947793546, -6.224999997268814589 ) ) ;
#189816=VERTEX_POINT ( 'NONE', #196971 ) ;
#189824=ORIENTED_EDGE ( 'NONE', *, *, #187510, .F. ) ;
#189848=DIRECTION ( 'NONE',  ( 0.000000000000000000, 0.000000000000000000, 1.000000000000000000 ) ) ;
#189888=DIRECTION ( 'NONE',  ( 1.000000000000000000, -3.552713678800500929E-15, 0.000000000000000000 ) ) ;
#189942=DIRECTION ( 'NONE',  ( -1.000000000000000000, 0.000000000000000000, 0.000000000000000000 ) ) ;
#189946=DIRECTION ( 'NONE',  ( -0.000000000000000000, -0.000000000000000000, 1.000000000000000000 ) ) ;
#189969=CARTESIAN_POINT ( 'NONE',  ( -3.573655867282028392E-15, -180.0000000000000000, -25.00000000000000000 ) ) ;
#189977=ORIENTED_EDGE ( 'NONE', *, *, #167871, .T. ) ;
#189980=CARTESIAN_POINT ( 'NONE',  ( 9.100000000000001421, -3.435030038190235346E-14, -64.92279855667830191 ) ) ;
#189994=DIRECTION ( 'NONE',  ( 1.000000000000000000, 0.000000000000000000, 0.000000000000000000 ) ) ;
#189997=CARTESIAN_POINT ( 'NONE',  ( 28.61453998622355144, -24.72048905145110709, -21.14736193440035095 ) ) ;
#190000=ADVANCED_FACE ( 'NONE', ( #104944 ), #158396, .T. ) ;
#190010=CARTESIAN_POINT ( 'NONE',  ( -19.99604614807107694, -21.41307096498895390, -49.20022480689105038 ) ) ;
#190041=CARTESIAN_POINT ( 'NONE',  ( -1.503321482105500984, -30.27664185797782537, -47.91583118997741764 ) ) ;
#190046=DIRECTION ( 'NONE',  ( 0.9974398506828145994, -0.07151044867601324961, 1.161577285759629397E-15 ) ) ;
#190123=ADVANCED_FACE ( 'NONE', ( #64404 ), #126073, .T. ) ;
#190175=CIRCLE ( 'NONE', #103009, 6.100000000000006750 ) ;
#190209=CARTESIAN_POINT ( 'NONE',  ( 15.01118352434402858, -1.500065973499219218, -62.04667436142315040 ) ) ;
#190234=EDGE_CURVE ( 'NONE', #40506, #166185, #172582, .T. ) ;
#190237=DIRECTION ( 'NONE',  ( 1.000000000000000000, 0.000000000000000000, 0.000000000000000000 ) ) ;
#190250=ORIENTED_EDGE ( 'NONE', *, *, #121940, .T. ) ;
#190274=CARTESIAN_POINT ( 'NONE',  ( -11.74264578624800670, 36.14014761921585972, -10.14999999453762669 ) ) ;
#190277=CARTESIAN_POINT ( 'NONE',  ( 33.23029939923979725, -20.96646023091231470, -17.75854212242024843 ) ) ;
#190280=ORIENTED_EDGE ( 'NONE', *, *, #18014, .T. ) ;
#190338=AXIS2_PLACEMENT_3D ( 'NONE', #158826, #123507, #5138 ) ;
#190354=CARTESIAN_POINT ( 'NONE',  ( -6.856101608890801443E-16, -64.86648100006283357, -22.99999901186701123 ) ) ;
#190385=FACE_OUTER_BOUND ( 'NONE', #36490, .T. ) ;
#190390=CARTESIAN_POINT ( 'NONE',  ( -29.40414617605185654, -24.07794639774997236, -17.69092940303636396 ) ) ;
#190392=CARTESIAN_POINT ( 'NONE',  ( -20.06002596795686443, -21.05152699199194899, -52.46707657590843610 ) ) ;
#190444=CARTESIAN_POINT ( 'NONE',  ( -35.57212018828867883, -18.96864681237437722, -18.54270186059685344 ) ) ;
#190468=CARTESIAN_POINT ( 'NONE',  ( -31.61347055016709007, 0.9086318102908346184, -46.06737158113915598 ) ) ;
#190472=CARTESIAN_POINT ( 'NONE',  ( 3.766062262543149401E-15, -39.95556452105413570, -7.249999994537627224 ) ) ;
#190475=DIRECTION ( 'NONE',  ( 1.000000000000000000, 0.000000000000000000, 0.000000000000000000 ) ) ;
#190547=ADVANCED_FACE ( 'NONE', ( #189749 ), #18907, .F. ) ;
#190550=VERTEX_POINT ( 'NONE', #78563 ) ;
#190551=CARTESIAN_POINT ( 'NONE',  ( -37.45873412500000654, 2.428612866367529932E-14, -10.31249999863440792 ) ) ;
#190554=CARTESIAN_POINT ( 'NONE',  ( -11.40812507854754720, -35.11059874428192273, -8.724999997268813701 ) ) ;
#190587=CARTESIAN_POINT ( 'NONE',  ( 5.000000000000003553, -4.999999999999996447, -18.00000000000000000 ) ) ;
#190686=ORIENTED_EDGE ( 'NONE', *, *, #164374, .F. ) ;
#190710=CARTESIAN_POINT ( 'NONE',  ( 0.000000000000000000, 0.000000000000000000, -32.60000000000000142 ) ) ;
#190715=CARTESIAN_POINT ( 'NONE',  ( -23.36741966814226146, -32.36690354120219837, -22.32433735814168330 ) ) ;
#190734=VERTEX_POINT ( 'NONE', #7694 ) ;
#190786=CARTESIAN_POINT ( 'NONE',  ( 29.86685920354754487, 21.69954338932564752, -5.924999997268813878 ) ) ;
#190787=CARTESIAN_POINT ( 'NONE',  ( -22.99870628207715484, 21.53952979013931213, -49.63989001790915268 ) ) ;
#190801=ORIENTED_EDGE ( 'NONE', *, *, #93266, .T. ) ;
#190867=ADVANCED_FACE ( 'NONE', ( #55211 ), #70386, .F. ) ;
#190871=DIRECTION ( 'NONE',  ( -0.000000000000000000, -0.000000000000000000, 1.000000000000000000 ) ) ;
#190912=CARTESIAN_POINT ( 'NONE',  ( 19.97888994334924107, -34.65319547504298470, -5.000000000000000000 ) ) ;
#190930=CARTESIAN_POINT ( 'NONE',  ( -7.005188342139613944, -46.65430082754587460, -22.59844067006689272 ) ) ;
#190952=CARTESIAN_POINT ( 'NONE',  ( -31.78116016545939715, 0.5954834035870623099, -49.28208245900471240 ) ) ;
#190965=VERTEX_POINT ( 'NONE', #178572 ) ;
#190968=DIRECTION ( 'NONE',  ( -0.000000000000000000, -0.000000000000000000, 1.000000000000000000 ) ) ;
#190971=CARTESIAN_POINT ( 'NONE',  ( -6.020228577223754586E-15, 39.95556452105416412, -2.249999994537625891 ) ) ;
#190982=FACE_OUTER_BOUND ( 'NONE', #720, .T. ) ;
#190986=CARTESIAN_POINT ( 'NONE',  ( -2.500000000000000000, -105.0000000000000000, 12.00000000000000355 ) ) ;
#191015=EDGE_CURVE ( 'NONE', #140310, #29006, #14062, .T. ) ;
#191042=CARTESIAN_POINT ( 'NONE',  ( -13.59403193627398387, -42.61206874334182970, -22.32444481402297498 ) ) ;
#191043=ORIENTED_EDGE ( 'NONE', *, *, #23592, .F. ) ;
#191055=ORIENTED_EDGE ( 'NONE', *, *, #145315, .T. ) ;
#191066=CARTESIAN_POINT ( 'NONE',  ( -38.00000000000000711, 2.428612866367529932E-14, -9.749999994537626336 ) ) ;
#191077=CARTESIAN_POINT ( 'NONE',  ( -0.7627558185761093013, -6.293264767923594682, -62.46802126132829613 ) ) ;
#191101=CARTESIAN_POINT ( 'NONE',  ( -8.969129508634374304, -36.34711360786828749, -31.52745775292092034 ) ) ;
#191111=DIRECTION ( 'NONE',  ( -0.000000000000000000, -0.000000000000000000, 1.000000000000000000 ) ) ;
#191135=EDGE_CURVE ( 'NONE', #126569, #64219, #174863, .T. ) ;
#191176=CARTESIAN_POINT ( 'NONE',  ( -14.62203461105352886, -16.42370670853598824, -58.41511589169243024 ) ) ;
#191197=DIRECTION ( 'NONE',  ( 1.000000000000000000, 0.000000000000000000, 0.000000000000000000 ) ) ;
#191225=FACE_OUTER_BOUND ( 'NONE', #111891, .T. ) ;
#191266=CARTESIAN_POINT ( 'NONE',  ( -38.00000000000000711, 12.34694845685046438, -9.849999994537625980 ) ) ;
#191269=CARTESIAN_POINT ( 'NONE',  ( 26.89045226410947720, -26.45365283845879745, -20.38637362917750551 ) ) ;
#191292=CARTESIAN_POINT ( 'NONE',  ( -17.18269478283327345, -17.18269478283298568, -64.92279855667830191 ) ) ;
#191296=ORIENTED_EDGE ( 'NONE', *, *, #197529, .T. ) ;
#191328=ADVANCED_FACE ( 'NONE', ( #127703 ), #141880, .T. ) ;
#191407=( BOUNDED_CURVE ( )  B_SPLINE_CURVE ( 2, ( #100409, #191423, #72080, #39737, #6393, #86244, #162090, #68072, #195448, #85233, #133754 ),
 .UNSPECIFIED., .F., .T. ) 
 B_SPLINE_CURVE_WITH_KNOTS ( ( 3, 2, 2, 2, 2, 3 ),
 ( 0.3000000000000000444, 0.3200000000000000622, 0.3400000000000000799, 0.3599999999999999867, 0.3800000000000000044, 0.4000000000000000222 ),
 .UNSPECIFIED. ) 
 CURVE ( )  GEOMETRIC_REPRESENTATION_ITEM ( )  RATIONAL_B_SPLINE_CURVE ( ( 0.9999999999999998890, 0.9510565162951536422, 1.000000000000000000, 0.9510565162951535312, 1.000000000000000000, 0.9510565162951535312, 1.000000000000000000, 0.9510565162951535312, 1.000000000000000000, 0.9510565162951535312, 1.000000000000000000 ) ) 
 REPRESENTATION_ITEM ( '' )  );
#191422=ORIENTED_EDGE ( 'NONE', *, *, #55329, .F. ) ;
#191423=CARTESIAN_POINT ( 'NONE',  ( 37.99999999999998579, -12.34694845685043951, -3.100000000000000977 ) ) ;
#191431=CARTESIAN_POINT ( 'NONE',  ( -9.553523354579670723, -9.835363051420090486, -62.57666384180342334 ) ) ;
#191474=VERTEX_POINT ( 'NONE', #160043 ) ;
#191477=CARTESIAN_POINT ( 'NONE',  ( -29.86685920354755197, -21.69954338932560134, -10.42499999726881299 ) ) ;
#191505=DIRECTION ( 'NONE',  ( -0.000000000000000000, 0.000000000000000000, -1.000000000000000000 ) ) ;
#191541=CARTESIAN_POINT ( 'NONE',  ( -36.91746825000000598, 2.428612866367529932E-14, -9.124999997268814056 ) ) ;
#191573=EDGE_CURVE ( 'NONE', #124248, #145335, #178101, .T. ) ;
#191579=CYLINDRICAL_SURFACE ( 'NONE', #70961, 61.99999999999998579 ) ;
#191645=VECTOR ( 'NONE', #141485, 1000.000000000000000 ) ;
#191674=ORIENTED_EDGE ( 'NONE', *, *, #35293, .F. ) ;
#191687=CARTESIAN_POINT ( 'NONE',  ( 20.08580022215228666, 20.97218796591011625, -49.51012018364364309 ) ) ;
#191702=LINE ( 'NONE', #23866, #180822 ) ;
#191709=ORIENTED_EDGE ( 'NONE', *, *, #145315, .F. ) ;
#191711=CARTESIAN_POINT ( 'NONE',  ( 1.508955259217861487E-14, -71.74905152827281540, -24.99410988490251029 ) ) ;
#191713=CARTESIAN_POINT ( 'NONE',  ( 29.86685920354754487, 21.69954338932564752, -1.424999997268813212 ) ) ;
#191720=ORIENTED_EDGE ( 'NONE', *, *, #125126, .F. ) ;
#191722=AXIS2_PLACEMENT_3D ( 'NONE', #104055, #120209, #133388 ) ;
#191742=EDGE_CURVE ( 'NONE', #119352, #76158, #152812, .T. ) ;
#191792=ORIENTED_EDGE ( 'NONE', *, *, #148801, .T. ) ;
#191943=LINE ( 'NONE', #175788, #37849 ) ;
#191950=VECTOR ( 'NONE', #136374, 1000.000000000000000 ) ;
#191957=ORIENTED_EDGE ( 'NONE', *, *, #44038, .T. ) ;
#191971=LINE ( 'NONE', #172078, #24260 ) ;
#191974=LINE ( 'NONE', #145462, #167160 ) ;
#191996=DIRECTION ( 'NONE',  ( 1.000000000000000000, 0.000000000000000000, 0.000000000000000000 ) ) ;
#192007=CIRCLE ( 'NONE', #133869, 28.90000000000004476 ) ;
#192022=DIRECTION ( 'NONE',  ( 0.000000000000000000, 0.000000000000000000, 1.000000000000000000 ) ) ;
#192029=DIRECTION ( 'NONE',  ( -0.000000000000000000, -0.000000000000000000, 1.000000000000000000 ) ) ;
#192030=ORIENTED_EDGE ( 'NONE', *, *, #143190, .T. ) ;
#192036=CARTESIAN_POINT ( 'NONE',  ( -18.37518290867432214, -35.61898371400481267, -22.28534798804468053 ) ) ;
#192064=DIRECTION ( 'NONE',  ( -0.000000000000000000, -0.000000000000000000, -1.000000000000000000 ) ) ;
#192121=EDGE_CURVE ( 'NONE', #22413, #178146, #133496, .T. ) ;
#192143=CONICAL_SURFACE ( 'NONE', #153458, 2.500000000000000000, 1.029744258676656976 ) ;
#192175=CARTESIAN_POINT ( 'NONE',  ( -16.17338109997596973, -17.62895962574413389, -57.05728224822367878 ) ) ;
#192219=TOROIDAL_SURFACE ( 'NONE', #53348, 69.99999999999998579, 8.000000000000000000 ) ;
#192226=AXIS2_PLACEMENT_3D ( 'NONE', #125573, #154913, #79059 ) ;
#192227=CYLINDRICAL_SURFACE ( 'NONE', #112651, 1.499999999999997780 ) ;
#192238=DIRECTION ( 'NONE',  ( 1.000000000000000000, 0.000000000000000000, 0.000000000000000000 ) ) ;
#192252=ORIENTED_EDGE ( 'NONE', *, *, #195257, .T. ) ;
#192278=CARTESIAN_POINT ( 'NONE',  ( 28.83006054357690573, -24.83490584245822674, -16.72457388842970261 ) ) ;
#192282=ORIENTED_EDGE ( 'NONE', *, *, #58626, .T. ) ;
#192285=B_SPLINE_CURVE_WITH_KNOTS ( 'NONE', 3,
 ( #17377, #168075, #29572, #14389, #60879, #184246, #45728, #169052, #50706, #156888, #81020, #65853, #3195, #190209, #126530, #34534, #159862, #37517, #80035, #173057, #64868, #97172 ),
 .UNSPECIFIED., .F., .F.,
 ( 4, 2, 2, 2, 2, 2, 2, 2, 2, 2, 4 ),
 ( 1.970604704475788300E-07, 0.0003054521314109980793, 0.0006107072023515486498, 0.001221217344232650116, 0.001831727486113751691, 0.002136982557054302369, 0.002442237627994853482, 0.003052747769875962646, 0.003663257911757071810, 0.004273768053638180540, 0.004884278195519286235 ),
 .UNSPECIFIED. ) ;
#192307=ORIENTED_EDGE ( 'NONE', *, *, #170515, .T. ) ;
#192338=FACE_OUTER_BOUND ( 'NONE', #84516, .T. ) ;
#192341=ORIENTED_EDGE ( 'NONE', *, *, #152270, .T. ) ;
#192347=FACE_OUTER_BOUND ( 'NONE', #75058, .T. ) ;
#192388=DIRECTION ( 'NONE',  ( 0.9930308165857338887, -0.1178549842436482226, 0.000000000000000000 ) ) ;
#192437=AXIS2_PLACEMENT_3D ( 'NONE', #167149, #43800, #151968 ) ;
#192465=CARTESIAN_POINT ( 'NONE',  ( -30.11448378070091891, 1.481880339025834381, -48.12989299794421072 ) ) ;
#192484=EDGE_CURVE ( 'NONE', #123757, #84237, #97940, .T. ) ;
#192491=CARTESIAN_POINT ( 'NONE',  ( -11.40812507854754720, -35.11059874428192273, -8.224999997268813701 ) ) ;
#192513=ORIENTED_EDGE ( 'NONE', *, *, #31579, .F. ) ;
#192547=ORIENTED_EDGE ( 'NONE', *, *, #197529, .F. ) ;
#192549=LINE ( 'NONE', #25715, #22784 ) ;
#192552=CARTESIAN_POINT ( 'NONE',  ( -36.91746825000001309, 11.99521256947798342, -8.724999997268813701 ) ) ;
#192588=CARTESIAN_POINT ( 'NONE',  ( 29.18776880969887699, -0.8894290736107985929, -52.33677266386643367 ) ) ;
#192619=ORIENTED_EDGE ( 'NONE', *, *, #25423, .T. ) ;
#192660=EDGE_CURVE ( 'NONE', #5010, #196218, #182042, .T. ) ;
#192699=CARTESIAN_POINT ( 'NONE',  ( 22.35296335725861994, 22.73357338108561265, -45.67722784712128714 ) ) ;
#192723=LINE ( 'NONE', #51210, #117886 ) ;
#192725=CARTESIAN_POINT ( 'NONE',  ( -36.91746825000000598, 11.99521256947798520, -0.7249999972688133676 ) ) ;
#192734=VERTEX_POINT ( 'NONE', #92980 ) ;
#192810=ORIENTED_EDGE ( 'NONE', *, *, #55941, .F. ) ;
#192837=VECTOR ( 'NONE', #150437, 1000.000000000000000 ) ;
#192859=ORIENTED_EDGE ( 'NONE', *, *, #48777, .T. ) ;
#192956=CARTESIAN_POINT ( 'NONE',  ( 17.24269848851061226, -15.08844724069277454, -55.31736789360020623 ) ) ;
#192965=EDGE_CURVE ( 'NONE', #45827, #9769, #9059, .T. ) ;
#192969=ORIENTED_EDGE ( 'NONE', *, *, #160152, .F. ) ;
#192972=CYLINDRICAL_SURFACE ( 'NONE', #140706, 21.30000000000002913 ) ;
#192975=CARTESIAN_POINT ( 'NONE',  ( -38.00000000000000711, 2.428612866367529932E-14, -7.749999994537626336 ) ) ;
#192980=EDGE_CURVE ( 'NONE', #156405, #181594, #60655, .T. ) ;
#192989=FACE_OUTER_BOUND ( 'NONE', #116412, .T. ) ;
#192993=CIRCLE ( 'NONE', #105812, 13.70000000000001528 ) ;
#193025=CARTESIAN_POINT ( 'NONE',  ( 11.40812507854754365, 35.11059874428196537, -5.724999997268812812 ) ) ;
#193026=CARTESIAN_POINT ( 'NONE',  ( 0.000000000000000000, 0.000000000000000000, -56.77278709839600879 ) ) ;
#193035=LINE ( 'NONE', #133347, #162948 ) ;
#193048=CARTESIAN_POINT ( 'NONE',  ( -7.905529020988549149, -46.70198807553910569, -24.42054064165492733 ) ) ;
#193058=CARTESIAN_POINT ( 'NONE',  ( 9.621741624713976648, 11.74323870453916996, -62.00714677346290671 ) ) ;
#193063=CARTESIAN_POINT ( 'NONE',  ( 23.15940025311444472, -1.498759781556224580, -55.09305739490147857 ) ) ;
#193200=CARTESIAN_POINT ( 'NONE',  ( 8.636255518949004895, -38.40306468563544229, -32.12764100183819949 ) ) ;
#193229=FACE_OUTER_BOUND ( 'NONE', #8010, .T. ) ;
#193246=CARTESIAN_POINT ( 'NONE',  ( -16.61636759701969979, 0.5040881997805581882, -59.17093420172795248 ) ) ;
#193266=ORIENTED_EDGE ( 'NONE', *, *, #94659, .T. ) ;
#193305=EDGE_CURVE ( 'NONE', #102181, #27924, #175808, .T. ) ;
#193343=VERTEX_POINT ( 'NONE', #96950 ) ;
#193431=EDGE_LOOP ( 'NONE', ( #87156, #68908, #72384, #109791 ) ) ;
#193437=DIRECTION ( 'NONE',  ( 1.000000000000000000, 0.000000000000000000, 0.000000000000000000 ) ) ;
#193458=DIRECTION ( 'NONE',  ( 1.000000000000000000, 0.000000000000000000, 0.000000000000000000 ) ) ;
#193461=VERTEX_POINT ( 'NONE', #22120 ) ;
#193471=CARTESIAN_POINT ( 'NONE',  ( 4.884805615686635960, 6.795352961392285174, -64.11485260110077888 ) ) ;
#193472=CARTESIAN_POINT ( 'NONE',  ( 11.74264578624800315, -36.14014761921581709, -7.149999994537626691 ) ) ;
#193474=CARTESIAN_POINT ( 'NONE',  ( 16.68934465457933669, -0.2055526423334347597, -59.13845350790284527 ) ) ;
#193484=DIRECTION ( 'NONE',  ( 1.000000000000000000, 0.000000000000000000, 0.000000000000000000 ) ) ;
#193492=CARTESIAN_POINT ( 'NONE',  ( -38.00000000000001421, -12.34694845685042708, -1.899999999999999911 ) ) ;
#193498=CARTESIAN_POINT ( 'NONE',  ( 1.500000000000122347, 15.29436794386904097, -59.75403449828548474 ) ) ;
#193502=CARTESIAN_POINT ( 'NONE',  ( 28.71047547314890025, -27.16362253576316377, -18.60589795199476271 ) ) ;
#193552=ORIENTED_EDGE ( 'NONE', *, *, #165816, .F. ) ;
#193557=CARTESIAN_POINT ( 'NONE',  ( 11.40812507854755253, -35.11059874428192273, -8.024999997268814411 ) ) ;
#193562=DIRECTION ( 'NONE',  ( -1.000000000000000000, 0.000000000000000000, 0.000000000000000000 ) ) ;
#193594=CARTESIAN_POINT ( 'NONE',  ( -193.3062444957834884, -155.7167183371838064, 0.000000000000000000 ) ) ;
#193642=ADVANCED_FACE ( 'NONE', ( #126310 ), #90994, .F. ) ;
#193677=VERTEX_POINT ( 'NONE', #126076 ) ;
#193684=EDGE_CURVE ( 'NONE', #66459, #52978, #33456, .T. ) ;
#193707=ORIENTED_EDGE ( 'NONE', *, *, #37197, .T. ) ;
#193723=CARTESIAN_POINT ( 'NONE',  ( -31.65755289763026781, -24.31906878930451654, -22.32084141216703088 ) ) ;
#193734=CARTESIAN_POINT ( 'NONE',  ( 11.40812507854754365, 35.11059874428196537, -1.224999997268813479 ) ) ;
#193745=DIRECTION ( 'NONE',  ( 1.000000000000000000, 3.552713678800500929E-15, 0.000000000000000000 ) ) ;
#193785=LINE ( 'NONE', #25944, #17856 ) ;
#193869=CARTESIAN_POINT ( 'NONE',  ( -8.388830574159379737E-16, -13.70000000000001528, -64.92279855667830191 ) ) ;
#193896=EDGE_CURVE ( 'NONE', #91244, #157973, #6510, .T. ) ;
#193906=CARTESIAN_POINT ( 'NONE',  ( -23.48529157249600985, 32.32473071737754111, -2.049999994537626158 ) ) ;
#193924=CARTESIAN_POINT ( 'NONE',  ( -15.51017872335181558, 14.74842737557647787, -56.39952970130666898 ) ) ;
#193942=CARTESIAN_POINT ( 'NONE',  ( -5.630366384182114103, -47.63986359793420888, -22.87684677290789637 ) ) ;
#193948=CARTESIAN_POINT ( 'NONE',  ( -1.428615351859108040, -15.66706267174403422, -61.77652290643389676 ) ) ;
#193982=CARTESIAN_POINT ( 'NONE',  ( -69.65682714487590488, -71.74905178543390605, -23.00000000000000000 ) ) ;
#193986=CARTESIAN_POINT ( 'NONE',  ( 37.99999999999999289, 2.893978650043524126E-14, -8.749999994537628112 ) ) ;
#193993=CARTESIAN_POINT ( 'NONE',  ( 6.852329227654482047, -5.080395570733999833, -62.03049426788788878 ) ) ;
#193999=CARTESIAN_POINT ( 'NONE',  ( -12.05038478428680371, 9.979736640218501265, -59.62998087139816761 ) ) ;
#194037=CARTESIAN_POINT ( 'NONE',  ( -29.86685920354755197, -21.69954338932560134, -6.924999997268813878 ) ) ;
#194038=CARTESIAN_POINT ( 'NONE',  ( -0.5310992180246781880, -24.20670376297026749, -56.83968087238905298 ) ) ;
#194047=CARTESIAN_POINT ( 'NONE',  ( 0.000000000000000000, 0.000000000000000000, -18.00000000000000000 ) ) ;
#194061=CARTESIAN_POINT ( 'NONE',  ( -25.90378602754346815, -30.37248848106881027, -17.06839622125142952 ) ) ;
#194072=CARTESIAN_POINT ( 'NONE',  ( 10.33258783678506987, 12.20200080651908792, -61.66593582935062301 ) ) ;
#194076=CARTESIAN_POINT ( 'NONE',  ( 24.30000000000003268, 0.000000000000000000, -54.21489346206828230 ) ) ;
#194088=CARTESIAN_POINT ( 'NONE',  ( 1.216837300817233514, 16.09857462465207334, -61.59776990020974097 ) ) ;
#194187=CARTESIAN_POINT ( 'NONE',  ( -23.48529157249600985, 32.32473071737754111, -6.299999999999999822 ) ) ;
#194207=VERTEX_POINT ( 'NONE', #105598 ) ;
#194210=CARTESIAN_POINT ( 'NONE',  ( 15.38714178908743690, -36.74766143018467801, -28.97229394964844928 ) ) ;
#194240=CARTESIAN_POINT ( 'NONE',  ( -9.887582997646811478, -11.98499751262841073, -59.67881039541425281 ) ) ;
#194247=CARTESIAN_POINT ( 'NONE',  ( 0.000000000000000000, 0.000000000000000000, -62.58071313852362039 ) ) ;
#194281=EDGE_CURVE ( 'NONE', #44348, #73091, #3996, .T. ) ;
#194285=DIRECTION ( 'NONE',  ( 3.469446951953612217E-15, 0.000000000000000000, -1.000000000000000000 ) ) ;
#194310=EDGE_CURVE ( 'NONE', #178697, #44348, #170549, .T. ) ;
#194438=ORIENTED_EDGE ( 'NONE', *, *, #58231, .T. ) ;
#194447=CARTESIAN_POINT ( 'NONE',  ( -9.616242481452241364, -9.758483323059184755, -62.58071313852360618 ) ) ;
#194465=DIRECTION ( 'NONE',  ( -1.000000000000000000, 0.000000000000000000, 0.000000000000000000 ) ) ;
#194467=CARTESIAN_POINT ( 'NONE',  ( 1.461575671818346356, 7.989192496695419976, -62.12244103964774666 ) ) ;
#194471=CARTESIAN_POINT ( 'NONE',  ( -3.573655867282028392E-15, 2.428612866367529932E-14, -15.00000000000000000 ) ) ;
#194492=VERTEX_POINT ( 'NONE', #98346 ) ;
#194495=CARTESIAN_POINT ( 'NONE',  ( -36.91746825000000598, 2.428612866367529932E-14, -8.624999997268814056 ) ) ;
#194521=CARTESIAN_POINT ( 'NONE',  ( 2.802625768539491524, -39.09149893265185227, -22.99999999999999289 ) ) ;
#194525=VERTEX_POINT ( 'NONE', #34712 ) ;
#194532=CARTESIAN_POINT ( 'NONE',  ( -24.78074900657737345, -31.51706519598950607, -17.29086010071288726 ) ) ;
#194548=EDGE_CURVE ( 'NONE', #11425, #192734, #69101, .T. ) ;
#194556=CARTESIAN_POINT ( 'NONE',  ( -5.950531402560715689E-15, 38.81732327939063509, -9.124999997268815832 ) ) ;
#194618=ORIENTED_EDGE ( 'NONE', *, *, #193305, .F. ) ;
#194649=VECTOR ( 'NONE', #42654, 1000.000000000000000 ) ;
#194707=CARTESIAN_POINT ( 'NONE',  ( 1.304248841091933035E-15, 21.30000000000002913, -56.46919128290398504 ) ) ;
#194716=CARTESIAN_POINT ( 'NONE',  ( -14.98799772565112498, -15.13475115289583961, -56.46919128290397794 ) ) ;
#194721=CARTESIAN_POINT ( 'NONE',  ( -20.41037832431298682, -34.40082058117823749, -25.00000000000009592 ) ) ;
#194765=EDGE_LOOP ( 'NONE', ( #53086, #162089, #98581, #151019, #167942 ) ) ;
#194805=EDGE_LOOP ( 'NONE', ( #33952, #21202, #21190, #26706, #107277 ) ) ;
#194812=ADVANCED_FACE ( 'NONE', ( #110553 ), #141882, .T. ) ;
#194848=AXIS2_PLACEMENT_3D ( 'NONE', #95727, #33076, #141237 ) ;
#194861=ORIENTED_EDGE ( 'NONE', *, *, #187746, .T. ) ;
#194879=DIRECTION ( 'NONE',  ( 1.000000000000000000, 0.000000000000000000, 0.000000000000000000 ) ) ;
#194935=CARTESIAN_POINT ( 'NONE',  ( -17.93416671128591489, -36.08982269496700468, -18.53391066944203303 ) ) ;
#194941=CARTESIAN_POINT ( 'NONE',  ( -1.216645939406758359, -16.09882439466101189, -61.59766612755958448 ) ) ;
#194961=CARTESIAN_POINT ( 'NONE',  ( 12.08085585438963605, -10.04536149086137264, -59.60010879982917231 ) ) ;
#194976=CARTESIAN_POINT ( 'NONE',  ( 30.74264578624799782, 22.33583958711400541, -8.549999994537627046 ) ) ;
#195028=CARTESIAN_POINT ( 'NONE',  ( 29.86685920354754487, 21.69954338932564752, -3.924999997268812990 ) ) ;
#195029=CARTESIAN_POINT ( 'NONE',  ( -0.9720251121415244278, -23.94686256013569192, -57.02522261278124205 ) ) ;
#195050=CARTESIAN_POINT ( 'NONE',  ( -25.79201298824010991, -30.25621121864696050, -20.58051720724199996 ) ) ;
#195052=ORIENTED_EDGE ( 'NONE', *, *, #192980, .T. ) ;
#195061=CARTESIAN_POINT ( 'NONE',  ( 11.80868324581537543, 11.80868324581533990, -61.34707691135562868 ) ) ;
#195065=CARTESIAN_POINT ( 'NONE',  ( -1.500047742438159526, -7.503727747132431958, -64.26135111332261829 ) ) ;
#195183=CARTESIAN_POINT ( 'NONE',  ( -4.713873842512037449, 4.023452810412264213, -62.49134662286012087 ) ) ;
#195186=CARTESIAN_POINT ( 'NONE',  ( -30.51643230682433838, -22.56685799121283509, -22.94790682118908620 ) ) ;
#195188=EDGE_CURVE ( 'NONE', #142912, #53136, #4420, .T. ) ;
#195208=DIRECTION ( 'NONE',  ( -0.000000000000000000, -0.000000000000000000, 1.000000000000000000 ) ) ;
#195236=CARTESIAN_POINT ( 'NONE',  ( -38.00000000000000711, 12.34694845685046438, -4.100000000000000533 ) ) ;
#195249=CARTESIAN_POINT ( 'NONE',  ( 1.304248841091933035E-15, 21.30000000000002913, -65.00100000000003320 ) ) ;
#195253=CARTESIAN_POINT ( 'NONE',  ( 11.55487914182273457, -42.80721638308649801, -21.19679778042605278 ) ) ;
#195257=EDGE_CURVE ( 'NONE', #141549, #137721, #43192, .T. ) ;
#195352=CARTESIAN_POINT ( 'NONE',  ( 1.135581650430530276, 6.614994358112536332, -64.43300989196958994 ) ) ;
#195370=EDGE_CURVE ( 'NONE', #171664, #119464, #134408, .T. ) ;
#195377=CIRCLE ( 'NONE', #40350, 2.500000000000000000 ) ;
#195390=CARTESIAN_POINT ( 'NONE',  ( -38.00000000000000711, -12.34694845685042708, -3.649999994537626691 ) ) ;
#195421=AXIS2_PLACEMENT_3D ( 'NONE', #150966, #136761, #41790 ) ;
#195448=CARTESIAN_POINT ( 'NONE',  ( -30.74264578624800492, -22.33583958711396278, -3.799999999999999822 ) ) ;
#195458=CARTESIAN_POINT ( 'NONE',  ( 1.223485768069169977, 29.52714030619467422, -51.95675375490479553 ) ) ;
#195501=EDGE_CURVE ( 'NONE', #145210, #152430, #152953, .T. ) ;
#195505=CARTESIAN_POINT ( 'NONE',  ( 36.91746825000000598, -11.99521256947793546, -9.724999997268813701 ) ) ;
#195535=ORIENTED_EDGE ( 'NONE', *, *, #85538, .T. ) ;
#195550=CIRCLE ( 'NONE', #24368, 9.100000000000001421 ) ;
#195560=ORIENTED_EDGE ( 'NONE', *, *, #749, .T. ) ;
#195565=CARTESIAN_POINT ( 'NONE',  ( -29.86685920354755197, -21.69954338932560134, -4.424999997268812990 ) ) ;
#195610=EDGE_CURVE ( 'NONE', #150779, #190965, #125819, .T. ) ;
#195638=ORIENTED_EDGE ( 'NONE', *, *, #197184, .T. ) ;
#195656=EDGE_CURVE ( 'NONE', #85313, #515, #85111, .T. ) ;
#195701=EDGE_CURVE ( 'NONE', #93860, #194492, #32826, .T. ) ;
#195719=CARTESIAN_POINT ( 'NONE',  ( -8.343164238912773811, -45.63112023308526233, -22.26988597240830003 ) ) ;
#195734=DIRECTION ( 'NONE',  ( 0.000000000000000000, 0.000000000000000000, 1.000000000000000000 ) ) ;
#195743=CARTESIAN_POINT ( 'NONE',  ( -32.86500790357915491, -22.80501606679668924, -22.13190935960392025 ) ) ;
#195771=B_SPLINE_CURVE_WITH_KNOTS ( 'NONE', 3,
 ( #48268, #198964, #123096, #45282, #78580, #124085, #106935, #110912, #93756, #14941, #742, #107923, #76601, #2742, #60431, #122105, #183795, #62414, #109922, #30108, #16927, #92754, #155437, #64419, #168608, #34084 ),
 .UNSPECIFIED., .F., .F.,
 ( 4, 2, 2, 2, 2, 2, 2, 2, 2, 2, 2, 2, 4 ),
 ( 2.788259459799404871E-07, 0.0002964138711649459907, 0.0005925489163839111695, 0.0008886839616028763484, 0.001184819006821841419, 0.001777089097259771776, 0.002369359187697702568, 0.002665494232916669048, 0.002961629278135635094, 0.003257764323354601574, 0.003553899368573567186, 0.004146169459011494508, 0.004738439549449421397 ),
 .UNSPECIFIED. ) ;
#195888=AXIS2_PLACEMENT_3D ( 'NONE', #10187, #195208, #7160 ) ;
#195971=CARTESIAN_POINT ( 'NONE',  ( 1.499999999999985789, 30.40000000000003766, -65.00100000000003320 ) ) ;
#195982=EDGE_LOOP ( 'NONE', ( #13857, #153311, #67166, #88345, #2238 ) ) ;
#195991=CARTESIAN_POINT ( 'NONE',  ( -6.020228577223754586E-15, 39.95556452105416412, -10.24999999453762456 ) ) ;
#196003=DIRECTION ( 'NONE',  ( -1.000000000000000000, -0.000000000000000000, -1.908195823574487804E-15 ) ) ;
#196022=CIRCLE ( 'NONE', #60318, 24.30000000000003268 ) ;
#196040=CARTESIAN_POINT ( 'NONE',  ( 3.556970738554034288E-15, -38.81732327939057114, -6.624999997268814056 ) ) ;
#196041=CARTESIAN_POINT ( 'NONE',  ( -0.2211803504528828124, -21.31248648291599324, -58.84879416108401529 ) ) ;
#196057=EDGE_LOOP ( 'NONE', ( #81653, #41041, #64339, #194618 ) ) ;
#196063=CARTESIAN_POINT ( 'NONE',  ( -23.74378949184693965, -32.05510596162310577, -22.01707947879407357 ) ) ;
#196064=ORIENTED_EDGE ( 'NONE', *, *, #11729, .F. ) ;
#196079=CARTESIAN_POINT ( 'NONE',  ( -0.1983487321476344600, -9.090093023806476324, -63.95305636720455311 ) ) ;
#196092=LINE ( 'NONE', #57562, #85641 ) ;
#196131=CARTESIAN_POINT ( 'NONE',  ( -19.24578484527059175, -180.9428398739491684, 0.000000000000000000 ) ) ;
#196203=CYLINDRICAL_SURFACE ( 'NONE', #86579, 1.500000000000001332 ) ;
#196218=VERTEX_POINT ( 'NONE', #8460 ) ;
#196221=CARTESIAN_POINT ( 'NONE',  ( 5.035744501201078851E-13, -76.33743099897125717, -22.99988689144064580 ) ) ;
#196237=VERTEX_POINT ( 'NONE', #177328 ) ;
#196246=CARTESIAN_POINT ( 'NONE',  ( 21.00373069265142689, 22.92260996908688142, -50.16862556671883056 ) ) ;
#196267=CARTESIAN_POINT ( 'NONE',  ( 24.24789025133660303, -29.25582059975608118, -16.65643465479911711 ) ) ;
#196285=DIRECTION ( 'NONE',  ( -1.000000000000000000, 0.000000000000000000, 0.000000000000000000 ) ) ;
#196289=CARTESIAN_POINT ( 'NONE',  ( -6.673977169394459175, 4.619345608252460877, -64.16796455867367399 ) ) ;
#196300=EDGE_LOOP ( 'NONE', ( #151453, #138560, #196685, #168116 ) ) ;
#196325=DIRECTION ( 'NONE',  ( 1.000000000000000000, 0.000000000000000000, 0.000000000000000000 ) ) ;
#196326=ORIENTED_EDGE ( 'NONE', *, *, #155138, .F. ) ;
#196359=VERTEX_POINT ( 'NONE', #97441 ) ;
#196364=CARTESIAN_POINT ( 'NONE',  ( -38.00000000000000711, 2.428612866367529932E-14, -10.00000000000000000 ) ) ;
#196444=ORIENTED_EDGE ( 'NONE', *, *, #84390, .T. ) ;
#196446=ADVANCED_FACE ( 'NONE', ( #38799 ), #162136, .F. ) ;
#196490=FACE_OUTER_BOUND ( 'NONE', #167083, .T. ) ;
#196503=VERTEX_POINT ( 'NONE', #189495 ) ;
#196506=CARTESIAN_POINT ( 'NONE',  ( -11.74264578624800670, 36.14014761921585972, -8.400000000000000355 ) ) ;
#196511=CARTESIAN_POINT ( 'NONE',  ( 1.212108430020047534, 16.08886519554586414, -59.40479301947630120 ) ) ;
#196558=ORIENTED_EDGE ( 'NONE', *, *, #87165, .T. ) ;
#196562=CARTESIAN_POINT ( 'NONE',  ( -22.81625015709509441, -31.40387420917324590, -8.324999997268815122 ) ) ;
#196595=CYLINDRICAL_SURFACE ( 'NONE', #175423, 4.000000000000000888 ) ;
#196600=DIRECTION ( 'NONE',  ( 0.000000000000000000, 0.000000000000000000, -1.000000000000000000 ) ) ;
#196611=B_SPLINE_CURVE_WITH_KNOTS ( 'NONE', 3,
 ( #29470, #14283, #184140, #75951, #137625, #30452 ),
 .UNSPECIFIED., .F., .F.,
 ( 4, 2, 4 ),
 ( 0.004725762209527889501, 0.005384798814614493584, 0.006043835419701097667 ),
 .UNSPECIFIED. ) ;
#196625=ORIENTED_EDGE ( 'NONE', *, *, #110504, .F. ) ;
#196685=ORIENTED_EDGE ( 'NONE', *, *, #176309, .F. ) ;
#196713=CARTESIAN_POINT ( 'NONE',  ( -14.53388260107741736, -39.78846373132474667, -19.96647037889510656 ) ) ;
#196723=LINE ( 'NONE', #121827, #37037 ) ;
#196738=CARTESIAN_POINT ( 'NONE',  ( -22.81625015709509441, -31.40387420917324590, -8.324999997268813345 ) ) ;
#196744=ORIENTED_EDGE ( 'NONE', *, *, #160152, .T. ) ;
#196755=CARTESIAN_POINT ( 'NONE',  ( 10.05780954200632493, -38.14163830725774318, -31.65208490131638541 ) ) ;
#196832=ADVANCED_FACE ( 'NONE', ( #72130 ), #166146, .F. ) ;
#196867=VERTEX_POINT ( 'NONE', #56970 ) ;
#196878=EDGE_CURVE ( 'NONE', #5010, #176889, #117464, .T. ) ;
#196939=CARTESIAN_POINT ( 'NONE',  ( 10.78896075761529261, -9.218258452770006883, -62.39945043303440997 ) ) ;
#196940=CARTESIAN_POINT ( 'NONE',  ( 1.220435812286612354, 14.30591040068875408, -60.18371924376236137 ) ) ;
#196952=CARTESIAN_POINT ( 'NONE',  ( -11.30153831258471975, -180.0000000000000000, -15.00000000000000178 ) ) ;
#196968=ORIENTED_EDGE ( 'NONE', *, *, #73495, .T. ) ;
#196971=CARTESIAN_POINT ( 'NONE',  ( 4.999999999999996447, 37.66961640367475184, -15.00000000000000000 ) ) ;
#196975=CARTESIAN_POINT ( 'NONE',  ( -23.48529157249599919, -32.32473071737750558, -5.449999994537626513 ) ) ;
#196989=CARTESIAN_POINT ( 'NONE',  ( -11.80868324581538253, 11.80868324581533457, -59.13370768023891344 ) ) ;
#197001=CARTESIAN_POINT ( 'NONE',  ( -23.16108095314128690, 1.467328942211057585, -57.58004187413776265 ) ) ;
#197014=DIRECTION ( 'NONE',  ( -0.000000000000000000, -0.000000000000000000, 1.000000000000000000 ) ) ;
#197017=CARTESIAN_POINT ( 'NONE',  ( -15.06137443927361019, -15.06137443927335440, -58.85720012050613548 ) ) ;
#197027=CARTESIAN_POINT ( 'NONE',  ( -5.950531402560715689E-15, 38.81732327939063509, -7.624999997268814056 ) ) ;
#197028=CARTESIAN_POINT ( 'NONE',  ( -0.8193109935766856866, -21.52594032250406642, -58.70475745007095014 ) ) ;
#197048=CARTESIAN_POINT ( 'NONE',  ( -20.09009762002150978, -36.41118502144959024, -19.08443133123632762 ) ) ;
#197049=VERTEX_POINT ( 'NONE', #133804 ) ;
#197063=CARTESIAN_POINT ( 'NONE',  ( -1.425084765988079205, -7.121805330552575697, -64.33521149768087355 ) ) ;
#197115=CARTESIAN_POINT ( 'NONE',  ( 4.000000000000000888, -165.0000000000000000, 12.00000000000000355 ) ) ;
#197151=VECTOR ( 'NONE', #176962, 1000.000000000000000 ) ;
#197159=DIRECTION ( 'NONE',  ( 0.000000000000000000, 0.000000000000000000, -1.000000000000000000 ) ) ;
#197176=CARTESIAN_POINT ( 'NONE',  ( -6.795175062723227022, 4.884302457959417865, -62.06722337258344879 ) ) ;
#197180=CARTESIAN_POINT ( 'NONE',  ( 0.6293029420441302868, 31.76613490820970398, -45.84550579068238818 ) ) ;
#197183=CARTESIAN_POINT ( 'NONE',  ( 0.000000000000000000, 0.000000000000000000, -49.13275782002545355 ) ) ;
#197184=EDGE_CURVE ( 'NONE', #75168, #150285, #91239, .T. ) ;
#197214=EDGE_CURVE ( 'NONE', #25387, #133509, #78474, .T. ) ;
#197245=CARTESIAN_POINT ( 'NONE',  ( 28.47622644277404191, -25.16156846422445881, -16.68312038616162241 ) ) ;
#197268=CARTESIAN_POINT ( 'NONE',  ( -6.576150211591581751, 6.293193206003589779, -63.95112321872120731 ) ) ;
#197319=ADVANCED_FACE ( 'NONE', ( #64902 ), #171093, .F. ) ;
#197338=DIRECTION ( 'NONE',  ( -0.000000000000000000, 0.000000000000000000, 1.000000000000000000 ) ) ;
#197342=CARTESIAN_POINT ( 'NONE',  ( 0.000000000000000000, -105.0000000000000000, 12.00000000000000355 ) ) ;
#197373=CARTESIAN_POINT ( 'NONE',  ( -30.74264578624800492, -22.33583958711396278, -3.549999994537626602 ) ) ;
#197461=DIRECTION ( 'NONE',  ( -0.000000000000000000, -0.000000000000000000, 1.000000000000000000 ) ) ;
#197463=CARTESIAN_POINT ( 'NONE',  ( 17.46008511430124344, -15.43033707490625162, -57.51273177586173091 ) ) ;
#197476=CARTESIAN_POINT ( 'NONE',  ( -3.573655867282028392E-15, 2.428612866367529932E-14, -15.00000000000000000 ) ) ;
#197484=CARTESIAN_POINT ( 'NONE',  ( -38.00000000000001421, -12.34694845685042708, -5.900000000000000355 ) ) ;
#197513=VERTEX_POINT ( 'NONE', #127561 ) ;
#197529=EDGE_CURVE ( 'NONE', #73471, #21583, #159435, .T. ) ;
#197536=VERTEX_POINT ( 'NONE', #159898 ) ;
#197557=EDGE_CURVE ( 'NONE', #107603, #45261, #8674, .T. ) ;
#197575=DIRECTION ( 'NONE',  ( -0.000000000000000000, -0.000000000000000000, 1.000000000000000000 ) ) ;
#197599=CARTESIAN_POINT ( 'NONE',  ( 1.500000000002908562, 30.39999999999990266, -50.95361246531977173 ) ) ;
#197617=DIRECTION ( 'NONE',  ( 1.000000000000000000, 0.000000000000000000, 0.000000000000000000 ) ) ;
#197660=ORIENTED_EDGE ( 'NONE', *, *, #100613, .F. ) ;
#197688=CARTESIAN_POINT ( 'NONE',  ( -21.25171708481316912, -32.43382446246058493, -17.33145006470357075 ) ) ;
#197713=CARTESIAN_POINT ( 'NONE',  ( -11.40812507854754720, -35.11059874428192273, -8.224999997268813701 ) ) ;
#197719=ORIENTED_EDGE ( 'NONE', *, *, #117749, .T. ) ;
#197812=B_SPLINE_CURVE_WITH_KNOTS ( 'NONE', 3,
 ( #94939, #39245, #7898, #25100, #85744, #196939, #118095, #116087, #99906, #69583, #10919, #119099, #179785, #103918, #23085, #26094 ),
 .UNSPECIFIED., .F., .F.,
 ( 4, 2, 2, 2, 2, 2, 2, 4 ),
 ( 2.787258272608875357E-07, 0.0004619591141080896354, 0.0009236395023889183058, 0.001847000278950579116, 0.002308680667231405130, 0.002770361055512230927, 0.003232041443793056291, 0.003693721832073882522 ),
 .UNSPECIFIED. ) ;
#197900=FACE_OUTER_BOUND ( 'NONE', #147518, .T. ) ;
#197947=VERTEX_POINT ( 'NONE', #157914 ) ;
#197952=FACE_OUTER_BOUND ( 'NONE', #21694, .T. ) ;
#197956=CARTESIAN_POINT ( 'NONE',  ( -11.40812507854755609, 35.11059874428196537, -1.524999997268813301 ) ) ;
#198010=CARTESIAN_POINT ( 'NONE',  ( 0.1984113195539776442, 9.090086778104248921, -63.95305758601499235 ) ) ;
#198014=AXIS2_PLACEMENT_3D ( 'NONE', #108912, #170592, #93739 ) ;
#198016=CARTESIAN_POINT ( 'NONE',  ( 30.43137438583966059, -22.75957854975411010, -19.69424960774841082 ) ) ;
#198029=CARTESIAN_POINT ( 'NONE',  ( -32.63354670694344151, -22.83594557639104750, -20.39123836177964222 ) ) ;
#198040=EDGE_LOOP ( 'NONE', ( #59883, #137944, #36601, #188996 ) ) ;
#198044=DIRECTION ( 'NONE',  ( 1.000000000000000000, 3.552713678800500929E-15, 0.000000000000000000 ) ) ;
#198056=CARTESIAN_POINT ( 'NONE',  ( 7.990187535671190666, -1.461319442807313740, -64.16708268805474802 ) ) ;
#198078=ORIENTED_EDGE ( 'NONE', *, *, #36572, .T. ) ;
#198117=DIRECTION ( 'NONE',  ( -0.000000000000000000, -0.000000000000000000, 1.000000000000000000 ) ) ;
#198160=CARTESIAN_POINT ( 'NONE',  ( -20.97218796591018020, 20.08580022215221206, -49.51012018364362888 ) ) ;
#198190=EDGE_CURVE ( 'NONE', #181556, #127301, #169113, .T. ) ;
#198205=DIRECTION ( 'NONE',  ( 0.000000000000000000, 0.000000000000000000, 1.000000000000000000 ) ) ;
#198225=CARTESIAN_POINT ( 'NONE',  ( 15.49673173449294694, -38.75597260389996990, -19.54956558032594316 ) ) ;
#198260=EDGE_LOOP ( 'NONE', ( #76299, #182785, #79107, #16377 ) ) ;
#198353=CARTESIAN_POINT ( 'NONE',  ( -6.404328268737242702, 0.9271017399332003306, -64.47359807031669732 ) ) ;
#198402=ORIENTED_EDGE ( 'NONE', *, *, #19810, .F. ) ;
#198406=ORIENTED_EDGE ( 'NONE', *, *, #4868, .T. ) ;
#198420=CIRCLE ( 'NONE', #137074, 69.99999999999998579 ) ;
#198446=CARTESIAN_POINT ( 'NONE',  ( 15.18083716703543651, -14.94191171151153341, -58.85720012050614969 ) ) ;
#198452=CARTESIAN_POINT ( 'NONE',  ( -16.12203461105344005, -16.12203461105316649, -64.92279855667830191 ) ) ;
#198454=CARTESIAN_POINT ( 'NONE',  ( -40.00000000000000711, 2.918471586026471156E-14, -25.00000000000000000 ) ) ;
#198469=CARTESIAN_POINT ( 'NONE',  ( 23.48529157249600630, -32.32473071737749137, -5.300000000000000711 ) ) ;
#198496=CARTESIAN_POINT ( 'NONE',  ( -12.73749492396214578, -155.7167183371837496, -15.00000000000000178 ) ) ;
#198523=EDGE_LOOP ( 'NONE', ( #177888, #22581, #54692, #79453, #103001 ) ) ;
#198557=CIRCLE ( 'NONE', #163046, 21.30000000000002913 ) ;
#198579=VECTOR ( 'NONE', #174824, 1000.000000000000000 ) ;
#198589=CARTESIAN_POINT ( 'NONE',  ( 1.363652971230786992, 31.04735526335058537, -50.18466865107295405 ) ) ;
#198615=CIRCLE ( 'NONE', #111407, 38.00000000000000000 ) ;
#198616=CARTESIAN_POINT ( 'NONE',  ( 15.19344129729077331, 17.31327599691201868, -55.22348155082431731 ) ) ;
#198618=CYLINDRICAL_SURFACE ( 'NONE', #111126, 28.90000000000004476 ) ;
#198654=ORIENTED_EDGE ( 'NONE', *, *, #115666, .T. ) ;
#198657=VERTEX_POINT ( 'NONE', #30357 ) ;
#198666=CARTESIAN_POINT ( 'NONE',  ( -10.75775780536858051, -37.01749054245972559, -23.73535027650243023 ) ) ;
#198705=CARTESIAN_POINT ( 'NONE',  ( 3.556970738554034288E-15, -38.81732327939057114, -10.12499999726881228 ) ) ;
#198744=VERTEX_POINT ( 'NONE', #96974 ) ;
#198885=ORIENTED_EDGE ( 'NONE', *, *, #29329, .T. ) ;
#198894=AXIS2_PLACEMENT_3D ( 'NONE', #98936, #87772, #145448 ) ;
#198913=CARTESIAN_POINT ( 'NONE',  ( 0.9479838643943441223, 14.02093834921316429, -60.30661765432581944 ) ) ;
#198927=CARTESIAN_POINT ( 'NONE',  ( 17.62203461105334767, -16.12203461105336189, -54.55577602037946150 ) ) ;
#198930=CARTESIAN_POINT ( 'NONE',  ( -1.022580077288041090E-15, -16.70000000000002061, -59.13370768023891344 ) ) ;
#198937=CARTESIAN_POINT ( 'NONE',  ( -21.71908475311230546, -22.98719380919931510, -46.06929478400958544 ) ) ;
#198946=ORIENTED_EDGE ( 'NONE', *, *, #147318, .F. ) ;
#198952=CARTESIAN_POINT ( 'NONE',  ( 30.74264578624799782, 22.33583958711400541, -10.54999999453762705 ) ) ;
#198964=CARTESIAN_POINT ( 'NONE',  ( 4.242540618128931129, 4.384162112346963625, -62.50719930893271226 ) ) ;
#198999=CARTESIAN_POINT ( 'NONE',  ( 3.556970738554034288E-15, -38.81732327939057114, -10.62499999726880873 ) ) ;
#199001=CARTESIAN_POINT ( 'NONE',  ( 0.000000000000000000, 0.000000000000000000, -64.92279855667830191 ) ) ;
#199044=CARTESIAN_POINT ( 'NONE',  ( 8.349412516403786455, -1.313804288003802112, -64.09731636040743297 ) ) ;
#199123=EDGE_CURVE ( 'NONE', #59792, #47952, #32647, .T. ) ;
#199145=CARTESIAN_POINT ( 'NONE',  ( -6.719756334737514436, 4.704316316549534527, -62.10423353180174644 ) ) ;
#199149=CARTESIAN_POINT ( 'NONE',  ( 0.5056555311937657171, 28.98228079209996366, -49.57211623589792282 ) ) ;
#199168=CARTESIAN_POINT ( 'NONE',  ( -4.570733098192837459E-16, -74.04324336000735229, -22.99263613531268291 ) ) ;
#199187=CIRCLE ( 'NONE', #189508, 28.90000000000004476 ) ;
#199216=CARTESIAN_POINT ( 'NONE',  ( -6.206754193738958314, -6.630370177702000767, -63.95556908907604310 ) ) ;
#199217=AXIS2_PLACEMENT_3D ( 'NONE', #101025, #23209, #69702 ) ;
#199242=CARTESIAN_POINT ( 'NONE',  ( -6.795352961392306490, 4.884805615686619973, -64.11485260110077888 ) ) ;
#199248=CARTESIAN_POINT ( 'NONE',  ( -26.36902008128208408, -29.90370362120039616, -17.00062383490520901 ) ) ;
#199276=B_SPLINE_CURVE_WITH_KNOTS ( 'NONE', 3,
 ( #171648, #139310, #188816, #64467, #154488, #156475, #124134, #92800, #187829, #79630, #15982, #32144, #789, #172641, #141298, #78627, #62461, #50299, #107969, #46314, #169656, #185833 ),
 .UNSPECIFIED., .F., .F.,
 ( 4, 2, 2, 2, 2, 2, 2, 2, 2, 2, 4 ),
 ( 2.787258305036405189E-07, 0.0003055402697144848283, 0.0006108018135984659511, 0.001221324901366425053, 0.001831847989134390009, 0.002137109533018372379, 0.002442371076902354748, 0.003052894164670319488, 0.003663417252438284661, 0.004273940340206248967, 0.004884463427974213706 ),
 .UNSPECIFIED. ) ;
#199293=ADVANCED_FACE ( 'NONE', ( #164668 ), #27162, .F. ) ;
#199320=CARTESIAN_POINT ( 'NONE',  ( 4.647474457565486646E-15, -28.90000000000004476, -64.92279855667830191 ) ) ;
#199362=VECTOR ( 'NONE', #34290, 1000.000000000000000 ) ;
#199407=CARTESIAN_POINT ( 'NONE',  ( -11.74264578624800670, 36.14014761921585972, -8.149999994537626691 ) ) ;
#199438=CARTESIAN_POINT ( 'NONE',  ( -11.45643923738959735, 5.000000000000007105, -18.00000000000000000 ) ) ;
#199440=CARTESIAN_POINT ( 'NONE',  ( 14.82524568295233891, -1.464953661134022367, -59.95866808466630005 ) ) ;
#199452=CIRCLE ( 'NONE', #73619, 7.999999999999998224 ) ;
#199458=EDGE_CURVE ( 'NONE', #74853, #171133, #42324, .T. ) ;
#199461=CARTESIAN_POINT ( 'NONE',  ( -23.48529157249599919, -32.32473071737750558, -5.700000000000000178 ) ) ;
#199487=CARTESIAN_POINT ( 'NONE',  ( 12.38288446667197995, -41.98357824127743498, -20.85955585120671074 ) ) ;
#199554=EDGE_CURVE ( 'NONE', #110784, #89826, #39312, .T. ) ;
#199575=CARTESIAN_POINT ( 'NONE',  ( 1.280994563191180546, 31.20196472458911785, -49.99722732359649058 ) ) ;
#199595=FACE_OUTER_BOUND ( 'NONE', #25973, .T. ) ;
#199603=CARTESIAN_POINT ( 'NONE',  ( -22.24618122112613960, -22.80753876826822690, -49.18602036547672185 ) ) ;
#199637=AXIS2_PLACEMENT_3D ( 'NONE', #135790, #197461, #71118 ) ;
#199640=EDGE_LOOP ( 'NONE', ( #115007, #47043, #20579, #43271 ) ) ;
#199653=CARTESIAN_POINT ( 'NONE',  ( -15.59283147534494063, -34.52683219101068346, -28.07673947521500324 ) ) ;
#199659=ORIENTED_EDGE ( 'NONE', *, *, #194281, .T. ) ;
#199686=CARTESIAN_POINT ( 'NONE',  ( 8.388830574159379737E-16, 13.70000000000001528, -60.44446360152740283 ) ) ;
#199696=CARTESIAN_POINT ( 'NONE',  ( 22.81625015709509441, 31.40387420917330275, -9.324999997268813345 ) ) ;
#199707=DIRECTION ( 'NONE',  ( 1.000000000000000000, 0.000000000000000000, 0.000000000000000000 ) ) ;
#199754=ORIENTED_EDGE ( 'NONE', *, *, #125272, .T. ) ;
#199791=CARTESIAN_POINT ( 'NONE',  ( 1.322848289251850051, 15.93242547297147738, -61.66673749439198104 ) ) ;
#199820=FACE_OUTER_BOUND ( 'NONE', #121027, .T. ) ;
#199927=FACE_BOUND ( 'NONE', #10749, .T. ) ;
#199933=CARTESIAN_POINT ( 'NONE',  ( -22.39645207350164924, -22.70003318984301188, -45.66685071139480812 ) ) ;
#199948=CARTESIAN_POINT ( 'NONE',  ( -36.91746825000001309, -11.99521256947794789, -5.024999997268813523 ) ) ;
#199960=CARTESIAN_POINT ( 'NONE',  ( 12.06208868505712672, -11.49801227349071731, -59.15175176635164433 ) ) ;
#200029=CIRCLE ( 'NONE', #158005, 61.99999999999998579 ) ;
#200059=EDGE_CURVE ( 'NONE', #99831, #17478, #5234, .T. ) ;
#200135=DIRECTION ( 'NONE',  ( -1.000000000000000000, 6.391086490440865492E-16, 0.000000000000000000 ) ) ;
#200139=CARTESIAN_POINT ( 'NONE',  ( -22.99905646750782751, 21.51934928555102289, -46.25979504214461713 ) ) ;
#200173=EDGE_LOOP ( 'NONE', ( #163171, #30976 ) ) ;
#200177=CARTESIAN_POINT ( 'NONE',  ( -6.941592873960384935, 1.351304681146122233, -62.33628431810819137 ) ) ;
#200187=CARTESIAN_POINT ( 'NONE',  ( 23.88070017481517837, -1.044764468832730664, -57.07230391339720654 ) ) ;
ENDSEC;
END-ISO-10303-21;
